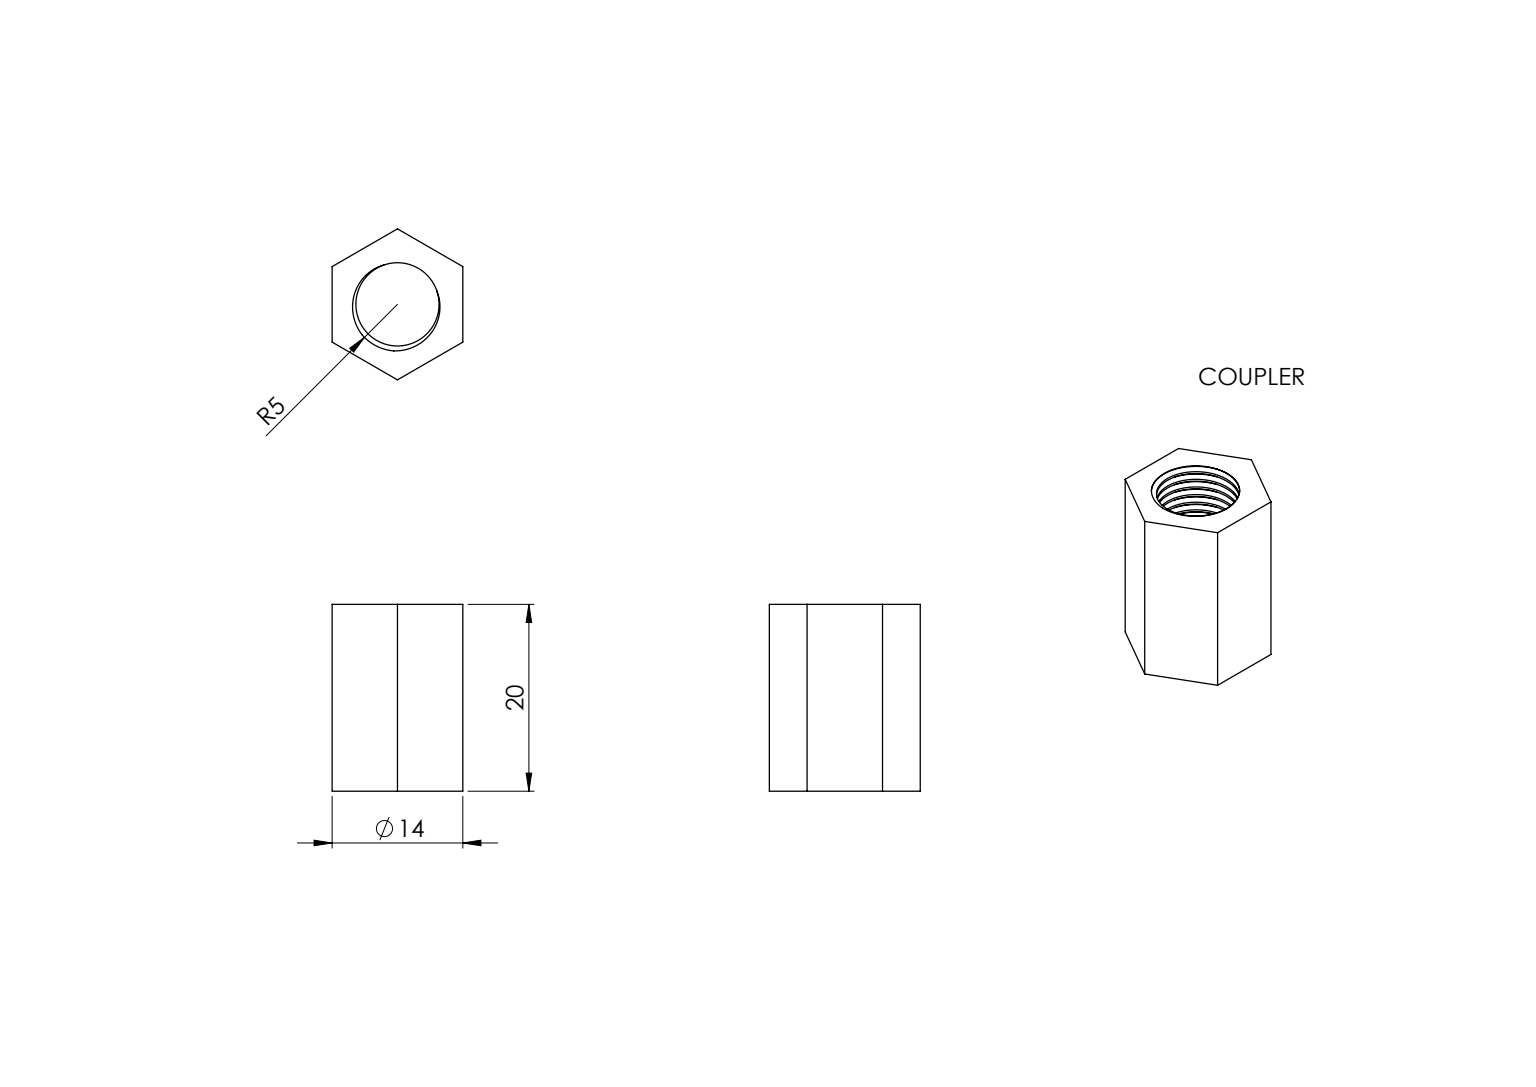
ISO-10303-21;
HEADER;
FILE_DESCRIPTION (('STEP AP214'),
    '1' );
FILE_NAME ('coupler.step',
    '2026-10-25T05:52:03',
    ( '' ),
    ( '' ),
    'SwSTEP 2.0',
    'SolidWorks 2026',
    '' );
FILE_SCHEMA (( 'AUTOMOTIVE_DESIGN' ));
ENDSEC;

DATA;
#3=CARTESIAN_POINT ( 'NONE',  ( -59.29741812935640155, -128.8750000013656063, -2.196230717870135685 ) ) ;
#16=CARTESIAN_POINT ( 'NONE',  ( -60.14911071818854538, -150.1875000027311842, 1.666127454062681368 ) ) ;
#81=CARTESIAN_POINT ( 'NONE',  ( -50.70258187064364108, -139.3750000013656063, 2.196230717870141014 ) ) ;
#85=ORIENTED_EDGE ( 'NONE', *, *, #22562, .F. ) ;
#86=ADVANCED_FACE ( 'NONE', ( #1332 ), #40849, .F. ) ;
#94=CARTESIAN_POINT ( 'NONE',  ( -54.60164318462004474, -140.3750000000000284, -4.984105922594373794 ) ) ;
#101=ADVANCED_FACE ( 'NONE', ( #35084 ), #10624, .T. ) ;
#104=ADVANCED_FACE ( 'NONE', ( #49860 ), #20614, .F. ) ;
#106=CARTESIAN_POINT ( 'NONE',  ( -58.39396692619412477, -139.4375000013656063, 2.891590998281057701 ) ) ;
#132=CARTESIAN_POINT ( 'NONE',  ( -51.60603307380591787, -145.1875000013656063, -2.891590998281053704 ) ) ;
#163=ORIENTED_EDGE ( 'NONE', *, *, #35025, .F. ) ;
#169=CARTESIAN_POINT ( 'NONE',  ( -50.18089887299979068, -133.6875000000000568, 2.462841084822635640 ) ) ;
#178=CARTESIAN_POINT ( 'NONE',  ( -60.14911071818854538, -125.1875000027312126, 1.666127454062681368 ) ) ;
#202=CARTESIAN_POINT ( 'NONE',  ( -53.51423613279429503, -126.2500000013656063, 4.591703134518082763 ) ) ;
#203=CARTESIAN_POINT ( 'NONE',  ( -52.10840900171896806, -147.1875000013656063, 3.393966926194110556 ) ) ;
#214=CARTESIAN_POINT ( 'NONE',  ( -55.35523342533222291, -125.5625000013655921, 4.444560631937231499 ) ) ;
#235=CARTESIAN_POINT ( 'NONE',  ( -59.44456063193725015, -149.8125000013656063, -0.3552334253322034230 ) ) ;
#246=CARTESIAN_POINT ( 'NONE',  ( -53.33387254593733928, -145.8125000000000284, 5.149110718188519620 ) ) ;
#253=ORIENTED_EDGE ( 'NONE', *, *, #51599, .T. ) ;
#254=CARTESIAN_POINT ( 'NONE',  ( -59.29741812935640155, -144.8750000013656063, -2.196230717870135685 ) ) ;
#255=CARTESIAN_POINT ( 'NONE',  ( -49.85088928181150436, -137.6875000027312126, -1.666127454062680702 ) ) ;
#267=CARTESIAN_POINT ( 'NONE',  ( -49.85088928181150436, -153.5625000000000284, -1.666127454062680480 ) ) ;
#268=CARTESIAN_POINT ( 'NONE',  ( -50.40829686548195099, -135.0000000013656347, -1.485763867205728284 ) ) ;
#283=CARTESIAN_POINT ( 'NONE',  ( -59.59170313451811296, -138.5000000013656347, 1.485763867205729394 ) ) ;
#314=CARTESIAN_POINT ( 'NONE',  ( -56.48576386720575471, -152.7500000013655779, -4.591703134518078322 ) ) ;
#321=CARTESIAN_POINT ( 'NONE',  ( -57.19623071787017210, -127.6250000013656205, 4.297418129356382899 ) ) ;
#331=CARTESIAN_POINT ( 'NONE',  ( -51.19402409849444524, -149.6250000027312126, -3.242614290531456334 ) ) ;
#360=CARTESIAN_POINT ( 'NONE',  ( -55.00000000000002132, -155.0000000000000284, 1.734723475976807094E-15 ) ) ;
#374=CARTESIAN_POINT ( 'NONE',  ( -59.77950423082105402, -135.0000000000000284, -0.4113032182319603658 ) ) ;
#389=EDGE_CURVE ( 'NONE', #14198, #16286, #4716, .T. ) ;
#399=CARTESIAN_POINT ( 'NONE',  ( -51.60603307380591787, -141.1875000013656063, -2.891590998281053704 ) ) ;
#402=EDGE_LOOP ( 'NONE', ( #47162, #48030, #33761, #57243 ) ) ;
#404=ORIENTED_EDGE ( 'NONE', *, *, #32775, .T. ) ;
#408=CYLINDRICAL_SURFACE ( 'NONE', #17648, 5.000000000000000000 ) ;
#418=CARTESIAN_POINT ( 'NONE',  ( -52.10840900171896806, -139.1875000013656347, 3.393966926194110556 ) ) ;
#441=CARTESIAN_POINT ( 'NONE',  ( -52.10840900171896806, -143.4375000013656063, 3.393966926194110556 ) ) ;
#470=CARTESIAN_POINT ( 'NONE',  ( -60.14911071818854538, -151.0625000000000284, 1.666127454062681146 ) ) ;
#485=CARTESIAN_POINT ( 'NONE',  ( -49.85088928181150436, -130.5625000000000568, -1.666127454062680702 ) ) ;
#491=ORIENTED_EDGE ( 'NONE', *, *, #46738, .F. ) ;
#493=CARTESIAN_POINT ( 'NONE',  ( -51.60603307380591787, -152.9375000013656063, -2.891590998281053704 ) ) ;
#515=CIRCLE ( 'NONE', #57003, 5.000000000000000000 ) ;
#516=CARTESIAN_POINT ( 'NONE',  ( -50.70258187064364108, -154.3750000013656063, 2.196230717870141014 ) ) ;
#517=CARTESIAN_POINT ( 'NONE',  ( -54.64476657466781973, -145.8125000013656063, -4.444560631937228834 ) ) ;
#518=EDGE_CURVE ( 'NONE', #43968, #24595, #43685, .T. ) ;
#542=EDGE_CURVE ( 'NONE', #41301, #34010, #1942, .T. ) ;
#546=DIRECTION ( 'NONE',  ( 0.000000000000000000, -1.000000000000000000, 0.000000000000000000 ) ) ;
#552=CARTESIAN_POINT ( 'NONE',  ( -52.10840900171896806, -146.4375000013656063, 3.393966926194110556 ) ) ;
#562=CARTESIAN_POINT ( 'NONE',  ( -52.53715891517739323, -147.4375000000000284, -4.819101127000233298 ) ) ;
#571=CARTESIAN_POINT ( 'NONE',  ( -59.59170313451810586, -144.7500000013655779, 1.485763867205729394 ) ) ;
#573=CARTESIAN_POINT ( 'NONE',  ( -51.75738570946856498, -134.8750000027312126, 3.805975901505576964 ) ) ;
#585=CARTESIAN_POINT ( 'NONE',  ( -52.80376928212989185, -132.8750000013656063, -4.297418129356379346 ) ) ;
#600=CARTESIAN_POINT ( 'NONE',  ( -59.44456063193725015, -138.5625000013656063, -0.3552334253322034230 ) ) ;
#610=CARTESIAN_POINT ( 'NONE',  ( -55.35523342533222291, -133.5625000013656063, 4.444560631937231499 ) ) ;
#633=CARTESIAN_POINT ( 'NONE',  ( -59.44456063193725015, -151.5625000013656063, -0.3552334253322034230 ) ) ;
#641=CARTESIAN_POINT ( 'NONE',  ( -52.80376928212989185, -129.1250000013655779, -4.297418129356379346 ) ) ;
#644=CARTESIAN_POINT ( 'NONE',  ( -50.01589407740564042, -136.7500000027312126, 0.3983568153799778022 ) ) ;
#651=CARTESIAN_POINT ( 'NONE',  ( -50.01589407740564042, -150.7500000027312410, 0.3983568153799778022 ) ) ;
#655=ORIENTED_EDGE ( 'NONE', *, *, #11941, .T. ) ;
#656=AXIS2_PLACEMENT_3D ( 'NONE', #10891, #51098, #35667 ) ;
#672=CARTESIAN_POINT ( 'NONE',  ( -54.64476657466781973, -150.8125000013656063, -4.444560631937228834 ) ) ;
#674=CARTESIAN_POINT ( 'NONE',  ( -50.01589407740564042, -148.6250000000000284, 0.3983568153799778022 ) ) ;
#697=VECTOR ( 'NONE', #14487, 1000.000000000000114 ) ;
#717=CARTESIAN_POINT ( 'NONE',  ( -55.35523342533222291, -139.5625000013656063, 4.444560631937231499 ) ) ;
#728=CARTESIAN_POINT ( 'NONE',  ( -52.53715891517739323, -140.4375000000000000, -4.819101127000233298 ) ) ;
#738=CARTESIAN_POINT ( 'NONE',  ( -50.40829686548195099, -141.0000000013656063, -1.485763867205728284 ) ) ;
#764=CARTESIAN_POINT ( 'NONE',  ( -49.85088928181150436, -154.5625000000000000, -1.666127454062680480 ) ) ;
#768=CARTESIAN_POINT ( 'NONE',  ( -55.35523342533222291, -143.5625000013656063, 4.444560631937231499 ) ) ;
#769=CARTESIAN_POINT ( 'NONE',  ( -55.00000000000002132, -155.0000000000000284, 1.734723475976807094E-15 ) ) ;
#774=CARTESIAN_POINT ( 'NONE',  ( -58.24261429053147765, -136.2500000000000284, -3.805975901505573855 ) ) ;
#782=CARTESIAN_POINT ( 'NONE',  ( -54.60164318462004474, -138.5000000027312126, -4.984105922594373794 ) ) ;
#804=CARTESIAN_POINT ( 'NONE',  ( -56.66612745406293783, -141.3125000000000000, -5.149110718188535607 ) ) ;
#809=CARTESIAN_POINT ( 'NONE',  ( -58.80597590150559739, -130.0000000000000284, 3.242614290531460330 ) ) ;
#819=CARTESIAN_POINT ( 'NONE',  ( -57.19623071787017210, -154.3750000013656063, 4.297418129356382899 ) ) ;
#822=DIRECTION ( 'NONE',  ( 0.000000000000000000, -1.000000000000000000, 0.000000000000000000 ) ) ;
#848=CARTESIAN_POINT ( 'NONE',  ( -56.48576386720575471, -124.7500000013655921, -4.591703134518078322 ) ) ;
#849=CARTESIAN_POINT ( 'NONE',  ( -55.35523342533222291, -142.3125000013656063, 4.444560631937231499 ) ) ;
#877=ORIENTED_EDGE ( 'NONE', *, *, #37498, .T. ) ;
#888=CARTESIAN_POINT ( 'NONE',  ( -51.75738570946856498, -139.7500000000000000, 3.805975901505576964 ) ) ;
#898=CARTESIAN_POINT ( 'NONE',  ( -59.59170313451810586, -146.7500000013656063, 1.485763867205729394 ) ) ;
#900=CARTESIAN_POINT ( 'NONE',  ( -60.14911071818854538, -134.1875000027312410, 1.666127454062681368 ) ) ;
#916=CARTESIAN_POINT ( 'NONE',  ( -52.80376928212989185, -128.8750000013656063, -4.297418129356379346 ) ) ;
#933=( BOUNDED_CURVE ( )  B_SPLINE_CURVE ( 2, ( #61186, #36731, #45181, #61505, #52157, #37669, #30381, #11955, #12285 ),
 .UNSPECIFIED., .F., .F. ) 
 B_SPLINE_CURVE_WITH_KNOTS ( ( 3, 2, 2, 2, 3 ),
 ( 0.2250000000000001998, 0.2291666666666668517, 0.2333333333333335313, 0.2375000000000001832, 0.2416666666666668628 ),
 .UNSPECIFIED. ) 
 CURVE ( )  GEOMETRIC_REPRESENTATION_ITEM ( )  RATIONAL_B_SPLINE_CURVE ( ( 0.9999999999999964473, 0.9238795325112902912, 1.000000000000000000, 0.9238795325112867385, 1.000000000000000000, 0.9238795325112867385, 1.000000000000000000, 0.9238795325112831858, 1.000000000000003553 ) ) 
 REPRESENTATION_ITEM ( '' )  );
#934=CARTESIAN_POINT ( 'NONE',  ( -52.80376928212989185, -138.8750000013655779, -4.297418129356379346 ) ) ;
#945=CARTESIAN_POINT ( 'NONE',  ( -52.80376928212989185, -130.1250000013656347, -4.297418129356379346 ) ) ;
#970=CARTESIAN_POINT ( 'NONE',  ( -59.59170313451810586, -151.5000000013655779, 1.485763867205729394 ) ) ;
#977=CARTESIAN_POINT ( 'NONE',  ( -50.01589407740564042, -154.6250000000000284, 0.3983568153799778022 ) ) ;
#988=CARTESIAN_POINT ( 'NONE',  ( -50.18089887299979068, -145.8125000027311842, 2.462841084822635640 ) ) ;
#1004=CARTESIAN_POINT ( 'NONE',  ( -56.66612745406288099, -143.3125000000000000, -5.149110718188529390 ) ) ;
#1006=CARTESIAN_POINT ( 'NONE',  ( -57.89159099828107458, -149.6875000013656063, -3.393966926194107447 ) ) ;
#1025=CARTESIAN_POINT ( 'NONE',  ( -51.75738570946856498, -140.7500000000000000, 3.805975901505576964 ) ) ;
#1037=CARTESIAN_POINT ( 'NONE',  ( -51.19402409849444524, -147.6250000027312126, -3.242614290531456334 ) ) ;
#1052=CARTESIAN_POINT ( 'NONE',  ( -51.60603307380591787, -134.1875000013656063, -2.891590998281053704 ) ) ;
#1058=CARTESIAN_POINT ( 'NONE',  ( -55.00000000000002132, -155.0000000000000284, 1.734723475976807094E-15 ) ) ;
#1068=CARTESIAN_POINT ( 'NONE',  ( -53.51423613279429503, -140.2500000013656063, 4.591703134518082763 ) ) ;
#1073=ORIENTED_EDGE ( 'NONE', *, *, #41605, .F. ) ;
#1090=CARTESIAN_POINT ( 'NONE',  ( -56.66612745406272467, -154.3125000000000284, -5.149110718188517843 ) ) ;
#1093=CARTESIAN_POINT ( 'NONE',  ( -50.55543936806279248, -145.3125000013656063, 0.3552334253322060320 ) ) ;
#1138=CARTESIAN_POINT ( 'NONE',  ( -50.01589407740564042, -128.6250000000000284, 0.3983568153799778022 ) ) ;
#1145=CARTESIAN_POINT ( 'NONE',  ( -52.53715891517739323, -124.5625000027312268, -4.819101127000233298 ) ) ;
#1167=VECTOR ( 'NONE', #55223, 1000.000000000000000 ) ;
#1170=CARTESIAN_POINT ( 'NONE',  ( -55.35523342533222291, -126.3125000013655921, 4.444560631937231499 ) ) ;
#1171=CARTESIAN_POINT ( 'NONE',  ( -55.35523342533222291, -141.3125000013656063, 4.444560631937231499 ) ) ;
#1213=CARTESIAN_POINT ( 'NONE',  ( -58.24261429053147765, -140.2500000000000000, -3.805975901505573855 ) ) ;
#1216=ORIENTED_EDGE ( 'NONE', *, *, #46137, .T. ) ;
#1223=CARTESIAN_POINT ( 'NONE',  ( -57.89159099828107458, -144.9375000013656063, -3.393966926194107447 ) ) ;
#1225=CARTESIAN_POINT ( 'NONE',  ( -53.33387254593733928, -132.9375000027312126, 5.149110718188519620 ) ) ;
#1237=CARTESIAN_POINT ( 'NONE',  ( -50.40829686548195099, -129.0000000013656063, -1.485763867205728284 ) ) ;
#1251=CARTESIAN_POINT ( 'NONE',  ( -53.51423613279429503, -138.2500000013656063, 4.591703134518082763 ) ) ;
#1260=CARTESIAN_POINT ( 'NONE',  ( -58.39396692619412477, -133.6875000013656063, 2.891590998281057701 ) ) ;
#1289=CARTESIAN_POINT ( 'NONE',  ( -54.64476657466781973, -149.8125000013656063, -4.444560631937228834 ) ) ;
#1296=EDGE_CURVE ( 'NONE', #19989, #11458, #56971, .T. ) ;
#1299=CARTESIAN_POINT ( 'NONE',  ( -58.24261429053147765, -154.2500000000000284, -3.805975901505573855 ) ) ;
#1309=CARTESIAN_POINT ( 'NONE',  ( -56.66612745406270335, -145.4375000027312694, -5.149110718188516067 ) ) ;
#1325=CARTESIAN_POINT ( 'NONE',  ( -51.60603307380591787, -148.9375000013656063, -2.891590998281053704 ) ) ;
#1332=FACE_OUTER_BOUND ( 'NONE', #402, .T. ) ;
#1364=CARTESIAN_POINT ( 'NONE',  ( -57.46284108482265651, -141.0625000027312410, 4.819101127000238627 ) ) ;
#1372=CARTESIAN_POINT ( 'NONE',  ( -59.59170313451811296, -135.7500000013656063, 1.485763867205729394 ) ) ;
#1388=CARTESIAN_POINT ( 'NONE',  ( -57.89159099828107458, -140.6875000013656063, -3.393966926194107447 ) ) ;
#1389=CARTESIAN_POINT ( 'NONE',  ( -51.75738570946856498, -154.7500000000000284, 3.805975901505576964 ) ) ;
#1413=CARTESIAN_POINT ( 'NONE',  ( -51.60603307380591787, -141.1875000013656063, -2.891590998281053704 ) ) ;
#1423=VERTEX_POINT ( 'NONE', #56144 ) ;
#1432=CARTESIAN_POINT ( 'NONE',  ( -58.24261429053147765, -151.3750000027312126, -3.805975901505573855 ) ) ;
#1444=AXIS2_PLACEMENT_3D ( 'NONE', #10621, #50516, #34419 ) ;
#1446=CARTESIAN_POINT ( 'NONE',  ( -54.60164318462004474, -137.3750000000000284, -4.984105922594373794 ) ) ;
#1453=CARTESIAN_POINT ( 'NONE',  ( -51.19402409849444524, -129.5000000000000284, -3.242614290531456334 ) ) ;
#1457=VECTOR ( 'NONE', #822, 1000.000000000000000 ) ;
#1461=CARTESIAN_POINT ( 'NONE',  ( -50.55543936806279248, -151.0625000013656063, 0.3552334253322060320 ) ) ;
#1467=EDGE_CURVE ( 'NONE', #46511, #2425, #9232, .T. ) ;
#1484=CARTESIAN_POINT ( 'NONE',  ( -59.29741812935640155, -127.6250000013656205, -2.196230717870135685 ) ) ;
#1485=CARTESIAN_POINT ( 'NONE',  ( -50.55543936806279248, -141.0625000013656063, 0.3552334253322060320 ) ) ;
#1488=CARTESIAN_POINT ( 'NONE',  ( -50.18089887299979068, -153.8125000027311842, 2.462841084822631199 ) ) ;
#1521=CARTESIAN_POINT ( 'NONE',  ( -55.39835681537999790, -141.8750000000000284, 4.984105922594378235 ) ) ;
#1530=CARTESIAN_POINT ( 'NONE',  ( -57.89159099828107458, -140.9375000013656063, -3.393966926194107447 ) ) ;
#1532=CARTESIAN_POINT ( 'NONE',  ( -50.01589407740564042, -133.7500000027312126, 0.3983568153799778022 ) ) ;
#1547=CARTESIAN_POINT ( 'NONE',  ( -55.35523342533222291, -128.3125000013656063, 4.444560631937231499 ) ) ;
#1562=CARTESIAN_POINT ( 'NONE',  ( -50.40829686548195099, -138.0000000013656063, -1.485763867205728284 ) ) ;
#1571=ORIENTED_EDGE ( 'NONE', *, *, #11677, .F. ) ;
#1573=CARTESIAN_POINT ( 'NONE',  ( -52.10840900171896806, -132.4375000013656063, 3.393966926194110556 ) ) ;
#1607=CARTESIAN_POINT ( 'NONE',  ( -56.48576386720575471, -125.0000000013656205, -4.591703134518078322 ) ) ;
#1617=CARTESIAN_POINT ( 'NONE',  ( -58.24261429053147765, -145.3750000027312126, -3.805975901505573855 ) ) ;
#1630=ORIENTED_EDGE ( 'NONE', *, *, #7870, .T. ) ;
#1637=CARTESIAN_POINT ( 'NONE',  ( -58.39396692619412477, -149.4375000013656063, 2.891590998281057701 ) ) ;
#1666=CARTESIAN_POINT ( 'NONE',  ( -50.01589407740564042, -147.7500000027312126, 0.3983568153799778022 ) ) ;
#1680=CARTESIAN_POINT ( 'NONE',  ( -57.19623071787017210, -133.6250000013655779, 4.297418129356382899 ) ) ;
#1688=CARTESIAN_POINT ( 'NONE',  ( -50.84841373685102184, -135.0000000000001137, -1.652645393539816210 ) ) ;
#1689=ORIENTED_EDGE ( 'NONE', *, *, #14237, .T. ) ;
#1717=AXIS2_PLACEMENT_3D ( 'NONE', #19426, #24252, #13966 ) ;
#1726=CARTESIAN_POINT ( 'NONE',  ( -50.40829686548195099, -141.2500000013656347, -1.485763867205728284 ) ) ;
#1728=EDGE_CURVE ( 'NONE', #35208, #29222, #34787, .T. ) ;
#1743=CARTESIAN_POINT ( 'NONE',  ( -50.18089887299976937, -138.8125000027312126, 2.462841084822397164 ) ) ;
#1748=CARTESIAN_POINT ( 'NONE',  ( -59.44456063193725015, -136.8125000013656063, -0.3552334253322034230 ) ) ;
#1760=CARTESIAN_POINT ( 'NONE',  ( -53.51423613279429503, -148.5000000013655779, 4.591703134518082763 ) ) ;
#1764=ORIENTED_EDGE ( 'NONE', *, *, #58262, .F. ) ;
#1772=CARTESIAN_POINT ( 'NONE',  ( -59.81910112700025905, -131.1875000000000568, -2.462841084822630311 ) ) ;
#1778=AXIS2_PLACEMENT_3D ( 'NONE', #35397, #61762, #7412 ) ;
#1781=CARTESIAN_POINT ( 'NONE',  ( -50.55543936806279248, -153.0625000013656063, 0.3552334253322060320 ) ) ;
#1782=CARTESIAN_POINT ( 'NONE',  ( -57.46284108482265651, -150.0625000027312126, 4.819101127000238627 ) ) ;
#1784=( BOUNDED_SURFACE ( )  B_SPLINE_SURFACE ( 1, 2, ( 
 ( #18999, #28654, #39246, #49226, #52797, #4527, #19635, #4227, #38932, #38612, #58248, #34108, #8733, #23841, #14174, #33800, #62771, #58873, #14803, #39563, #34417, #47958, #29595, #33489, #63399, #54046, #9983, #5167, #53418, #24785, #59204, #18691, #15132, #28341, #3913, #58567, #9351, #43131, #28963, #38317, #57945, #13865, #43444, #24152, #55013, #35392, #15775, #49544, #40843, #39883, #5484, #45996, #41159, #45039, #25745, #25420, #25099, #20923, #672, #10937, #60804, #16415, #55345, #35715, #50513, #45678, #26063, #36033, #11259, #54380, #6765, #30883, #55665, #6454, #11578, #1961, #1006, #34754, #20281, #30555, #1637, #21237, #50180, #6132, #60487, #31198, #44709, #50827, #1325, #40528, #26378, #45360, #35078, #54698, #21562, #10305, #29918, #59528, #60170, #20610, #30231, #15461, #16091, #10619, #49855, #5803, #40215, #59850, #11891, #21879, #61442, #22198, #12851, #31838, #32147, #7724, #27017, #46635, #2906, #55978, #17368, #51469, #16731, #36991, #32470, #37611, #42745, #36347, #42114, #41798, #22521, #27645, #52099, #12534, #51782, #2581, #27329, #46959, #61758, #17686, #52422, #8039, #31509, #37301, #17050, #56930, #56618, #47272, #3218, #22838, #42429, #51154, #62071, #26701, #2275, #36666, #7087, #41475, #27954, #17985, #57252, #13168, #8354, #46318, #32792, #47576, #3528, #23137, #61125, #56293, #12223, #7408, #14734, #53347, #43065, #43998, #24715, #53035, #43375, #62703, #33108, #18628, #18928, #19565, #8973, #62388, #9597, #19244, #52722, #29518, #38860, #58496, #9910, #9282, #14420, #38251, #57566, #63646, #34042, #53663, #63021, #8656, #48830, #18309, #28269, #28897, #24395, #29204, #24086, #13492, #4458, #4770, #13794, #14104, #48518, #28583, #48204, #43681, #37934, #38542, #33416, #47884, #58174, #39177, #58802, #3842, #23462, #63325, #23774, #34351, #53980, #49150, #33729, #5096, #4157, #57872, #15703, #35321, #50108, #16342, #35644, #59131, #30485, #44641, #6063, #20538, #25676, #5734, #25350, #934, #19882, #10868, #54298, #29843, #600, #283, #5414, #55590, #10549, #1251, #44970, #35964, #39495, #1562, #40135, #11509, #31125, #55270, #54942, #45285, #20852, #60417, #40456, #25031, #25988, #6692, #35009, #59777, #20210, #15066, #39812, #60096, #21164, #54624, #44319, #11188, #16017, #34679, #50748, #30811, #50441, #10238, #6382, #45605, #59454, #49476, #40771, #15385, #30159, #49788, #16654, #12772, #45921, #60732, #56540, #52019, #2823, #51708, #41086, #32071, #61364, #32394, #61679, #36279, #22442, #12460, #7649, #27562, #2504, #26622, #46241, #42039, #17612, #37228, #56854, #22122, #16974, #21807, #1884, #27252, #46879, #26297, #31433, #7963, #36585, #21488, #51073, #7336, #31761, #47195, #3138, #55903, #7014, #22757, #56220, #11814, #2203, #26947, #51394, #42355, #41402, #41714, #17286, #12140, #46564, #61994, #61053, #36909, #17914, #37535, #57175, #13092, #32712, #52340, #8274, #33653, #33338, #58093, #19158, #23999, #4077, #23700, #57795, #62933, #43297, #18847, #14024, #43915, #63245, #23064, #53271, #8579, #9206, #48126, #28819, #52955, #8893, #28508, #47497, #38467, #18231, #57490, #28191, #27878, #33030, #19483, #38173, #48440, #4380, #63563, #3450, #29122, #43601, #39096, #58725, #38777, #58416, #14343, #33964, #24309, #53585, #52646, #9515, #34270, #62629, #48745, #47806, #42669, #3763, #4687, #14651, #18551, #62308, #37857, #13409, #23387, #42986, #13715, #50027, #1484, #44887, #5985, #10153, #49065, #55186, #25590, #45203, #54543, #44238, #40375, #9821, #24631, #20450, #15939, #30404, #15625, #5011, #59694, #25266, #60016, #1170, #202, #20770, #40050, #35242, #11106, #30078, #54215, #29758, #35562, #30731, #50353, #6300, #49709, #44559, #49392, #29431, #10466, #25905, #19800, #45523, #5654, #21087, #40691, #60336, #848, #54861, #10792, #16264, #53896, #34583 ),
 ( #39408, #59047, #14975, #5336, #24953, #516, #20127, #39727, #59366, #15299, #34922, #36509, #26223, #22363, #55512, #6610, #2430, #61604, #12387, #61286, #50669, #41633, #7258, #41963, #7568, #45843, #32001, #22041, #17208, #37158, #12060, #36199, #55820, #51635, #27181, #46797, #2743, #31685, #26546, #31354, #11426, #36835, #56465, #35882, #41012, #17539, #46166, #31044, #60655, #16892, #41325, #56782, #50995, #51320, #26871, #2128, #21729, #12701, #1805, #56140, #6934, #21409, #46483, #32314, #51945, #61922, #16579, #7885, #60972, #27488, #47118, #3066, #22683, #42283, #11736, #8822, #52887, #28437, #23625, #53509, #9133, #32634, #4003, #18153, #43221, #57722, #37465, #32954, #62556, #52263, #23928, #22997, #8201, #29049, #24238, #28120, #48050, #8510, #27804, #9439, #28739, #62861, #18774, #38401, #33889, #58024, #62236, #63174, #43842, #47737, #18476, #37782, #47429, #57413, #38097, #38704, #3694, #17842, #48366, #13953, #3380, #48673, #33579, #53199, #4613, #4309, #43529, #13333, #13015, #19085, #58341, #14270, #13648, #42599, #57095, #52578, #23307, #42907, #33268, #39976, #25189, #14574, #5575, #34850, #5903, #35173, #9750, #59621, #30008, #49638, #1093, #39653, #132, #19726, #15553, #54789, #10719, #30326, #59290, #54136, #58968, #39026, #44805, #20375, #63488, #4937, #45129, #10075, #58654, #24560, #44482, #5260, #49950, #14896, #15221, #54471, #29687, #49317, #768, #34197, #441, #34504, #19412, #20048, #25510, #20702, #25833, #53821, #40306, #24881, #59944, #15867, #35488, #10398, #55107, #11029, #30653, #50276, #6221, #29357, #48990, #44164, #39335, #31609, #45769, #40931, #16814, #26788, #60579, #26471, #2046, #21013, #11981, #55432, #30971, #1726, #1413, #6536, #56704, #11660, #2356, #46086, #17462, #40620, #2664, #21652, #12622, #36434, #36122, #60264, #51244, #11349, #41244, #51866, #27104, #21964, #46407, #61210, #56388, #36759, #46719, #41559, #16182, #37084, #17136, #22285, #12315, #41884, #32235, #55744, #7809, #50596, #60891, #31927, #51555, #56064, #61530, #7491, #21331, #50914, #45449, #35807, #26150, #16500, #31280, #7180, #6857, #62478, #61849, #47664, #28354, #13880, #27411, #3616, #23855, #42205, #4240, #47356, #47974, #18076, #63103, #43458, #57650, #33508, #2991, #19015, #38628, #22927, #52181, #53435, #3928, #43146, #58270, #37385, #33815, #22609, #14190, #47042, #23223, #42836, #17768, #57338, #27729, #53124, #57019, #12934, #18398, #62786, #3305, #13578, #13254, #32878, #8749, #32558, #42519, #37697, #52506, #8126, #23546, #57959, #62156, #38330, #8440, #28044, #38019, #33196, #9058, #28668, #48285, #52811, #18705, #25999, #20219, #45617, #30822, #50453, #1260, #10879, #610, #15712, #11519, #1894, #36289, #30496, #21500, #28979, #25360, #54950, #24167, #16353, #15394, #43770, #41096, #16666, #20547, #6073, #1573, #10556, #40466, #40144, #35330, #55281, #48601, #5741, #59789, #50117, #39820, #6393, #40781, #60743, #21173, #4541, #50759, #54632, #20863, #60427, #35974, #55601, #25686, #31134, #6703, #59462, #26309, #45931, #9366, #60106, #45295, #35019, #16027, #30167, #49797, #44979, #35654, #945, #11200, #7345, #36921, #7024, #62004, #61064, #26633, #3461, #62319, #2515, #46890, #46574, #46253, #42048, #21816, #32081, #18244, #37545, #12782, #56864, #7974, #3149, #47206, #57185, #32404, #11824, #27888, #52031, #13104, #27572, #32722, #23074, #22131, #55912, #41413, #56550, #22769, #42365, #51718, #8284, #17923, #56231, #61374, #52350, #47510, #42678, #31443, #51086, #12471, #2213, #27264, #16984, #7659, #36596, #12152, #31771, #2833, #51403, #26956, #41725, #17295, #22451, #61691, #17622, #37239, #4391, #43928, #13418, #9833, #34283, #33351, #62641, #214, #14354, #53597, #29445, #47816, #44250, #33041, #53907, #49077, #33663, #53281, #5024, #4089, #38184, #24322 ) ),
 .UNSPECIFIED., .F., .F., .F. ) 
 B_SPLINE_SURFACE_WITH_KNOTS ( ( 2, 2 ),
 ( 3, 2, 2, 2, 2, 2, 2, 2, 2, 2, 2, 2, 2, 2, 2, 2, 2, 2, 2, 2, 2, 2, 2, 2, 2, 2, 2, 2, 2, 2, 2, 2, 2, 2, 2, 2, 2, 2, 2, 2, 2, 2, 2, 2, 2, 2, 2, 2, 2, 2, 2, 2, 2, 2, 2, 2, 2, 2, 2, 2, 2, 2, 2, 2, 2, 2, 2, 2, 2, 2, 2, 2, 2, 2, 2, 2, 2, 2, 2, 2, 2, 2, 2, 2, 2, 2, 2, 2, 2, 2, 2, 2, 2, 2, 2, 2, 2, 2, 2, 2, 2, 2, 2, 2, 2, 2, 2, 2, 2, 2, 2, 2, 2, 2, 2, 2, 2, 2, 2, 2, 2, 2, 2, 2, 2, 2, 2, 2, 2, 2, 2, 2, 2, 2, 2, 2, 2, 2, 2, 2, 2, 2, 2, 2, 2, 2, 2, 2, 2, 2, 2, 2, 2, 2, 2, 2, 2, 2, 2, 2, 2, 2, 2, 2, 2, 2, 2, 2, 2, 2, 2, 2, 2, 2, 2, 2, 2, 2, 2, 2, 2, 2, 2, 2, 2, 2, 2, 2, 2, 2, 2, 2, 2, 2, 2, 2, 2, 2, 2, 2, 2, 2, 2, 2, 2, 2, 2, 2, 2, 2, 2, 2, 2, 2, 2, 2, 2, 2, 2, 2, 2, 2, 2, 2, 2, 2, 2, 2, 2, 2, 2, 2, 2, 2, 2, 2, 2, 2, 2, 2, 3 ),
 ( 0.000000000000000000, 1.000000000000000000 ),
 ( 0.000000000000000000, 0.004166666666666666609, 0.008333333333333333218, 0.01250000000000000069, 0.01666666666666666644, 0.02083333333333333218, 0.02500000000000000139, 0.02916666666666666713, 0.03333333333333333287, 0.03749999999999999861, 0.04166666666666666435, 0.04583333333333333010, 0.05000000000000000278, 0.05416666666666666852, 0.05833333333333333426, 0.06250000000000000000, 0.06666666666666666574, 0.07083333333333333148, 0.07499999999999999722, 0.07916666666666666297, 0.08333333333333332871, 0.08749999999999999445, 0.09166666666666666019, 0.09583333333333333981, 0.1000000000000000056, 0.1041666666666666713, 0.1083333333333333370, 0.1125000000000000028, 0.1166666666666666685, 0.1208333333333333343, 0.1250000000000000000, 0.1291666666666666796, 0.1333333333333333315, 0.1375000000000000111, 0.1416666666666666630, 0.1458333333333333426, 0.1499999999999999944, 0.1541666666666666741, 0.1583333333333333259, 0.1625000000000000056, 0.1666666666666666574, 0.1708333333333333370, 0.1749999999999999889, 0.1791666666666666685, 0.1833333333333333204, 0.1875000000000000000, 0.1916666666666666796, 0.1958333333333333315, 0.2000000000000000111, 0.2041666666666666630, 0.2083333333333333426, 0.2124999999999999944, 0.2166666666666666741, 0.2208333333333333259, 0.2250000000000000056, 0.2291666666666666574, 0.2333333333333333370, 0.2374999999999999889, 0.2416666666666666685, 0.2458333333333333204, 0.2500000000000000000, 0.2541666666666666519, 0.2583333333333333592, 0.2625000000000000111, 0.2666666666666666630, 0.2708333333333333148, 0.2750000000000000222, 0.2791666666666666741, 0.2833333333333333259, 0.2874999999999999778, 0.2916666666666666852, 0.2958333333333333370, 0.2999999999999999889, 0.3041666666666666408, 0.3083333333333333481, 0.3125000000000000000, 0.3166666666666666519, 0.3208333333333333592, 0.3250000000000000111, 0.3291666666666666630, 0.3333333333333333148, 0.3375000000000000222, 0.3416666666666666741, 0.3458333333333333259, 0.3499999999999999778, 0.3541666666666666852, 0.3583333333333333370, 0.3624999999999999889, 0.3666666666666666408, 0.3708333333333333481, 0.3750000000000000000, 0.3791666666666666519, 0.3833333333333333592, 0.3875000000000000111, 0.3916666666666666630, 0.3958333333333333148, 0.4000000000000000222, 0.4041666666666666741, 0.4083333333333333259, 0.4124999999999999778, 0.4166666666666666852, 0.4208333333333333370, 0.4249999999999999889, 0.4291666666666666408, 0.4333333333333333481, 0.4375000000000000000, 0.4416666666666666519, 0.4458333333333333592, 0.4500000000000000111, 0.4541666666666666630, 0.4583333333333333148, 0.4625000000000000222, 0.4666666666666666741, 0.4708333333333333259, 0.4749999999999999778, 0.4791666666666666852, 0.4833333333333333370, 0.4874999999999999889, 0.4916666666666666408, 0.4958333333333333481, 0.5000000000000000000, 0.5041666666666666519, 0.5083333333333333037, 0.5124999999999999556, 0.5166666666666667185, 0.5208333333333333703, 0.5250000000000000222, 0.5291666666666666741, 0.5333333333333333259, 0.5374999999999999778, 0.5416666666666666297, 0.5458333333333332815, 0.5500000000000000444, 0.5541666666666666963, 0.5583333333333333481, 0.5625000000000000000, 0.5666666666666666519, 0.5708333333333333037, 0.5749999999999999556, 0.5791666666666667185, 0.5833333333333333703, 0.5875000000000000222, 0.5916666666666666741, 0.5958333333333333259, 0.5999999999999999778, 0.6041666666666666297, 0.6083333333333332815, 0.6125000000000000444, 0.6166666666666666963, 0.6208333333333333481, 0.6250000000000000000, 0.6291666666666666519, 0.6333333333333333037, 0.6374999999999999556, 0.6416666666666667185, 0.6458333333333333703, 0.6500000000000000222, 0.6541666666666666741, 0.6583333333333333259, 0.6624999999999999778, 0.6666666666666666297, 0.6708333333333332815, 0.6750000000000000444, 0.6791666666666666963, 0.6833333333333333481, 0.6875000000000000000, 0.6916666666666666519, 0.6958333333333333037, 0.6999999999999999556, 0.7041666666666667185, 0.7083333333333333703, 0.7125000000000000222, 0.7166666666666666741, 0.7208333333333333259, 0.7249999999999999778, 0.7291666666666666297, 0.7333333333333332815, 0.7375000000000000444, 0.7416666666666666963, 0.7458333333333333481, 0.7500000000000000000, 0.7541666666666666519, 0.7583333333333333037, 0.7624999999999999556, 0.7666666666666667185, 0.7708333333333333703, 0.7750000000000000222, 0.7791666666666666741, 0.7833333333333333259, 0.7874999999999999778, 0.7916666666666666297, 0.7958333333333332815, 0.8000000000000000444, 0.8041666666666666963, 0.8083333333333333481, 0.8125000000000000000, 0.8166666666666666519, 0.8208333333333333037, 0.8249999999999999556, 0.8291666666666667185, 0.8333333333333333703, 0.8375000000000000222, 0.8416666666666666741, 0.8458333333333333259, 0.8499999999999999778, 0.8541666666666666297, 0.8583333333333332815, 0.8625000000000000444, 0.8666666666666666963, 0.8708333333333333481, 0.8750000000000000000, 0.8791666666666666519, 0.8833333333333333037, 0.8874999999999999556, 0.8916666666666667185, 0.8958333333333333703, 0.9000000000000000222, 0.9041666666666666741, 0.9083333333333333259, 0.9124999999999999778, 0.9166666666666666297, 0.9208333333333332815, 0.9250000000000000444, 0.9291666666666666963, 0.9333333333333333481, 0.9375000000000000000, 0.9416666666666666519, 0.9458333333333333037, 0.9499999999999999556, 0.9541666666666667185, 0.9583333333333333703, 0.9625000000000000222, 0.9666666666666666741, 0.9708333333333333259, 0.9749999999999999778, 0.9791666666666666297, 0.9833333333333332815, 0.9875000000000000444, 0.9916666666666666963, 0.9958333333333333481, 1.000000000000000000 ),
 .UNSPECIFIED. ) 
 GEOMETRIC_REPRESENTATION_ITEM ( )  RATIONAL_B_SPLINE_SURFACE ( (
 ( 1.000000000000000000, 0.9238795325112867385, 1.000000000000000000, 0.9238795325112867385, 1.000000000000000000, 0.9238795325112867385, 1.000000000000000000, 0.9238795325112867385, 1.000000000000000000, 0.9238795325112867385, 1.000000000000000000, 0.9238795325112867385, 1.000000000000000000, 0.9238795325112867385, 1.000000000000000000, 0.9238795325112867385, 1.000000000000000000, 0.9238795325112867385, 1.000000000000000000, 0.9238795325112867385, 1.000000000000000000, 0.9238795325112867385, 1.000000000000000000, 0.9238795325112867385, 1.000000000000000000, 0.9238795325112867385, 1.000000000000000000, 0.9238795325112867385, 1.000000000000000000, 0.9238795325112867385, 1.000000000000000000, 0.9238795325112867385, 1.000000000000000000, 0.9238795325112867385, 1.000000000000000000, 0.9238795325112867385, 1.000000000000000000, 0.9238795325112867385, 1.000000000000000000, 0.9238795325112867385, 1.000000000000000000, 0.9238795325112867385, 1.000000000000000000, 0.9238795325112867385, 1.000000000000000000, 0.9238795325112867385, 1.000000000000000000, 0.9238795325112867385, 1.000000000000000000, 0.9238795325112867385, 1.000000000000000000, 0.9238795325112867385, 1.000000000000000000, 0.9238795325112867385, 1.000000000000000000, 0.9238795325112867385, 1.000000000000000000, 0.9238795325112867385, 1.000000000000000000, 0.9238795325112867385, 1.000000000000000000, 0.9238795325112867385, 1.000000000000000000, 0.9238795325112867385, 1.000000000000000000, 0.9238795325112867385, 1.000000000000000000, 0.9238795325112867385, 1.000000000000000000, 0.9238795325112867385, 1.000000000000000000, 0.9238795325112867385, 1.000000000000000000, 0.9238795325112867385, 1.000000000000000000, 0.9238795325112867385, 1.000000000000000000, 0.9238795325112867385, 1.000000000000000000, 0.9238795325112867385, 1.000000000000000000, 0.9238795325112867385, 1.000000000000000000, 0.9238795325112867385, 1.000000000000000000, 0.9238795325112867385, 1.000000000000000000, 0.9238795325112867385, 1.000000000000000000, 0.9238795325112867385, 1.000000000000000000, 0.9238795325112867385, 1.000000000000000000, 0.9238795325112867385, 1.000000000000000000, 0.9238795325112867385, 1.000000000000000000, 0.9238795325112867385, 1.000000000000000000, 0.9238795325112867385, 1.000000000000000000, 0.9238795325112867385, 1.000000000000000000, 0.9238795325112867385, 1.000000000000000000, 0.9238795325112867385, 1.000000000000000000, 0.9238795325112867385, 1.000000000000000000, 0.9238795325112867385, 1.000000000000000000, 0.9238795325112867385, 1.000000000000000000, 0.9238795325112867385, 1.000000000000000000, 0.9238795325112867385, 1.000000000000000000, 0.9238795325112867385, 1.000000000000000000, 0.9238795325112867385, 1.000000000000000000, 0.9238795325112867385, 1.000000000000000000, 0.9238795325112867385, 1.000000000000000000, 0.9238795325112867385, 1.000000000000000000, 0.9238795325112867385, 1.000000000000000000, 0.9238795325112867385, 1.000000000000000000, 0.9238795325112867385, 1.000000000000000000, 0.9238795325112867385, 1.000000000000000000, 0.9238795325112867385, 1.000000000000000000, 0.9238795325112867385, 1.000000000000000000, 0.9238795325112867385, 1.000000000000000000, 0.9238795325112867385, 1.000000000000000000, 0.9238795325112867385, 1.000000000000000000, 0.9238795325112867385, 1.000000000000000000, 0.9238795325112867385, 1.000000000000000000, 0.9238795325112867385, 1.000000000000000000, 0.9238795325112867385, 1.000000000000000000, 0.9238795325112867385, 1.000000000000000000, 0.9238795325112867385, 1.000000000000000000, 0.9238795325112867385, 1.000000000000000000, 0.9238795325112867385, 1.000000000000000000, 0.9238795325112867385, 1.000000000000000000, 0.9238795325112867385, 1.000000000000000000, 0.9238795325112867385, 1.000000000000000000, 0.9238795325112867385, 1.000000000000000000, 0.9238795325112867385, 1.000000000000000000, 0.9238795325112867385, 1.000000000000000000, 0.9238795325112867385, 1.000000000000000000, 0.9238795325112867385, 1.000000000000000000, 0.9238795325112867385, 1.000000000000000000, 0.9238795325112867385, 1.000000000000000000, 0.9238795325112867385, 1.000000000000000000, 0.9238795325112867385, 1.000000000000000000, 0.9238795325112867385, 1.000000000000000000, 0.9238795325112867385, 1.000000000000000000, 0.9238795325112867385, 1.000000000000000000, 0.9238795325112867385, 1.000000000000000000, 0.9238795325112867385, 1.000000000000000000, 0.9238795325112867385, 1.000000000000000000, 0.9238795325112867385, 1.000000000000000000, 0.9238795325112867385, 1.000000000000000000, 0.9238795325112867385, 1.000000000000000000, 0.9238795325112867385, 1.000000000000000000, 0.9238795325112867385, 1.000000000000000000, 0.9238795325112867385, 1.000000000000000000, 0.9238795325112867385, 1.000000000000000000, 0.9238795325112867385, 1.000000000000000000, 0.9238795325112867385, 1.000000000000000000, 0.9238795325112867385, 1.000000000000000000, 0.9238795325112867385, 1.000000000000000000, 0.9238795325112867385, 1.000000000000000000, 0.9238795325112867385, 1.000000000000000000, 0.9238795325112867385, 1.000000000000000000, 0.9238795325112867385, 1.000000000000000000, 0.9238795325112867385, 1.000000000000000000, 0.9238795325112867385, 1.000000000000000000, 0.9238795325112867385, 1.000000000000000000, 0.9238795325112867385, 1.000000000000000000, 0.9238795325112867385, 1.000000000000000000, 0.9238795325112867385, 1.000000000000000000, 0.9238795325112867385, 1.000000000000000000, 0.9238795325112867385, 1.000000000000000000, 0.9238795325112867385, 1.000000000000000000, 0.9238795325112867385, 1.000000000000000000, 0.9238795325112867385, 1.000000000000000000, 0.9238795325112867385, 1.000000000000000000, 0.9238795325112867385, 1.000000000000000000, 0.9238795325112867385, 1.000000000000000000, 0.9238795325112867385, 1.000000000000000000, 0.9238795325112867385, 1.000000000000000000, 0.9238795325112867385, 1.000000000000000000, 0.9238795325112867385, 1.000000000000000000, 0.9238795325112867385, 1.000000000000000000, 0.9238795325112867385, 1.000000000000000000, 0.9238795325112867385, 1.000000000000000000, 0.9238795325112867385, 1.000000000000000000, 0.9238795325112867385, 1.000000000000000000, 0.9238795325112867385, 1.000000000000000000, 0.9238795325112867385, 1.000000000000000000, 0.9238795325112867385, 1.000000000000000000, 0.9238795325112867385, 1.000000000000000000, 0.9238795325112867385, 1.000000000000000000, 0.9238795325112867385, 1.000000000000000000, 0.9238795325112867385, 1.000000000000000000, 0.9238795325112867385, 1.000000000000000000, 0.9238795325112867385, 1.000000000000000000, 0.9238795325112867385, 1.000000000000000000, 0.9238795325112867385, 1.000000000000000000, 0.9238795325112867385, 1.000000000000000000, 0.9238795325112867385, 1.000000000000000000, 0.9238795325112867385, 1.000000000000000000, 0.9238795325112867385, 1.000000000000000000, 0.9238795325112867385, 1.000000000000000000, 0.9238795325112867385, 1.000000000000000000, 0.9238795325112867385, 1.000000000000000000, 0.9238795325112867385, 1.000000000000000000, 0.9238795325112867385, 1.000000000000000000, 0.9238795325112867385, 1.000000000000000000, 0.9238795325112867385, 1.000000000000000000, 0.9238795325112867385, 1.000000000000000000, 0.9238795325112867385, 1.000000000000000000, 0.9238795325112867385, 1.000000000000000000, 0.9238795325112867385, 1.000000000000000000, 0.9238795325112867385, 1.000000000000000000, 0.9238795325112867385, 1.000000000000000000, 0.9238795325112867385, 1.000000000000000000, 0.9238795325112867385, 1.000000000000000000, 0.9238795325112867385, 1.000000000000000000, 0.9238795325112867385, 1.000000000000000000, 0.9238795325112867385, 1.000000000000000000, 0.9238795325112867385, 1.000000000000000000, 0.9238795325112867385, 1.000000000000000000, 0.9238795325112867385, 1.000000000000000000, 0.9238795325112867385, 1.000000000000000000, 0.9238795325112867385, 1.000000000000000000, 0.9238795325112867385, 1.000000000000000000, 0.9238795325112867385, 1.000000000000000000, 0.9238795325112867385, 1.000000000000000000, 0.9238795325112867385, 1.000000000000000000, 0.9238795325112867385, 1.000000000000000000, 0.9238795325112867385, 1.000000000000000000, 0.9238795325112867385, 1.000000000000000000, 0.9238795325112867385, 1.000000000000000000, 0.9238795325112867385, 1.000000000000000000, 0.9238795325112867385, 1.000000000000000000, 0.9238795325112867385, 1.000000000000000000, 0.9238795325112867385, 1.000000000000000000, 0.9238795325112867385, 1.000000000000000000, 0.9238795325112867385, 1.000000000000000000, 0.9238795325112867385, 1.000000000000000000, 0.9238795325112867385, 1.000000000000000000, 0.9238795325112867385, 1.000000000000000000, 0.9238795325112867385, 1.000000000000000000, 0.9238795325112867385, 1.000000000000000000, 0.9238795325112867385, 1.000000000000000000, 0.9238795325112867385, 1.000000000000000000, 0.9238795325112867385, 1.000000000000000000, 0.9238795325112867385, 1.000000000000000000, 0.9238795325112867385, 1.000000000000000000, 0.9238795325112867385, 1.000000000000000000, 0.9238795325112867385, 1.000000000000000000, 0.9238795325112867385, 1.000000000000000000, 0.9238795325112867385, 1.000000000000000000, 0.9238795325112867385, 1.000000000000000000, 0.9238795325112867385, 1.000000000000000000, 0.9238795325112867385, 1.000000000000000000, 0.9238795325112867385, 1.000000000000000000, 0.9238795325112867385, 1.000000000000000000, 0.9238795325112867385, 1.000000000000000000, 0.9238795325112867385, 1.000000000000000000, 0.9238795325112867385, 1.000000000000000000, 0.9238795325112867385, 1.000000000000000000, 0.9238795325112867385, 1.000000000000000000, 0.9238795325112867385, 1.000000000000000000, 0.9238795325112867385, 1.000000000000000000, 0.9238795325112867385, 1.000000000000000000, 0.9238795325112867385, 1.000000000000000000, 0.9238795325112867385, 1.000000000000000000, 0.9238795325112867385, 1.000000000000000000, 0.9238795325112867385, 1.000000000000000000, 0.9238795325112867385, 1.000000000000000000, 0.9238795325112867385, 1.000000000000000000, 0.9238795325112867385, 1.000000000000000000, 0.9238795325112867385, 1.000000000000000000, 0.9238795325112867385, 1.000000000000000000, 0.9238795325112867385, 1.000000000000000000, 0.9238795325112867385, 1.000000000000000000, 0.9238795325112867385, 1.000000000000000000, 0.9238795325112867385, 1.000000000000000000, 0.9238795325112867385, 1.000000000000000000, 0.9238795325112867385, 1.000000000000000000, 0.9238795325112867385, 1.000000000000000000, 0.9238795325112867385, 1.000000000000000000, 0.9238795325112867385, 1.000000000000000000, 0.9238795325112867385, 1.000000000000000000, 0.9238795325112867385, 1.000000000000000000, 0.9238795325112867385, 1.000000000000000000, 0.9238795325112867385, 1.000000000000000000, 0.9238795325112867385, 1.000000000000000000, 0.9238795325112867385, 1.000000000000000000, 0.9238795325112867385, 1.000000000000000000),
 ( 1.000000000000000000, 0.9238795325112867385, 1.000000000000000000, 0.9238795325112867385, 1.000000000000000000, 0.9238795325112867385, 1.000000000000000000, 0.9238795325112867385, 1.000000000000000000, 0.9238795325112867385, 1.000000000000000000, 0.9238795325112867385, 1.000000000000000000, 0.9238795325112867385, 1.000000000000000000, 0.9238795325112867385, 1.000000000000000000, 0.9238795325112867385, 1.000000000000000000, 0.9238795325112867385, 1.000000000000000000, 0.9238795325112867385, 1.000000000000000000, 0.9238795325112867385, 1.000000000000000000, 0.9238795325112867385, 1.000000000000000000, 0.9238795325112867385, 1.000000000000000000, 0.9238795325112867385, 1.000000000000000000, 0.9238795325112867385, 1.000000000000000000, 0.9238795325112867385, 1.000000000000000000, 0.9238795325112867385, 1.000000000000000000, 0.9238795325112867385, 1.000000000000000000, 0.9238795325112867385, 1.000000000000000000, 0.9238795325112867385, 1.000000000000000000, 0.9238795325112867385, 1.000000000000000000, 0.9238795325112867385, 1.000000000000000000, 0.9238795325112867385, 1.000000000000000000, 0.9238795325112867385, 1.000000000000000000, 0.9238795325112867385, 1.000000000000000000, 0.9238795325112867385, 1.000000000000000000, 0.9238795325112867385, 1.000000000000000000, 0.9238795325112867385, 1.000000000000000000, 0.9238795325112867385, 1.000000000000000000, 0.9238795325112867385, 1.000000000000000000, 0.9238795325112867385, 1.000000000000000000, 0.9238795325112867385, 1.000000000000000000, 0.9238795325112867385, 1.000000000000000000, 0.9238795325112867385, 1.000000000000000000, 0.9238795325112867385, 1.000000000000000000, 0.9238795325112867385, 1.000000000000000000, 0.9238795325112867385, 1.000000000000000000, 0.9238795325112867385, 1.000000000000000000, 0.9238795325112867385, 1.000000000000000000, 0.9238795325112867385, 1.000000000000000000, 0.9238795325112867385, 1.000000000000000000, 0.9238795325112867385, 1.000000000000000000, 0.9238795325112867385, 1.000000000000000000, 0.9238795325112867385, 1.000000000000000000, 0.9238795325112867385, 1.000000000000000000, 0.9238795325112867385, 1.000000000000000000, 0.9238795325112867385, 1.000000000000000000, 0.9238795325112867385, 1.000000000000000000, 0.9238795325112867385, 1.000000000000000000, 0.9238795325112867385, 1.000000000000000000, 0.9238795325112867385, 1.000000000000000000, 0.9238795325112867385, 1.000000000000000000, 0.9238795325112867385, 1.000000000000000000, 0.9238795325112867385, 1.000000000000000000, 0.9238795325112867385, 1.000000000000000000, 0.9238795325112867385, 1.000000000000000000, 0.9238795325112867385, 1.000000000000000000, 0.9238795325112867385, 1.000000000000000000, 0.9238795325112867385, 1.000000000000000000, 0.9238795325112867385, 1.000000000000000000, 0.9238795325112867385, 1.000000000000000000, 0.9238795325112867385, 1.000000000000000000, 0.9238795325112867385, 1.000000000000000000, 0.9238795325112867385, 1.000000000000000000, 0.9238795325112867385, 1.000000000000000000, 0.9238795325112867385, 1.000000000000000000, 0.9238795325112867385, 1.000000000000000000, 0.9238795325112867385, 1.000000000000000000, 0.9238795325112867385, 1.000000000000000000, 0.9238795325112867385, 1.000000000000000000, 0.9238795325112867385, 1.000000000000000000, 0.9238795325112867385, 1.000000000000000000, 0.9238795325112867385, 1.000000000000000000, 0.9238795325112867385, 1.000000000000000000, 0.9238795325112867385, 1.000000000000000000, 0.9238795325112867385, 1.000000000000000000, 0.9238795325112867385, 1.000000000000000000, 0.9238795325112867385, 1.000000000000000000, 0.9238795325112867385, 1.000000000000000000, 0.9238795325112867385, 1.000000000000000000, 0.9238795325112867385, 1.000000000000000000, 0.9238795325112867385, 1.000000000000000000, 0.9238795325112867385, 1.000000000000000000, 0.9238795325112867385, 1.000000000000000000, 0.9238795325112867385, 1.000000000000000000, 0.9238795325112867385, 1.000000000000000000, 0.9238795325112867385, 1.000000000000000000, 0.9238795325112867385, 1.000000000000000000, 0.9238795325112867385, 1.000000000000000000, 0.9238795325112867385, 1.000000000000000000, 0.9238795325112867385, 1.000000000000000000, 0.9238795325112867385, 1.000000000000000000, 0.9238795325112867385, 1.000000000000000000, 0.9238795325112867385, 1.000000000000000000, 0.9238795325112867385, 1.000000000000000000, 0.9238795325112867385, 1.000000000000000000, 0.9238795325112867385, 1.000000000000000000, 0.9238795325112867385, 1.000000000000000000, 0.9238795325112867385, 1.000000000000000000, 0.9238795325112867385, 1.000000000000000000, 0.9238795325112867385, 1.000000000000000000, 0.9238795325112867385, 1.000000000000000000, 0.9238795325112867385, 1.000000000000000000, 0.9238795325112867385, 1.000000000000000000, 0.9238795325112867385, 1.000000000000000000, 0.9238795325112867385, 1.000000000000000000, 0.9238795325112867385, 1.000000000000000000, 0.9238795325112867385, 1.000000000000000000, 0.9238795325112867385, 1.000000000000000000, 0.9238795325112867385, 1.000000000000000000, 0.9238795325112867385, 1.000000000000000000, 0.9238795325112867385, 1.000000000000000000, 0.9238795325112867385, 1.000000000000000000, 0.9238795325112867385, 1.000000000000000000, 0.9238795325112867385, 1.000000000000000000, 0.9238795325112867385, 1.000000000000000000, 0.9238795325112867385, 1.000000000000000000, 0.9238795325112867385, 1.000000000000000000, 0.9238795325112867385, 1.000000000000000000, 0.9238795325112867385, 1.000000000000000000, 0.9238795325112867385, 1.000000000000000000, 0.9238795325112867385, 1.000000000000000000, 0.9238795325112867385, 1.000000000000000000, 0.9238795325112867385, 1.000000000000000000, 0.9238795325112867385, 1.000000000000000000, 0.9238795325112867385, 1.000000000000000000, 0.9238795325112867385, 1.000000000000000000, 0.9238795325112867385, 1.000000000000000000, 0.9238795325112867385, 1.000000000000000000, 0.9238795325112867385, 1.000000000000000000, 0.9238795325112867385, 1.000000000000000000, 0.9238795325112867385, 1.000000000000000000, 0.9238795325112867385, 1.000000000000000000, 0.9238795325112867385, 1.000000000000000000, 0.9238795325112867385, 1.000000000000000000, 0.9238795325112867385, 1.000000000000000000, 0.9238795325112867385, 1.000000000000000000, 0.9238795325112867385, 1.000000000000000000, 0.9238795325112867385, 1.000000000000000000, 0.9238795325112867385, 1.000000000000000000, 0.9238795325112867385, 1.000000000000000000, 0.9238795325112867385, 1.000000000000000000, 0.9238795325112867385, 1.000000000000000000, 0.9238795325112867385, 1.000000000000000000, 0.9238795325112867385, 1.000000000000000000, 0.9238795325112867385, 1.000000000000000000, 0.9238795325112867385, 1.000000000000000000, 0.9238795325112867385, 1.000000000000000000, 0.9238795325112867385, 1.000000000000000000, 0.9238795325112867385, 1.000000000000000000, 0.9238795325112867385, 1.000000000000000000, 0.9238795325112867385, 1.000000000000000000, 0.9238795325112867385, 1.000000000000000000, 0.9238795325112867385, 1.000000000000000000, 0.9238795325112867385, 1.000000000000000000, 0.9238795325112867385, 1.000000000000000000, 0.9238795325112867385, 1.000000000000000000, 0.9238795325112867385, 1.000000000000000000, 0.9238795325112867385, 1.000000000000000000, 0.9238795325112867385, 1.000000000000000000, 0.9238795325112867385, 1.000000000000000000, 0.9238795325112867385, 1.000000000000000000, 0.9238795325112867385, 1.000000000000000000, 0.9238795325112867385, 1.000000000000000000, 0.9238795325112867385, 1.000000000000000000, 0.9238795325112867385, 1.000000000000000000, 0.9238795325112867385, 1.000000000000000000, 0.9238795325112867385, 1.000000000000000000, 0.9238795325112867385, 1.000000000000000000, 0.9238795325112867385, 1.000000000000000000, 0.9238795325112867385, 1.000000000000000000, 0.9238795325112867385, 1.000000000000000000, 0.9238795325112867385, 1.000000000000000000, 0.9238795325112867385, 1.000000000000000000, 0.9238795325112867385, 1.000000000000000000, 0.9238795325112867385, 1.000000000000000000, 0.9238795325112867385, 1.000000000000000000, 0.9238795325112867385, 1.000000000000000000, 0.9238795325112867385, 1.000000000000000000, 0.9238795325112867385, 1.000000000000000000, 0.9238795325112867385, 1.000000000000000000, 0.9238795325112867385, 1.000000000000000000, 0.9238795325112867385, 1.000000000000000000, 0.9238795325112867385, 1.000000000000000000, 0.9238795325112867385, 1.000000000000000000, 0.9238795325112867385, 1.000000000000000000, 0.9238795325112867385, 1.000000000000000000, 0.9238795325112867385, 1.000000000000000000, 0.9238795325112867385, 1.000000000000000000, 0.9238795325112867385, 1.000000000000000000, 0.9238795325112867385, 1.000000000000000000, 0.9238795325112867385, 1.000000000000000000, 0.9238795325112867385, 1.000000000000000000, 0.9238795325112867385, 1.000000000000000000, 0.9238795325112867385, 1.000000000000000000, 0.9238795325112867385, 1.000000000000000000, 0.9238795325112867385, 1.000000000000000000, 0.9238795325112867385, 1.000000000000000000, 0.9238795325112867385, 1.000000000000000000, 0.9238795325112867385, 1.000000000000000000, 0.9238795325112867385, 1.000000000000000000, 0.9238795325112867385, 1.000000000000000000, 0.9238795325112867385, 1.000000000000000000, 0.9238795325112867385, 1.000000000000000000, 0.9238795325112867385, 1.000000000000000000, 0.9238795325112867385, 1.000000000000000000, 0.9238795325112867385, 1.000000000000000000, 0.9238795325112867385, 1.000000000000000000, 0.9238795325112867385, 1.000000000000000000, 0.9238795325112867385, 1.000000000000000000, 0.9238795325112867385, 1.000000000000000000, 0.9238795325112867385, 1.000000000000000000, 0.9238795325112867385, 1.000000000000000000, 0.9238795325112867385, 1.000000000000000000, 0.9238795325112867385, 1.000000000000000000, 0.9238795325112867385, 1.000000000000000000, 0.9238795325112867385, 1.000000000000000000, 0.9238795325112867385, 1.000000000000000000, 0.9238795325112867385, 1.000000000000000000, 0.9238795325112867385, 1.000000000000000000, 0.9238795325112867385, 1.000000000000000000, 0.9238795325112867385, 1.000000000000000000, 0.9238795325112867385, 1.000000000000000000, 0.9238795325112867385, 1.000000000000000000, 0.9238795325112867385, 1.000000000000000000, 0.9238795325112867385, 1.000000000000000000, 0.9238795325112867385, 1.000000000000000000, 0.9238795325112867385, 1.000000000000000000, 0.9238795325112867385, 1.000000000000000000, 0.9238795325112867385, 1.000000000000000000, 0.9238795325112867385, 1.000000000000000000, 0.9238795325112867385, 1.000000000000000000, 0.9238795325112867385, 1.000000000000000000, 0.9238795325112867385, 1.000000000000000000, 0.9238795325112867385, 1.000000000000000000, 0.9238795325112867385, 1.000000000000000000, 0.9238795325112867385, 1.000000000000000000, 0.9238795325112867385, 1.000000000000000000, 0.9238795325112867385, 1.000000000000000000) ) ) 
 REPRESENTATION_ITEM ( '' )  SURFACE ( )  );
#1795=LINE ( 'NONE', #34911, #26498 ) ;
#1805=CARTESIAN_POINT ( 'NONE',  ( -54.64476657466781973, -151.0625000013656063, -4.444560631937228834 ) ) ;
#1806=CARTESIAN_POINT ( 'NONE',  ( -50.70258187064364108, -142.1250000013656063, 2.196230717870141014 ) ) ;
#1815=ORIENTED_EDGE ( 'NONE', *, *, #30216, .T. ) ;
#1818=CARTESIAN_POINT ( 'NONE',  ( -58.24261429053147765, -136.2500000000000284, -3.805975901505573855 ) ) ;
#1844=CARTESIAN_POINT ( 'NONE',  ( -54.60164318462004474, -142.3750000000000284, -4.984105922594373794 ) ) ;
#1853=CARTESIAN_POINT ( 'NONE',  ( -55.35523342533222291, -141.5625000013656063, 4.444560631937231499 ) ) ;
#1855=CARTESIAN_POINT ( 'NONE',  ( -60.14911071818854538, -135.1875000027312410, 1.666127454062681368 ) ) ;
#1869=CARTESIAN_POINT ( 'NONE',  ( -50.55543936806279248, -127.0625000013655921, 0.3552334253322060320 ) ) ;
#1884=CARTESIAN_POINT ( 'NONE',  ( -51.60603307380591787, -133.9375000013656063, -2.891590998281053704 ) ) ;
#1894=CARTESIAN_POINT ( 'NONE',  ( -50.70258187064364108, -133.3750000013656063, 2.196230717870141014 ) ) ;
#1906=AXIS2_PLACEMENT_3D ( 'NONE', #49615, #58077, #23369 ) ;
#1907=CARTESIAN_POINT ( 'NONE',  ( -53.33387254593710480, -138.9375000027312126, 5.149110718188539160 ) ) ;
#1921=CARTESIAN_POINT ( 'NONE',  ( -58.39396692619412477, -138.4375000013656063, 2.891590998281057701 ) ) ;
#1927=CARTESIAN_POINT ( 'NONE',  ( -50.01589407740564042, -153.6250000000000284, 0.3983568153799778022 ) ) ;
#1933=PRESENTATION_STYLE_ASSIGNMENT (( #51754 ) ) ;
#1939=CARTESIAN_POINT ( 'NONE',  ( -55.35523342533222291, -154.5625000013656347, 4.444560631937231499 ) ) ;
#1941=CARTESIAN_POINT ( 'NONE',  ( -59.98410592259440222, -145.2500000027312126, -0.3983568153799752487 ) ) ;
#1942=( BOUNDED_CURVE ( )  B_SPLINE_CURVE ( 2, ( #9601, #63025, #14108, #63650, #63332, #34046, #28273, #4774, #47888 ),
 .UNSPECIFIED., .F., .F. ) 
 B_SPLINE_CURVE_WITH_KNOTS ( ( 3, 2, 2, 2, 3 ),
 ( 0.3416666666666669516, 0.3458333333333336035, 0.3500000000000002554, 0.3541666666666669627, 0.3583333333333336146 ),
 .UNSPECIFIED. ) 
 CURVE ( )  GEOMETRIC_REPRESENTATION_ITEM ( )  RATIONAL_B_SPLINE_CURVE ( ( 0.9999999999999948930, 0.9238795325112918455, 1.000000000000000000, 0.9238795325112867385, 1.000000000000000000, 0.9238795325112867385, 1.000000000000000000, 0.9238795325112816315, 1.000000000000005107 ) ) 
 REPRESENTATION_ITEM ( '' )  );
#1961=CARTESIAN_POINT ( 'NONE',  ( -56.48576386720575471, -149.7500000013656063, -4.591703134518078322 ) ) ;
#1977=CARTESIAN_POINT ( 'NONE',  ( -58.80597590150559739, -152.1250000027312126, 3.242614290531460330 ) ) ;
#2005=CARTESIAN_POINT ( 'NONE',  ( -58.39396692619412477, -136.6875000013656063, 2.891590998281057701 ) ) ;
#2046=CARTESIAN_POINT ( 'NONE',  ( -55.35523342533222291, -141.5625000013656063, 4.444560631937231499 ) ) ;
#2081=CARTESIAN_POINT ( 'NONE',  ( -54.64476657466781973, -148.0625000013656063, -4.444560631937228834 ) ) ;
#2097=CARTESIAN_POINT ( 'NONE',  ( -53.33387254593733928, -125.8125000000000142, 5.149110718188519620 ) ) ;
#2105=CARTESIAN_POINT ( 'NONE',  ( -59.29741812935640155, -147.6250000013655779, -2.196230717870135685 ) ) ;
#2106=CARTESIAN_POINT ( 'NONE',  ( -59.98410592259440222, -150.2500000027312126, -0.3983568153799752487 ) ) ;
#2112=CARTESIAN_POINT ( 'NONE',  ( -52.53715891517739323, -152.5625000027311842, -4.819101127000233298 ) ) ;
#2128=CARTESIAN_POINT ( 'NONE',  ( -50.40829686548195099, -151.2500000013656063, -1.485763867205728284 ) ) ;
#2129=CARTESIAN_POINT ( 'NONE',  ( -52.10840900171896806, -142.1875000013656063, 3.393966926194110556 ) ) ;
#2165=CARTESIAN_POINT ( 'NONE',  ( -56.66612745406270335, -139.3125000000000284, -5.149110718188516067 ) ) ;
#2175=CARTESIAN_POINT ( 'NONE',  ( -52.80376928212989185, -144.1250000013656063, -4.297418129356378458 ) ) ;
#2178=CARTESIAN_POINT ( 'NONE',  ( -51.75738570946856498, -130.8750000027312126, 3.805975901505576964 ) ) ;
#2190=CARTESIAN_POINT ( 'NONE',  ( -57.19623071787017210, -128.3750000013656631, 4.297418129356382899 ) ) ;
#2203=CARTESIAN_POINT ( 'NONE',  ( -54.64476657466781973, -132.8125000013656063, -4.444560631937228834 ) ) ;
#2213=CARTESIAN_POINT ( 'NONE',  ( -56.48576386720575471, -127.0000000013656063, -4.591703134518078322 ) ) ;
#2239=CARTESIAN_POINT ( 'NONE',  ( -52.80376928212989185, -138.8750000013656063, -4.297418129356378458 ) ) ;
#2243=CARTESIAN_POINT ( 'NONE',  ( -51.75738570946856498, -148.7500000000000284, 3.805975901505576964 ) ) ;
#2244=CARTESIAN_POINT ( 'NONE',  ( -59.81910112700025905, -154.1875000000000000, -2.462841084822630311 ) ) ;
#2255=CARTESIAN_POINT ( 'NONE',  ( -50.18089887299979068, -147.8125000027312126, 2.462841084822635640 ) ) ;
#2275=CARTESIAN_POINT ( 'NONE',  ( -54.64476657466781973, -144.8125000013656063, -4.444560631937228834 ) ) ;
#2280=CARTESIAN_POINT ( 'NONE',  ( -58.24261429053147765, -141.3750000027312126, -3.805975901505573855 ) ) ;
#2317=CARTESIAN_POINT ( 'NONE',  ( -57.19623071787017210, -134.6250000013656347, 4.297418129356382899 ) ) ;
#2356=CARTESIAN_POINT ( 'NONE',  ( -57.89159099828107458, -140.9375000013656063, -3.393966926194107447 ) ) ;
#2387=CARTESIAN_POINT ( 'NONE',  ( -58.39396692619412477, -148.6875000013656063, 2.891590998281057701 ) ) ;
#2394=DIRECTION ( 'NONE',  ( 0.000000000000000000, 1.000000000000000000, 0.000000000000000000 ) ) ;
#2398=CARTESIAN_POINT ( 'NONE',  ( -59.98410592259440222, -126.1250000000000142, -0.3983568153799752487 ) ) ;
#2404=CARTESIAN_POINT ( 'NONE',  ( -59.29741812935640155, -148.6250000013656063, -2.196230717870135685 ) ) ;
#2425=VERTEX_POINT ( 'NONE', #30148 ) ;
#2430=CARTESIAN_POINT ( 'NONE',  ( -58.39396692619412477, -153.6875000013656063, 2.891590998281057701 ) ) ;
#2431=( BOUNDED_SURFACE ( )  B_SPLINE_SURFACE ( 1, 2, ( 
 ( #33164, #56669, #12587, #31891, #32200, #8091, #7769, #8706, #32842, #52778, #12897, #52470, #7460, #32519, #52149, #37662, #57303, #8406, #28007, #47625, #3581, #23188, #18359, #37984, #28634, #33782, #10289, #29894, #39543, #4826, #5146, #58226, #49524, #24446, #9331, #53399, #48569, #44049, #24766, #5465, #53088, #4509, #59181, #15115, #24135, #34399, #13844, #34732, #54359, #63381, #9024, #19617, #25081, #44690, #651, #33464, #28944, #48251, #4207, #43738, #20263, #57926, #23820, #16, #44370, #14155, #43424, #39229, #19296, #38914, #58548, #58853, #331, #63068, #18980, #14470, #38593, #34090, #53714, #9646, #29576, #14784, #29255, #48880, #54027, #9963, #49207, #19931, #26354, #36014, #25402, #10598, #20905, #15443, #16071, #41139, #6114, #11560, #30865, #49838, #30538, #2255, #35062, #11870, #25729, #35699, #54994, #21216, #60787, #26045, #6746, #10920, #40508, #31486, #60150, #5781, #45660, #54674, #50159, #46298, #55326, #30213, #50494, #45976, #39862, #51131, #45340, #55646, #35371, #6434, #16395, #45021, #16712, #988, #20591, #11241, #36328, #40197, #7066, #1309, #1617, #40824, #1941, #59833, #60470, #31179, #50809, #21543, #15755, #55956, #26679, #59506, #42404, #47250, #2559, #36642, #26994, #47552, #32446, #3502, #41771, #27620, #42720, #46613, #22173, #37910, #61420, #17663, #31813, #18286, #22812, #17344, #57541, #3196, #22496, #12513, #36963, #28245, #32124, #56593, #51760, #56907, #7387, #47859, #7704, #23116, #13467, #33085, #56274, #62363, #52699, #8016, #27307, #8633, #12197, #46932, #62047, #21859, #17963, #37279, #41454, #2882, #61103, #17028, #42092, #51448, #61734, #12826, #37586, #52075, #57227, #13146, #32766, #52397, #8332, #27931, #18905, #28873, #48180, #53638, #48804, #58147, #23440, #4743, #34016, #63616, #34325, #53325, #9881, #19853, #9571, #10211, #57851, #59104, #53950, #48495, #18603, #14394, #29178, #38229, #39467, #19215, #14076, #8945, #19537, #24368, #15031, #29487, #4432, #24059, #49123, #43970, #38832, #13769, #43656, #39151, #33705, #34647, #63297, #33391, #58776, #14706, #58469, #255, #5065, #9258, #54271, #53006, #23754, #24685, #44293, #29814, #28559, #3817, #43041, #62681, #4132, #43349, #62995, #38519, #49761, #55564, #5388, #50720, #54913, #26271, #6664, #49446, #45893, #40106, #60065, #25003, #6355, #30132, #41061, #16315, #25643, #20182, #20824, #55240, #21137, #44613, #25959, #1855, #21461, #45576, #11162, #5707, #573, #54596, #11479, #15989, #31099, #25322, #30784, #60708, #10518, #44942, #16628, #900, #45259, #59427, #36249, #50407, #55876, #15674, #1532, #39780, #11788, #15356, #10840, #34981, #40742, #20507, #59749, #35293, #30456, #50081, #6038, #1225, #40425, #35614, #60389, #35936, #42014, #42330, #31738, #47473, #61654, #46538, #7309, #22092, #17588, #61970, #42646, #26599, #41691, #13066, #61338, #26922, #17261, #3114, #37205, #41375, #2479, #36884, #46215, #32686, #12435, #17891, #27539, #16947, #2178, #32047, #6987, #7624, #52317, #56514, #22732, #22415, #61021, #51683, #57464, #21783, #3427, #27228, #46849, #2796, #12749, #8252, #56831, #37511, #32369, #51993, #23043, #7937, #36560, #47171, #56191, #57151, #37830, #27852, #12111, #62287, #18209, #31406, #51044, #51368, #29096, #8869, #4355, #53560, #62603, #53871, #8555, #28168, #48411, #9798, #3740, #24607, #43270, #14001, #48100, #19459, #47783, #23975, #19135, #34242, #28484, #38442, #57771, #63220, #58391, #4054, #33004, #14317, #43577, #9485, #43888, #62910, #39073, #29406, #38752, #19778, #23361, #4984, #63536, #58069, #42960, #33939, #48723, #18526, #49039, #28795, #23672, #38146, #4663, #24285, #44213, #58701, #33628, #53247, #14629, #178, #39386, #13693, #9183, #13383, #18823, #52621, #33312, #52932, #25562, #1145, #40024, #55484, #20745, #49685, #31018, #24928, #15273 ),
 ( #60311, #819, #35858, #16239, #59017, #11400, #5630, #5952, #34558, #15914, #39702, #50646, #25881, #35217, #29734, #30378, #59342, #6584, #40349, #59668, #25241, #54519, #1781, #44856, #493, #20424, #50001, #44536, #21381, #15599, #40667, #26199, #45819, #49366, #21062, #14948, #45179, #10442, #54189, #5310, #30056, #59991, #10127, #35535, #10767, #20096, #34897, #54837, #55163, #11082, #30704, #50329, #6275, #45497, #1461, #36486, #36810, #56754, #3041, #55797, #17514, #41298, #47093, #60632, #42257, #46460, #17816, #61898, #40988, #37441, #31661, #51611, #16552, #61579, #21706, #32609, #7858, #17184, #11714, #12362, #60947, #57072, #46772, #41610, #51297, #56112, #47403, #7233, #46139, #26847, #31976, #26521, #3354, #2404, #22659, #52235, #12984, #31332, #8177, #27779, #27156, #12036, #36176, #50967, #22016, #22340, #6910, #2718, #56440, #2105, #16868, #61260, #7544, #41938, #37134, #12677, #32291, #51917, #27464, #18447, #18751, #38678, #48648, #37754, #43819, #38070, #48027, #3667, #9108, #4285, #13624, #42571, #23904, #53174, #19060, #53485, #8795, #29024, #39000, #28715, #29331, #13307, #14552, #9413, #3977, #57386, #33553, #48338, #32930, #58632, #38375, #33242, #28094, #58317, #43504, #34171, #4590, #23597, #43194, #24213, #63149, #58002, #52553, #62836, #14242, #52862, #53794, #13928, #8485, #33865, #63465, #19384, #9728, #48961, #28407, #22971, #47712, #42883, #62211, #18127, #23280, #62528, #57698, #55081, #4913, #5550, #40592, #39946, #12207, #58940, #61111, #35460, #49611, #19702, #15527, #54763, #39312, #20989, #20347, #15197, #10050, #20675, #10691, #17036, #30625, #29982, #25162, #11003, #49921, #59594, #14869, #44776, #30301, #59265, #36651, #738, #34478, #35147, #5874, #25482, #1388, #45103, #34822, #56281, #54110, #24854, #54445, #1068, #40281, #29663, #59920, #50247, #24533, #15841, #31825, #6195, #25810, #5234, #45423, #44136, #106, #10373, #49294, #44458, #418, #20021, #39627, #62056, #27001, #8339, #32131, #43049, #18295, #27629, #22180, #22823, #51767, #3826, #57237, #52085, #42098, #46943, #57858, #61744, #56603, #17672, #42413, #36975, #13779, #37286, #33092, #62689, #23446, #41783, #13476, #18610, #37593, #2891, #8641, #61428, #22503, #32773, #38238, #13153, #3203, #51457, #12520, #7394, #46620, #7711, #17351, #2566, #27315, #52408, #52707, #56915, #47258, #3512, #28254, #12833, #47867, #32453, #8023, #17969, #27938, #47562, #23123, #42727, #62372, #37918, #57548, #268, #19229, #39480, #49460, #63629, #58479, #14089, #19549, #14718, #24070, #53016, #34338, #39163, #29503, #19866, #38845, #59116, #5400, #58788, #39795, #23761, #25016, #15045, #14405, #48188, #43982, #53962, #4141, #44626, #48815, #43666, #38528, #49135, #9894, #585, #34664, #34027, #53648, #54283, #5078, #4753, #43358, #9582, #24700, #63307, #20193, #29188, #63005, #44304, #10221, #24381, #29827, #59441, #33401, #8957, #18914, #53333, #28567, #58156, #33714, #9267, #28882, #48503, #4440, #16003, #51057, #50425, #55577, #15687, #21473, #34993, #16641, #20837, #55889, #36263, #15370, #11803, #6050, #25973, #54608, #35949, #59761, #7001, #45907, #55255, #49773, #6368, #35307, #31418, #21151, #35627, #25658, #10853, #21794, #45271, #20521, #1237, #45589, #916, #41389, #40439, #60718, #26610, #46227, #5719, #41072, #2190, #1547, #30468, #10532, #25334, #50096, #60404, #30144, #40755, #30797, #44956, #40120, #54927, #60081, #11174, #16329, #11495, #31111, #50733, #6677, #26284, #1869, #13079, #23054, #12126, #18220, #12447, #41702, #52634, #27866, #37217, #31749, #32383, #61350, #13395, #3125, #61668, #51695, #56527, #3752, #7636, #2493, #27241, #52008, #46550, #23374, #46865, #42659, #8568, #33018, #51381, #62298, #28179, #47183, #32059, #37846, #7323, #2809, #42343, #47795, #22746, #12760, #61037, #22109 ) ),
 .UNSPECIFIED., .F., .F., .F. ) 
 B_SPLINE_SURFACE_WITH_KNOTS ( ( 2, 2 ),
 ( 3, 2, 2, 2, 2, 2, 2, 2, 2, 2, 2, 2, 2, 2, 2, 2, 2, 2, 2, 2, 2, 2, 2, 2, 2, 2, 2, 2, 2, 2, 2, 2, 2, 2, 2, 2, 2, 2, 2, 2, 2, 2, 2, 2, 2, 2, 2, 2, 2, 2, 2, 2, 2, 2, 2, 2, 2, 2, 2, 2, 2, 2, 2, 2, 2, 2, 2, 2, 2, 2, 2, 2, 2, 2, 2, 2, 2, 2, 2, 2, 2, 2, 2, 2, 2, 2, 2, 2, 2, 2, 2, 2, 2, 2, 2, 2, 2, 2, 2, 2, 2, 2, 2, 2, 2, 2, 2, 2, 2, 2, 2, 2, 2, 2, 2, 2, 2, 2, 2, 2, 2, 2, 2, 2, 2, 2, 2, 2, 2, 2, 2, 2, 2, 2, 2, 2, 2, 2, 2, 2, 2, 2, 2, 2, 2, 2, 2, 2, 2, 2, 2, 2, 2, 2, 2, 2, 2, 2, 2, 2, 2, 2, 2, 2, 2, 2, 2, 2, 2, 2, 2, 2, 2, 2, 2, 2, 2, 2, 2, 2, 2, 2, 2, 2, 2, 2, 2, 2, 2, 2, 2, 2, 2, 2, 2, 2, 2, 2, 2, 2, 2, 2, 2, 2, 2, 2, 2, 2, 2, 2, 2, 2, 2, 2, 2, 2, 2, 2, 2, 2, 2, 2, 2, 2, 2, 2, 2, 2, 2, 2, 2, 2, 2, 2, 2, 2, 2, 2, 2, 2, 3 ),
 ( 0.000000000000000000, 1.000000000000000000 ),
 ( 0.000000000000000000, 0.004166666666666666609, 0.008333333333333333218, 0.01250000000000000069, 0.01666666666666666644, 0.02083333333333333218, 0.02500000000000000139, 0.02916666666666666713, 0.03333333333333333287, 0.03749999999999999861, 0.04166666666666666435, 0.04583333333333333010, 0.05000000000000000278, 0.05416666666666666852, 0.05833333333333333426, 0.06250000000000000000, 0.06666666666666666574, 0.07083333333333333148, 0.07499999999999999722, 0.07916666666666666297, 0.08333333333333332871, 0.08749999999999999445, 0.09166666666666666019, 0.09583333333333333981, 0.1000000000000000056, 0.1041666666666666713, 0.1083333333333333370, 0.1125000000000000028, 0.1166666666666666685, 0.1208333333333333343, 0.1250000000000000000, 0.1291666666666666796, 0.1333333333333333315, 0.1375000000000000111, 0.1416666666666666630, 0.1458333333333333426, 0.1499999999999999944, 0.1541666666666666741, 0.1583333333333333259, 0.1625000000000000056, 0.1666666666666666574, 0.1708333333333333370, 0.1749999999999999889, 0.1791666666666666685, 0.1833333333333333204, 0.1875000000000000000, 0.1916666666666666796, 0.1958333333333333315, 0.2000000000000000111, 0.2041666666666666630, 0.2083333333333333426, 0.2124999999999999944, 0.2166666666666666741, 0.2208333333333333259, 0.2250000000000000056, 0.2291666666666666574, 0.2333333333333333370, 0.2374999999999999889, 0.2416666666666666685, 0.2458333333333333204, 0.2500000000000000000, 0.2541666666666666519, 0.2583333333333333592, 0.2625000000000000111, 0.2666666666666666630, 0.2708333333333333148, 0.2750000000000000222, 0.2791666666666666741, 0.2833333333333333259, 0.2874999999999999778, 0.2916666666666666852, 0.2958333333333333370, 0.2999999999999999889, 0.3041666666666666408, 0.3083333333333333481, 0.3125000000000000000, 0.3166666666666666519, 0.3208333333333333592, 0.3250000000000000111, 0.3291666666666666630, 0.3333333333333333148, 0.3375000000000000222, 0.3416666666666666741, 0.3458333333333333259, 0.3499999999999999778, 0.3541666666666666852, 0.3583333333333333370, 0.3624999999999999889, 0.3666666666666666408, 0.3708333333333333481, 0.3750000000000000000, 0.3791666666666666519, 0.3833333333333333592, 0.3875000000000000111, 0.3916666666666666630, 0.3958333333333333148, 0.4000000000000000222, 0.4041666666666666741, 0.4083333333333333259, 0.4124999999999999778, 0.4166666666666666852, 0.4208333333333333370, 0.4249999999999999889, 0.4291666666666666408, 0.4333333333333333481, 0.4375000000000000000, 0.4416666666666666519, 0.4458333333333333592, 0.4500000000000000111, 0.4541666666666666630, 0.4583333333333333148, 0.4625000000000000222, 0.4666666666666666741, 0.4708333333333333259, 0.4749999999999999778, 0.4791666666666666852, 0.4833333333333333370, 0.4874999999999999889, 0.4916666666666666408, 0.4958333333333333481, 0.5000000000000000000, 0.5041666666666666519, 0.5083333333333333037, 0.5124999999999999556, 0.5166666666666667185, 0.5208333333333333703, 0.5250000000000000222, 0.5291666666666666741, 0.5333333333333333259, 0.5374999999999999778, 0.5416666666666666297, 0.5458333333333332815, 0.5500000000000000444, 0.5541666666666666963, 0.5583333333333333481, 0.5625000000000000000, 0.5666666666666666519, 0.5708333333333333037, 0.5749999999999999556, 0.5791666666666667185, 0.5833333333333333703, 0.5875000000000000222, 0.5916666666666666741, 0.5958333333333333259, 0.5999999999999999778, 0.6041666666666666297, 0.6083333333333332815, 0.6125000000000000444, 0.6166666666666666963, 0.6208333333333333481, 0.6250000000000000000, 0.6291666666666666519, 0.6333333333333333037, 0.6374999999999999556, 0.6416666666666667185, 0.6458333333333333703, 0.6500000000000000222, 0.6541666666666666741, 0.6583333333333333259, 0.6624999999999999778, 0.6666666666666666297, 0.6708333333333332815, 0.6750000000000000444, 0.6791666666666666963, 0.6833333333333333481, 0.6875000000000000000, 0.6916666666666666519, 0.6958333333333333037, 0.6999999999999999556, 0.7041666666666667185, 0.7083333333333333703, 0.7125000000000000222, 0.7166666666666666741, 0.7208333333333333259, 0.7249999999999999778, 0.7291666666666666297, 0.7333333333333332815, 0.7375000000000000444, 0.7416666666666666963, 0.7458333333333333481, 0.7500000000000000000, 0.7541666666666666519, 0.7583333333333333037, 0.7624999999999999556, 0.7666666666666667185, 0.7708333333333333703, 0.7750000000000000222, 0.7791666666666666741, 0.7833333333333333259, 0.7874999999999999778, 0.7916666666666666297, 0.7958333333333332815, 0.8000000000000000444, 0.8041666666666666963, 0.8083333333333333481, 0.8125000000000000000, 0.8166666666666666519, 0.8208333333333333037, 0.8249999999999999556, 0.8291666666666667185, 0.8333333333333333703, 0.8375000000000000222, 0.8416666666666666741, 0.8458333333333333259, 0.8499999999999999778, 0.8541666666666666297, 0.8583333333333332815, 0.8625000000000000444, 0.8666666666666666963, 0.8708333333333333481, 0.8750000000000000000, 0.8791666666666666519, 0.8833333333333333037, 0.8874999999999999556, 0.8916666666666667185, 0.8958333333333333703, 0.9000000000000000222, 0.9041666666666666741, 0.9083333333333333259, 0.9124999999999999778, 0.9166666666666666297, 0.9208333333333332815, 0.9250000000000000444, 0.9291666666666666963, 0.9333333333333333481, 0.9375000000000000000, 0.9416666666666666519, 0.9458333333333333037, 0.9499999999999999556, 0.9541666666666667185, 0.9583333333333333703, 0.9625000000000000222, 0.9666666666666666741, 0.9708333333333333259, 0.9749999999999999778, 0.9791666666666666297, 0.9833333333333332815, 0.9875000000000000444, 0.9916666666666666963, 0.9958333333333333481, 1.000000000000000000 ),
 .UNSPECIFIED. ) 
 GEOMETRIC_REPRESENTATION_ITEM ( )  RATIONAL_B_SPLINE_SURFACE ( (
 ( 1.000000000000000000, 0.9238795325112867385, 1.000000000000000000, 0.9238795325112867385, 1.000000000000000000, 0.9238795325112867385, 1.000000000000000000, 0.9238795325112867385, 1.000000000000000000, 0.9238795325112867385, 1.000000000000000000, 0.9238795325112867385, 1.000000000000000000, 0.9238795325112867385, 1.000000000000000000, 0.9238795325112867385, 1.000000000000000000, 0.9238795325112867385, 1.000000000000000000, 0.9238795325112867385, 1.000000000000000000, 0.9238795325112867385, 1.000000000000000000, 0.9238795325112867385, 1.000000000000000000, 0.9238795325112867385, 1.000000000000000000, 0.9238795325112867385, 1.000000000000000000, 0.9238795325112867385, 1.000000000000000000, 0.9238795325112867385, 1.000000000000000000, 0.9238795325112867385, 1.000000000000000000, 0.9238795325112867385, 1.000000000000000000, 0.9238795325112867385, 1.000000000000000000, 0.9238795325112867385, 1.000000000000000000, 0.9238795325112867385, 1.000000000000000000, 0.9238795325112867385, 1.000000000000000000, 0.9238795325112867385, 1.000000000000000000, 0.9238795325112867385, 1.000000000000000000, 0.9238795325112867385, 1.000000000000000000, 0.9238795325112867385, 1.000000000000000000, 0.9238795325112867385, 1.000000000000000000, 0.9238795325112867385, 1.000000000000000000, 0.9238795325112867385, 1.000000000000000000, 0.9238795325112867385, 1.000000000000000000, 0.9238795325112867385, 1.000000000000000000, 0.9238795325112867385, 1.000000000000000000, 0.9238795325112867385, 1.000000000000000000, 0.9238795325112867385, 1.000000000000000000, 0.9238795325112867385, 1.000000000000000000, 0.9238795325112867385, 1.000000000000000000, 0.9238795325112867385, 1.000000000000000000, 0.9238795325112867385, 1.000000000000000000, 0.9238795325112867385, 1.000000000000000000, 0.9238795325112867385, 1.000000000000000000, 0.9238795325112867385, 1.000000000000000000, 0.9238795325112867385, 1.000000000000000000, 0.9238795325112867385, 1.000000000000000000, 0.9238795325112867385, 1.000000000000000000, 0.9238795325112867385, 1.000000000000000000, 0.9238795325112867385, 1.000000000000000000, 0.9238795325112867385, 1.000000000000000000, 0.9238795325112867385, 1.000000000000000000, 0.9238795325112867385, 1.000000000000000000, 0.9238795325112867385, 1.000000000000000000, 0.9238795325112867385, 1.000000000000000000, 0.9238795325112867385, 1.000000000000000000, 0.9238795325112867385, 1.000000000000000000, 0.9238795325112867385, 1.000000000000000000, 0.9238795325112867385, 1.000000000000000000, 0.9238795325112867385, 1.000000000000000000, 0.9238795325112867385, 1.000000000000000000, 0.9238795325112867385, 1.000000000000000000, 0.9238795325112867385, 1.000000000000000000, 0.9238795325112867385, 1.000000000000000000, 0.9238795325112867385, 1.000000000000000000, 0.9238795325112867385, 1.000000000000000000, 0.9238795325112867385, 1.000000000000000000, 0.9238795325112867385, 1.000000000000000000, 0.9238795325112867385, 1.000000000000000000, 0.9238795325112867385, 1.000000000000000000, 0.9238795325112867385, 1.000000000000000000, 0.9238795325112867385, 1.000000000000000000, 0.9238795325112867385, 1.000000000000000000, 0.9238795325112867385, 1.000000000000000000, 0.9238795325112867385, 1.000000000000000000, 0.9238795325112867385, 1.000000000000000000, 0.9238795325112867385, 1.000000000000000000, 0.9238795325112867385, 1.000000000000000000, 0.9238795325112867385, 1.000000000000000000, 0.9238795325112867385, 1.000000000000000000, 0.9238795325112867385, 1.000000000000000000, 0.9238795325112867385, 1.000000000000000000, 0.9238795325112867385, 1.000000000000000000, 0.9238795325112867385, 1.000000000000000000, 0.9238795325112867385, 1.000000000000000000, 0.9238795325112867385, 1.000000000000000000, 0.9238795325112867385, 1.000000000000000000, 0.9238795325112867385, 1.000000000000000000, 0.9238795325112867385, 1.000000000000000000, 0.9238795325112867385, 1.000000000000000000, 0.9238795325112867385, 1.000000000000000000, 0.9238795325112867385, 1.000000000000000000, 0.9238795325112867385, 1.000000000000000000, 0.9238795325112867385, 1.000000000000000000, 0.9238795325112867385, 1.000000000000000000, 0.9238795325112867385, 1.000000000000000000, 0.9238795325112867385, 1.000000000000000000, 0.9238795325112867385, 1.000000000000000000, 0.9238795325112867385, 1.000000000000000000, 0.9238795325112867385, 1.000000000000000000, 0.9238795325112867385, 1.000000000000000000, 0.9238795325112867385, 1.000000000000000000, 0.9238795325112867385, 1.000000000000000000, 0.9238795325112867385, 1.000000000000000000, 0.9238795325112867385, 1.000000000000000000, 0.9238795325112867385, 1.000000000000000000, 0.9238795325112867385, 1.000000000000000000, 0.9238795325112867385, 1.000000000000000000, 0.9238795325112867385, 1.000000000000000000, 0.9238795325112867385, 1.000000000000000000, 0.9238795325112867385, 1.000000000000000000, 0.9238795325112867385, 1.000000000000000000, 0.9238795325112867385, 1.000000000000000000, 0.9238795325112867385, 1.000000000000000000, 0.9238795325112867385, 1.000000000000000000, 0.9238795325112867385, 1.000000000000000000, 0.9238795325112867385, 1.000000000000000000, 0.9238795325112867385, 1.000000000000000000, 0.9238795325112867385, 1.000000000000000000, 0.9238795325112867385, 1.000000000000000000, 0.9238795325112867385, 1.000000000000000000, 0.9238795325112867385, 1.000000000000000000, 0.9238795325112867385, 1.000000000000000000, 0.9238795325112867385, 1.000000000000000000, 0.9238795325112867385, 1.000000000000000000, 0.9238795325112867385, 1.000000000000000000, 0.9238795325112867385, 1.000000000000000000, 0.9238795325112867385, 1.000000000000000000, 0.9238795325112867385, 1.000000000000000000, 0.9238795325112867385, 1.000000000000000000, 0.9238795325112867385, 1.000000000000000000, 0.9238795325112867385, 1.000000000000000000, 0.9238795325112867385, 1.000000000000000000, 0.9238795325112867385, 1.000000000000000000, 0.9238795325112867385, 1.000000000000000000, 0.9238795325112867385, 1.000000000000000000, 0.9238795325112867385, 1.000000000000000000, 0.9238795325112867385, 1.000000000000000000, 0.9238795325112867385, 1.000000000000000000, 0.9238795325112867385, 1.000000000000000000, 0.9238795325112867385, 1.000000000000000000, 0.9238795325112867385, 1.000000000000000000, 0.9238795325112867385, 1.000000000000000000, 0.9238795325112867385, 1.000000000000000000, 0.9238795325112867385, 1.000000000000000000, 0.9238795325112867385, 1.000000000000000000, 0.9238795325112867385, 1.000000000000000000, 0.9238795325112867385, 1.000000000000000000, 0.9238795325112867385, 1.000000000000000000, 0.9238795325112867385, 1.000000000000000000, 0.9238795325112867385, 1.000000000000000000, 0.9238795325112867385, 1.000000000000000000, 0.9238795325112867385, 1.000000000000000000, 0.9238795325112867385, 1.000000000000000000, 0.9238795325112867385, 1.000000000000000000, 0.9238795325112867385, 1.000000000000000000, 0.9238795325112867385, 1.000000000000000000, 0.9238795325112867385, 1.000000000000000000, 0.9238795325112867385, 1.000000000000000000, 0.9238795325112867385, 1.000000000000000000, 0.9238795325112867385, 1.000000000000000000, 0.9238795325112867385, 1.000000000000000000, 0.9238795325112867385, 1.000000000000000000, 0.9238795325112867385, 1.000000000000000000, 0.9238795325112867385, 1.000000000000000000, 0.9238795325112867385, 1.000000000000000000, 0.9238795325112867385, 1.000000000000000000, 0.9238795325112867385, 1.000000000000000000, 0.9238795325112867385, 1.000000000000000000, 0.9238795325112867385, 1.000000000000000000, 0.9238795325112867385, 1.000000000000000000, 0.9238795325112867385, 1.000000000000000000, 0.9238795325112867385, 1.000000000000000000, 0.9238795325112867385, 1.000000000000000000, 0.9238795325112867385, 1.000000000000000000, 0.9238795325112867385, 1.000000000000000000, 0.9238795325112867385, 1.000000000000000000, 0.9238795325112867385, 1.000000000000000000, 0.9238795325112867385, 1.000000000000000000, 0.9238795325112867385, 1.000000000000000000, 0.9238795325112867385, 1.000000000000000000, 0.9238795325112867385, 1.000000000000000000, 0.9238795325112867385, 1.000000000000000000, 0.9238795325112867385, 1.000000000000000000, 0.9238795325112867385, 1.000000000000000000, 0.9238795325112867385, 1.000000000000000000, 0.9238795325112867385, 1.000000000000000000, 0.9238795325112867385, 1.000000000000000000, 0.9238795325112867385, 1.000000000000000000, 0.9238795325112867385, 1.000000000000000000, 0.9238795325112867385, 1.000000000000000000, 0.9238795325112867385, 1.000000000000000000, 0.9238795325112867385, 1.000000000000000000, 0.9238795325112867385, 1.000000000000000000, 0.9238795325112867385, 1.000000000000000000, 0.9238795325112867385, 1.000000000000000000, 0.9238795325112867385, 1.000000000000000000, 0.9238795325112867385, 1.000000000000000000, 0.9238795325112867385, 1.000000000000000000, 0.9238795325112867385, 1.000000000000000000, 0.9238795325112867385, 1.000000000000000000, 0.9238795325112867385, 1.000000000000000000, 0.9238795325112867385, 1.000000000000000000, 0.9238795325112867385, 1.000000000000000000, 0.9238795325112867385, 1.000000000000000000, 0.9238795325112867385, 1.000000000000000000, 0.9238795325112867385, 1.000000000000000000, 0.9238795325112867385, 1.000000000000000000, 0.9238795325112867385, 1.000000000000000000, 0.9238795325112867385, 1.000000000000000000, 0.9238795325112867385, 1.000000000000000000, 0.9238795325112867385, 1.000000000000000000, 0.9238795325112867385, 1.000000000000000000, 0.9238795325112867385, 1.000000000000000000, 0.9238795325112867385, 1.000000000000000000, 0.9238795325112867385, 1.000000000000000000, 0.9238795325112867385, 1.000000000000000000, 0.9238795325112867385, 1.000000000000000000, 0.9238795325112867385, 1.000000000000000000, 0.9238795325112867385, 1.000000000000000000, 0.9238795325112867385, 1.000000000000000000, 0.9238795325112867385, 1.000000000000000000, 0.9238795325112867385, 1.000000000000000000, 0.9238795325112867385, 1.000000000000000000, 0.9238795325112867385, 1.000000000000000000, 0.9238795325112867385, 1.000000000000000000, 0.9238795325112867385, 1.000000000000000000, 0.9238795325112867385, 1.000000000000000000, 0.9238795325112867385, 1.000000000000000000, 0.9238795325112867385, 1.000000000000000000, 0.9238795325112867385, 1.000000000000000000, 0.9238795325112867385, 1.000000000000000000, 0.9238795325112867385, 1.000000000000000000, 0.9238795325112867385, 1.000000000000000000, 0.9238795325112867385, 1.000000000000000000, 0.9238795325112867385, 1.000000000000000000, 0.9238795325112867385, 1.000000000000000000, 0.9238795325112867385, 1.000000000000000000, 0.9238795325112867385, 1.000000000000000000, 0.9238795325112867385, 1.000000000000000000, 0.9238795325112867385, 1.000000000000000000, 0.9238795325112867385, 1.000000000000000000, 0.9238795325112867385, 1.000000000000000000, 0.9238795325112867385, 1.000000000000000000),
 ( 1.000000000000000000, 0.9238795325112867385, 1.000000000000000000, 0.9238795325112867385, 1.000000000000000000, 0.9238795325112867385, 1.000000000000000000, 0.9238795325112867385, 1.000000000000000000, 0.9238795325112867385, 1.000000000000000000, 0.9238795325112867385, 1.000000000000000000, 0.9238795325112867385, 1.000000000000000000, 0.9238795325112867385, 1.000000000000000000, 0.9238795325112867385, 1.000000000000000000, 0.9238795325112867385, 1.000000000000000000, 0.9238795325112867385, 1.000000000000000000, 0.9238795325112867385, 1.000000000000000000, 0.9238795325112867385, 1.000000000000000000, 0.9238795325112867385, 1.000000000000000000, 0.9238795325112867385, 1.000000000000000000, 0.9238795325112867385, 1.000000000000000000, 0.9238795325112867385, 1.000000000000000000, 0.9238795325112867385, 1.000000000000000000, 0.9238795325112867385, 1.000000000000000000, 0.9238795325112867385, 1.000000000000000000, 0.9238795325112867385, 1.000000000000000000, 0.9238795325112867385, 1.000000000000000000, 0.9238795325112867385, 1.000000000000000000, 0.9238795325112867385, 1.000000000000000000, 0.9238795325112867385, 1.000000000000000000, 0.9238795325112867385, 1.000000000000000000, 0.9238795325112867385, 1.000000000000000000, 0.9238795325112867385, 1.000000000000000000, 0.9238795325112867385, 1.000000000000000000, 0.9238795325112867385, 1.000000000000000000, 0.9238795325112867385, 1.000000000000000000, 0.9238795325112867385, 1.000000000000000000, 0.9238795325112867385, 1.000000000000000000, 0.9238795325112867385, 1.000000000000000000, 0.9238795325112867385, 1.000000000000000000, 0.9238795325112867385, 1.000000000000000000, 0.9238795325112867385, 1.000000000000000000, 0.9238795325112867385, 1.000000000000000000, 0.9238795325112867385, 1.000000000000000000, 0.9238795325112867385, 1.000000000000000000, 0.9238795325112867385, 1.000000000000000000, 0.9238795325112867385, 1.000000000000000000, 0.9238795325112867385, 1.000000000000000000, 0.9238795325112867385, 1.000000000000000000, 0.9238795325112867385, 1.000000000000000000, 0.9238795325112867385, 1.000000000000000000, 0.9238795325112867385, 1.000000000000000000, 0.9238795325112867385, 1.000000000000000000, 0.9238795325112867385, 1.000000000000000000, 0.9238795325112867385, 1.000000000000000000, 0.9238795325112867385, 1.000000000000000000, 0.9238795325112867385, 1.000000000000000000, 0.9238795325112867385, 1.000000000000000000, 0.9238795325112867385, 1.000000000000000000, 0.9238795325112867385, 1.000000000000000000, 0.9238795325112867385, 1.000000000000000000, 0.9238795325112867385, 1.000000000000000000, 0.9238795325112867385, 1.000000000000000000, 0.9238795325112867385, 1.000000000000000000, 0.9238795325112867385, 1.000000000000000000, 0.9238795325112867385, 1.000000000000000000, 0.9238795325112867385, 1.000000000000000000, 0.9238795325112867385, 1.000000000000000000, 0.9238795325112867385, 1.000000000000000000, 0.9238795325112867385, 1.000000000000000000, 0.9238795325112867385, 1.000000000000000000, 0.9238795325112867385, 1.000000000000000000, 0.9238795325112867385, 1.000000000000000000, 0.9238795325112867385, 1.000000000000000000, 0.9238795325112867385, 1.000000000000000000, 0.9238795325112867385, 1.000000000000000000, 0.9238795325112867385, 1.000000000000000000, 0.9238795325112867385, 1.000000000000000000, 0.9238795325112867385, 1.000000000000000000, 0.9238795325112867385, 1.000000000000000000, 0.9238795325112867385, 1.000000000000000000, 0.9238795325112867385, 1.000000000000000000, 0.9238795325112867385, 1.000000000000000000, 0.9238795325112867385, 1.000000000000000000, 0.9238795325112867385, 1.000000000000000000, 0.9238795325112867385, 1.000000000000000000, 0.9238795325112867385, 1.000000000000000000, 0.9238795325112867385, 1.000000000000000000, 0.9238795325112867385, 1.000000000000000000, 0.9238795325112867385, 1.000000000000000000, 0.9238795325112867385, 1.000000000000000000, 0.9238795325112867385, 1.000000000000000000, 0.9238795325112867385, 1.000000000000000000, 0.9238795325112867385, 1.000000000000000000, 0.9238795325112867385, 1.000000000000000000, 0.9238795325112867385, 1.000000000000000000, 0.9238795325112867385, 1.000000000000000000, 0.9238795325112867385, 1.000000000000000000, 0.9238795325112867385, 1.000000000000000000, 0.9238795325112867385, 1.000000000000000000, 0.9238795325112867385, 1.000000000000000000, 0.9238795325112867385, 1.000000000000000000, 0.9238795325112867385, 1.000000000000000000, 0.9238795325112867385, 1.000000000000000000, 0.9238795325112867385, 1.000000000000000000, 0.9238795325112867385, 1.000000000000000000, 0.9238795325112867385, 1.000000000000000000, 0.9238795325112867385, 1.000000000000000000, 0.9238795325112867385, 1.000000000000000000, 0.9238795325112867385, 1.000000000000000000, 0.9238795325112867385, 1.000000000000000000, 0.9238795325112867385, 1.000000000000000000, 0.9238795325112867385, 1.000000000000000000, 0.9238795325112867385, 1.000000000000000000, 0.9238795325112867385, 1.000000000000000000, 0.9238795325112867385, 1.000000000000000000, 0.9238795325112867385, 1.000000000000000000, 0.9238795325112867385, 1.000000000000000000, 0.9238795325112867385, 1.000000000000000000, 0.9238795325112867385, 1.000000000000000000, 0.9238795325112867385, 1.000000000000000000, 0.9238795325112867385, 1.000000000000000000, 0.9238795325112867385, 1.000000000000000000, 0.9238795325112867385, 1.000000000000000000, 0.9238795325112867385, 1.000000000000000000, 0.9238795325112867385, 1.000000000000000000, 0.9238795325112867385, 1.000000000000000000, 0.9238795325112867385, 1.000000000000000000, 0.9238795325112867385, 1.000000000000000000, 0.9238795325112867385, 1.000000000000000000, 0.9238795325112867385, 1.000000000000000000, 0.9238795325112867385, 1.000000000000000000, 0.9238795325112867385, 1.000000000000000000, 0.9238795325112867385, 1.000000000000000000, 0.9238795325112867385, 1.000000000000000000, 0.9238795325112867385, 1.000000000000000000, 0.9238795325112867385, 1.000000000000000000, 0.9238795325112867385, 1.000000000000000000, 0.9238795325112867385, 1.000000000000000000, 0.9238795325112867385, 1.000000000000000000, 0.9238795325112867385, 1.000000000000000000, 0.9238795325112867385, 1.000000000000000000, 0.9238795325112867385, 1.000000000000000000, 0.9238795325112867385, 1.000000000000000000, 0.9238795325112867385, 1.000000000000000000, 0.9238795325112867385, 1.000000000000000000, 0.9238795325112867385, 1.000000000000000000, 0.9238795325112867385, 1.000000000000000000, 0.9238795325112867385, 1.000000000000000000, 0.9238795325112867385, 1.000000000000000000, 0.9238795325112867385, 1.000000000000000000, 0.9238795325112867385, 1.000000000000000000, 0.9238795325112867385, 1.000000000000000000, 0.9238795325112867385, 1.000000000000000000, 0.9238795325112867385, 1.000000000000000000, 0.9238795325112867385, 1.000000000000000000, 0.9238795325112867385, 1.000000000000000000, 0.9238795325112867385, 1.000000000000000000, 0.9238795325112867385, 1.000000000000000000, 0.9238795325112867385, 1.000000000000000000, 0.9238795325112867385, 1.000000000000000000, 0.9238795325112867385, 1.000000000000000000, 0.9238795325112867385, 1.000000000000000000, 0.9238795325112867385, 1.000000000000000000, 0.9238795325112867385, 1.000000000000000000, 0.9238795325112867385, 1.000000000000000000, 0.9238795325112867385, 1.000000000000000000, 0.9238795325112867385, 1.000000000000000000, 0.9238795325112867385, 1.000000000000000000, 0.9238795325112867385, 1.000000000000000000, 0.9238795325112867385, 1.000000000000000000, 0.9238795325112867385, 1.000000000000000000, 0.9238795325112867385, 1.000000000000000000, 0.9238795325112867385, 1.000000000000000000, 0.9238795325112867385, 1.000000000000000000, 0.9238795325112867385, 1.000000000000000000, 0.9238795325112867385, 1.000000000000000000, 0.9238795325112867385, 1.000000000000000000, 0.9238795325112867385, 1.000000000000000000, 0.9238795325112867385, 1.000000000000000000, 0.9238795325112867385, 1.000000000000000000, 0.9238795325112867385, 1.000000000000000000, 0.9238795325112867385, 1.000000000000000000, 0.9238795325112867385, 1.000000000000000000, 0.9238795325112867385, 1.000000000000000000, 0.9238795325112867385, 1.000000000000000000, 0.9238795325112867385, 1.000000000000000000, 0.9238795325112867385, 1.000000000000000000, 0.9238795325112867385, 1.000000000000000000, 0.9238795325112867385, 1.000000000000000000, 0.9238795325112867385, 1.000000000000000000, 0.9238795325112867385, 1.000000000000000000, 0.9238795325112867385, 1.000000000000000000, 0.9238795325112867385, 1.000000000000000000, 0.9238795325112867385, 1.000000000000000000, 0.9238795325112867385, 1.000000000000000000, 0.9238795325112867385, 1.000000000000000000, 0.9238795325112867385, 1.000000000000000000, 0.9238795325112867385, 1.000000000000000000, 0.9238795325112867385, 1.000000000000000000, 0.9238795325112867385, 1.000000000000000000, 0.9238795325112867385, 1.000000000000000000, 0.9238795325112867385, 1.000000000000000000, 0.9238795325112867385, 1.000000000000000000, 0.9238795325112867385, 1.000000000000000000, 0.9238795325112867385, 1.000000000000000000, 0.9238795325112867385, 1.000000000000000000, 0.9238795325112867385, 1.000000000000000000, 0.9238795325112867385, 1.000000000000000000, 0.9238795325112867385, 1.000000000000000000, 0.9238795325112867385, 1.000000000000000000, 0.9238795325112867385, 1.000000000000000000, 0.9238795325112867385, 1.000000000000000000, 0.9238795325112867385, 1.000000000000000000, 0.9238795325112867385, 1.000000000000000000, 0.9238795325112867385, 1.000000000000000000, 0.9238795325112867385, 1.000000000000000000, 0.9238795325112867385, 1.000000000000000000, 0.9238795325112867385, 1.000000000000000000, 0.9238795325112867385, 1.000000000000000000, 0.9238795325112867385, 1.000000000000000000, 0.9238795325112867385, 1.000000000000000000, 0.9238795325112867385, 1.000000000000000000, 0.9238795325112867385, 1.000000000000000000, 0.9238795325112867385, 1.000000000000000000, 0.9238795325112867385, 1.000000000000000000, 0.9238795325112867385, 1.000000000000000000, 0.9238795325112867385, 1.000000000000000000, 0.9238795325112867385, 1.000000000000000000, 0.9238795325112867385, 1.000000000000000000, 0.9238795325112867385, 1.000000000000000000, 0.9238795325112867385, 1.000000000000000000, 0.9238795325112867385, 1.000000000000000000, 0.9238795325112867385, 1.000000000000000000, 0.9238795325112867385, 1.000000000000000000, 0.9238795325112867385, 1.000000000000000000, 0.9238795325112867385, 1.000000000000000000, 0.9238795325112867385, 1.000000000000000000, 0.9238795325112867385, 1.000000000000000000, 0.9238795325112867385, 1.000000000000000000, 0.9238795325112867385, 1.000000000000000000, 0.9238795325112867385, 1.000000000000000000, 0.9238795325112867385, 1.000000000000000000, 0.9238795325112867385, 1.000000000000000000, 0.9238795325112867385, 1.000000000000000000) ) ) 
 REPRESENTATION_ITEM ( '' )  SURFACE ( )  );
#2458=CARTESIAN_POINT ( 'NONE',  ( -58.39396692619412477, -154.6875000013656063, 2.891590998281057701 ) ) ;
#2469=CARTESIAN_POINT ( 'NONE',  ( -55.39835681537999790, -135.8750000000000284, 4.984105922594378235 ) ) ;
#2477=CARTESIAN_POINT ( 'NONE',  ( -52.80376928212989185, -141.1250000013656063, -4.297418129356378458 ) ) ;
#2479=CARTESIAN_POINT ( 'NONE',  ( -58.24261429053147765, -131.3750000027312126, -3.805975901505573855 ) ) ;
#2493=CARTESIAN_POINT ( 'NONE',  ( -54.64476657466781973, -125.8125000013655921, -4.444560631937228834 ) ) ;
#2495=CARTESIAN_POINT ( 'NONE',  ( -51.75738570946856498, -141.8750000027312126, 3.805975901505576964 ) ) ;
#2504=CARTESIAN_POINT ( 'NONE',  ( -59.44456063193725015, -134.5625000013656063, -0.3552334253322034230 ) ) ;
#2515=CARTESIAN_POINT ( 'NONE',  ( -53.51423613279429503, -129.5000000013656347, 4.591703134518082763 ) ) ;
#2539=CARTESIAN_POINT ( 'NONE',  ( -51.75738570946856498, -137.8750000027312126, 3.805975901505576964 ) ) ;
#2543=CARTESIAN_POINT ( 'NONE',  ( -59.59170313451810586, -137.5000000013656063, 1.485763867205729394 ) ) ;
#2549=CARTESIAN_POINT ( 'NONE',  ( -51.19402409849444524, -149.5000000000000284, -3.242614290531456334 ) ) ;
#2558=CARTESIAN_POINT ( 'NONE',  ( -57.19623071787016499, -154.6250000013656063, 4.297418129356382899 ) ) ;
#2559=CARTESIAN_POINT ( 'NONE',  ( -54.60164318462004474, -144.5000000027312126, -4.984105922594373794 ) ) ;
#2566=CARTESIAN_POINT ( 'NONE',  ( -53.51423613279429503, -136.2500000013656063, 4.591703134518082763 ) ) ;
#2581=CARTESIAN_POINT ( 'NONE',  ( -50.40829686548195099, -146.0000000013656347, -1.485763867205728284 ) ) ;
#2624=CARTESIAN_POINT ( 'NONE',  ( -57.89159099828107458, -130.9375000013656063, -3.393966926194107447 ) ) ;
#2635=ORIENTED_EDGE ( 'NONE', *, *, #62620, .F. ) ;
#2640=CARTESIAN_POINT ( 'NONE',  ( -58.24261429053147765, -148.3750000027312126, -3.805975901505573855 ) ) ;
#2645=VERTEX_POINT ( 'NONE', #57400 ) ;
#2664=CARTESIAN_POINT ( 'NONE',  ( -58.39396692619412477, -140.6875000013656063, 2.891590998281057701 ) ) ;
#2671=ORIENTED_EDGE ( 'NONE', *, *, #9855, .T. ) ;
#2696=EDGE_CURVE ( 'NONE', #42590, #21128, #32721, .T. ) ;
#2697=CARTESIAN_POINT ( 'NONE',  ( -51.60603307380591787, -149.1875000013656063, -2.891590998281053704 ) ) ;
#2702=ORIENTED_EDGE ( 'NONE', *, *, #18187, .T. ) ;
#2708=( BOUNDED_CURVE ( )  B_SPLINE_CURVE ( 2, ( #53966, #14408, #34030, #29830, #49462, #25019, #53651, #49138, #58791 ),
 .UNSPECIFIED., .F., .F. ) 
 B_SPLINE_CURVE_WITH_KNOTS ( ( 3, 2, 2, 2, 3 ),
 ( 0.2416666666666668628, 0.2458333333333335147, 0.2500000000000002220, 0.2541666666666668739, 0.2583333333333335813 ),
 .UNSPECIFIED. ) 
 CURVE ( )  GEOMETRIC_REPRESENTATION_ITEM ( )  RATIONAL_B_SPLINE_CURVE ( ( 0.9999999999999964473, 0.9238795325112902912, 1.000000000000000000, 0.9238795325112867385, 1.000000000000000000, 0.9238795325112867385, 1.000000000000000000, 0.9238795325112826307, 1.000000000000003997 ) ) 
 REPRESENTATION_ITEM ( '' )  );
#2709=CARTESIAN_POINT ( 'NONE',  ( -54.60164318462004474, -127.3750000000000142, -4.984105922594373794 ) ) ;
#2718=CARTESIAN_POINT ( 'NONE',  ( -56.48576386720575471, -147.7500000013655779, -4.591703134518078322 ) ) ;
#2725=AXIS2_PLACEMENT_3D ( 'NONE', #11968, #7798, #51231 ) ;
#2743=CARTESIAN_POINT ( 'NONE',  ( -52.10840900171896806, -152.4375000013656063, 3.393966926194110556 ) ) ;
#2783=CARTESIAN_POINT ( 'NONE',  ( -56.66612745406270335, -136.3125000000000000, -5.149110718188516067 ) ) ;
#2789=ADVANCED_FACE ( 'NONE', ( #54460 ), #39016, .F. ) ;
#2794=CARTESIAN_POINT ( 'NONE',  ( -53.51423613279429503, -140.5000000013655779, 4.591703134518083651 ) ) ;
#2796=CARTESIAN_POINT ( 'NONE',  ( -53.33387254593733928, -129.9375000027312126, 5.149110718188519620 ) ) ;
#2809=CARTESIAN_POINT ( 'NONE',  ( -54.64476657466781973, -124.8125000013655921, -4.444560631937228834 ) ) ;
#2822=VECTOR ( 'NONE', #33796, 1000.000000000000000 ) ;
#2823=CARTESIAN_POINT ( 'NONE',  ( -55.35523342533222291, -135.3125000013656063, 4.444560631937231499 ) ) ;
#2833=CARTESIAN_POINT ( 'NONE',  ( -55.35523342533222291, -126.5625000013655921, 4.444560631937231499 ) ) ;
#2840=CARTESIAN_POINT ( 'NONE',  ( -54.60164318462004474, -137.5000000027312126, -4.984105922594373794 ) ) ;
#2856=CARTESIAN_POINT ( 'NONE',  ( -59.44456063193725015, -153.8125000013656347, -0.3552334253322034230 ) ) ;
#2860=CARTESIAN_POINT ( 'NONE',  ( -50.55543936806279248, -138.0625000013656063, 0.3552334253322060320 ) ) ;
#2868=CARTESIAN_POINT ( 'NONE',  ( -51.19402409849444524, -148.5000000000000284, -3.242614290531456334 ) ) ;
#2875=SURFACE_SIDE_STYLE ('',( #16706 ) ) ;
#2881=CARTESIAN_POINT ( 'NONE',  ( -58.39396692619412477, -153.6875000013656063, 2.891590998281057701 ) ) ;
#2882=CARTESIAN_POINT ( 'NONE',  ( -52.53715891517739323, -141.5625000027312126, -4.819101127000233298 ) ) ;
#2891=CARTESIAN_POINT ( 'NONE',  ( -50.70258187064364108, -137.1250000013655779, 2.196230717870141014 ) ) ;
#2906=CARTESIAN_POINT ( 'NONE',  ( -50.55543936806279248, -147.0625000013656063, 0.3552334253322060320 ) ) ;
#2914=( BOUNDED_CURVE ( )  B_SPLINE_CURVE ( 2, ( #20101, #5316, #49689, #59673, #5635, #48416, #53876, #63225, #24933 ),
 .UNSPECIFIED., .F., .F. ) 
 B_SPLINE_CURVE_WITH_KNOTS ( ( 3, 2, 2, 2, 3 ),
 ( 0.2916666666666669072, 0.2958333333333335591, 0.3000000000000002665, 0.3041666666666669183, 0.3083333333333336257 ),
 .UNSPECIFIED. ) 
 CURVE ( )  GEOMETRIC_REPRESENTATION_ITEM ( )  RATIONAL_B_SPLINE_CURVE ( ( 0.9999999999999958922, 0.9238795325112908463, 1.000000000000000000, 0.9238795325112867385, 1.000000000000000000, 0.9238795325112867385, 1.000000000000000000, 0.9238795325112816315, 1.000000000000005107 ) ) 
 REPRESENTATION_ITEM ( '' )  );
#2948=CARTESIAN_POINT ( 'NONE',  ( -56.48576386720575471, -131.0000000013656063, -4.591703134518078322 ) ) ;
#2955=FACE_OUTER_BOUND ( 'NONE', #59978, .T. ) ;
#2966=CARTESIAN_POINT ( 'NONE',  ( -52.53715891517739323, -148.5625000027311842, -4.819101127000233298 ) ) ;
#2976=CARTESIAN_POINT ( 'NONE',  ( -55.00000000000002132, -155.0000000000000284, 1.734723475976807094E-15 ) ) ;
#2979=CARTESIAN_POINT ( 'NONE',  ( -51.75738570946856498, -138.8750000027312126, 3.805975901505576964 ) ) ;
#2981=CYLINDRICAL_SURFACE ( 'NONE', #2725, 5.000000000000000000 ) ;
#2991=CARTESIAN_POINT ( 'NONE',  ( -57.89159099828107458, -136.9375000013655779, -3.393966926194107447 ) ) ;
#3023=CARTESIAN_POINT ( 'NONE',  ( -50.40829686548195099, -142.2500000013656063, -1.485763867205728284 ) ) ;
#3033=CARTESIAN_POINT ( 'NONE',  ( -51.75738570946856498, -126.7500000000000284, 3.805975901505576964 ) ) ;
#3041=CARTESIAN_POINT ( 'NONE',  ( -54.64476657466781973, -150.8125000013656063, -4.444560631937228834 ) ) ;
#3061=ORIENTED_EDGE ( 'NONE', *, *, #32988, .F. ) ;
#3066=CARTESIAN_POINT ( 'NONE',  ( -50.40829686548195099, -150.2500000013656063, -1.485763867205728284 ) ) ;
#3089=ORIENTED_EDGE ( 'NONE', *, *, #49591, .T. ) ;
#3104=CARTESIAN_POINT ( 'NONE',  ( -56.66612745406270335, -137.3125000000000284, -5.149110718188516067 ) ) ;
#3111=EDGE_LOOP ( 'NONE', ( #55303, #24448, #48634, #52654 ) ) ;
#3112=CARTESIAN_POINT ( 'NONE',  ( -58.39396692619412477, -137.6875000013656063, 2.891590998281057701 ) ) ;
#3114=CARTESIAN_POINT ( 'NONE',  ( -52.53715891517739323, -131.5625000027312410, -4.819101127000233298 ) ) ;
#3125=CARTESIAN_POINT ( 'NONE',  ( -52.10840900171896806, -126.1875000013656063, 3.393966926194110556 ) ) ;
#3128=AXIS2_PLACEMENT_3D ( 'NONE', #42970, #38155, #52942 ) ;
#3138=CARTESIAN_POINT ( 'NONE',  ( -52.10840900171896806, -133.1875000013656063, 3.393966926194110556 ) ) ;
#3149=CARTESIAN_POINT ( 'NONE',  ( -59.59170313451811296, -128.7500000013656063, 1.485763867205729394 ) ) ;
#3157=CARTESIAN_POINT ( 'NONE',  ( -49.85088928181150436, -137.6875000027311842, -1.666127454062680480 ) ) ;
#3162=ORIENTED_EDGE ( 'NONE', *, *, #43472, .F. ) ;
#3163=ADVANCED_FACE ( 'NONE', ( #21952 ), #2981, .F. ) ;
#3173=CARTESIAN_POINT ( 'NONE',  ( -50.55543936806279248, -154.3125000013656347, 0.3552334253322060320 ) ) ;
#3177=CARTESIAN_POINT ( 'NONE',  ( -55.35523342533222291, -139.3125000013656063, 4.444560631937231499 ) ) ;
#3184=CARTESIAN_POINT ( 'NONE',  ( -53.33387254593733928, -150.8125000000000000, 5.149110718188519620 ) ) ;
#3193=CARTESIAN_POINT ( 'NONE',  ( -58.24261429053147765, -149.3750000027312126, -3.805975901505573855 ) ) ;
#3195=CARTESIAN_POINT ( 'NONE',  ( -50.70258187064364108, -151.3750000013656063, 2.196230717870141014 ) ) ;
#3196=CARTESIAN_POINT ( 'NONE',  ( -59.81910112700025905, -143.3125000027312126, -2.462841084822630311 ) ) ;
#3203=CARTESIAN_POINT ( 'NONE',  ( -57.89159099828107458, -136.6875000013656063, -3.393966926194107447 ) ) ;
#3218=CARTESIAN_POINT ( 'NONE',  ( -52.10840900171896806, -145.1875000013656063, 3.393966926194110556 ) ) ;
#3234=CARTESIAN_POINT ( 'NONE',  ( -59.98410592259440222, -149.1250000000000284, -0.3983568153799752487 ) ) ;
#3257=ORIENTED_EDGE ( 'NONE', *, *, #9421, .F. ) ;
#3266=CARTESIAN_POINT ( 'NONE',  ( -53.51423613279429503, -130.5000000013656063, 4.591703134518082763 ) ) ;
#3281=CARTESIAN_POINT ( 'NONE',  ( -51.19402409849444524, -148.6250000027312126, -3.242614290531456334 ) ) ;
#3291=DIRECTION ( 'NONE',  ( 0.000000000000000000, 1.000000000000000000, 0.000000000000000000 ) ) ;
#3305=CARTESIAN_POINT ( 'NONE',  ( -52.10840900171896806, -135.4375000013656063, 3.393966926194110556 ) ) ;
#3307=CARTESIAN_POINT ( 'NONE',  ( -56.66612745406286678, -145.3125000000000284, -5.149110718188528502 ) ) ;
#3329=DIRECTION ( 'NONE',  ( -0.6485228581062915110, 0.000000000000000000, -0.7611951803011149931 ) ) ;
#3338=CARTESIAN_POINT ( 'NONE',  ( -52.10840900171896806, -144.4375000013656063, 3.393966926194110556 ) ) ;
#3347=CARTESIAN_POINT ( 'NONE',  ( -54.60164318462004474, -125.3750000000000142, -4.984105922594373794 ) ) ;
#3354=CARTESIAN_POINT ( 'NONE',  ( -57.89159099828107458, -148.6875000013656063, -3.393966926194107447 ) ) ;
#3369=CARTESIAN_POINT ( 'NONE',  ( -52.53715891517739323, -146.4375000000000000, -4.819101127000233298 ) ) ;
#3380=CARTESIAN_POINT ( 'NONE',  ( -51.60603307380591787, -147.1875000013656063, -2.891590998281053704 ) ) ;
#3385=CARTESIAN_POINT ( 'NONE',  ( -51.75738570946856498, -136.7500000000000284, 3.805975901505576964 ) ) ;
#3397=CARTESIAN_POINT ( 'NONE',  ( -50.01589407740564042, -152.6250000000000284, 0.3983568153799778022 ) ) ;
#3415=CARTESIAN_POINT ( 'NONE',  ( -50.01589407740564042, -136.6250000000000284, 0.3983568153799778022 ) ) ;
#3418=CARTESIAN_POINT ( 'NONE',  ( -50.01589407740564042, -140.6250000000000284, 0.3983568153799778022 ) ) ;
#3423=ORIENTED_EDGE ( 'NONE', *, *, #31816, .F. ) ;
#3425=CARTESIAN_POINT ( 'NONE',  ( -56.48576386720575471, -138.0000000013656063, -4.591703134518078322 ) ) ;
#3427=CARTESIAN_POINT ( 'NONE',  ( -58.80597590150559739, -130.1250000027312126, 3.242614290531460330 ) ) ;
#3443=ORIENTED_EDGE ( 'NONE', *, *, #61012, .T. ) ;
#3450=CARTESIAN_POINT ( 'NONE',  ( -58.39396692619412477, -129.4375000013656063, 2.891590998281057701 ) ) ;
#3461=CARTESIAN_POINT ( 'NONE',  ( -57.19623071787017210, -129.6250000013655779, 4.297418129356382899 ) ) ;
#3492=CARTESIAN_POINT ( 'NONE',  ( -58.24261429053147765, -150.2500000000000284, -3.805975901505573855 ) ) ;
#3501=CARTESIAN_POINT ( 'NONE',  ( -59.59170313451810586, -150.7500000013655779, 1.485763867205729394 ) ) ;
#3502=CARTESIAN_POINT ( 'NONE',  ( -60.14911071818854538, -144.1875000027312410, 1.666127454062681368 ) ) ;
#3512=CARTESIAN_POINT ( 'NONE',  ( -52.80376928212989185, -135.8750000013655779, -4.297418129356379346 ) ) ;
#3523=FACE_OUTER_BOUND ( 'NONE', #29654, .T. ) ;
#3528=CARTESIAN_POINT ( 'NONE',  ( -50.55543936806279248, -144.0625000013656063, 0.3552334253322060320 ) ) ;
#3541=( BOUNDED_CURVE ( )  B_SPLINE_CURVE ( 2, ( #44303, #29187, #48814, #267, #63628, #38527, #9893, #19548, #58155 ),
 .UNSPECIFIED., .F., .F. ) 
 B_SPLINE_CURVE_WITH_KNOTS ( ( 3, 2, 2, 2, 3 ),
 ( 0.04166666666666670599, 0.04583333333333337173, 0.05000000000000004441, 0.05416666666666671709, 0.05833333333333338283 ),
 .UNSPECIFIED. ) 
 CURVE ( )  GEOMETRIC_REPRESENTATION_ITEM ( )  RATIONAL_B_SPLINE_CURVE ( ( 0.9999999999999992228, 0.9238795325112875156, 1.000000000000000000, 0.9238795325112867385, 1.000000000000000000, 0.9238795325112867385, 1.000000000000000000, 0.9238795325112858503, 1.000000000000000888 ) ) 
 REPRESENTATION_ITEM ( '' )  );
#3571=CARTESIAN_POINT ( 'NONE',  ( -59.44456063193725015, -130.8125000013656063, -0.3552334253322034230 ) ) ;
#3581=CARTESIAN_POINT ( 'NONE',  ( -51.75738570946856498, -152.8750000027312126, 3.805975901505576964 ) ) ;
#3616=CARTESIAN_POINT ( 'NONE',  ( -57.19623071787017210, -137.6250000013655779, 4.297418129356382899 ) ) ;
#3617=CARTESIAN_POINT ( 'NONE',  ( -51.75738570946856498, -155.0000000000000284, 3.805975901505577408 ) ) ;
#3646=CARTESIAN_POINT ( 'NONE',  ( -55.35523342533222291, -143.5625000013656063, 4.444560631937231499 ) ) ;
#3667=CARTESIAN_POINT ( 'NONE',  ( -59.59170313451811296, -146.5000000013656347, 1.485763867205729394 ) ) ;
#3679=CARTESIAN_POINT ( 'NONE',  ( -49.85088928181150436, -142.6875000027312126, -1.666127454062680480 ) ) ;
#3686=CARTESIAN_POINT ( 'NONE',  ( -58.80597590150559739, -140.1250000027312126, 3.242614290531460330 ) ) ;
#3694=CARTESIAN_POINT ( 'NONE',  ( -52.10840900171896806, -147.4375000013656063, 3.393966926194110556 ) ) ;
#3700=CARTESIAN_POINT ( 'NONE',  ( -57.46284108482265651, -147.9375000000000284, 4.819101127000238627 ) ) ;
#3729=CARTESIAN_POINT ( 'NONE',  ( -49.85088928181150436, -134.5625000000000568, -1.666127454062680702 ) ) ;
#3731=ORIENTED_EDGE ( 'NONE', *, *, #30650, .F. ) ;
#3738=CARTESIAN_POINT ( 'NONE',  ( -52.80376928212989185, -138.1250000013656063, -4.297418129356378458 ) ) ;
#3740=CARTESIAN_POINT ( 'NONE',  ( -55.39835681537999790, -128.0000000027312126, 4.984105922594378235 ) ) ;
#3748=DIRECTION ( 'NONE',  ( 0.000000000000000000, 1.000000000000000000, 0.000000000000000000 ) ) ;
#3752=CARTESIAN_POINT ( 'NONE',  ( -51.60603307380591787, -125.9375000013656063, -2.891590998281053704 ) ) ;
#3763=CARTESIAN_POINT ( 'NONE',  ( -55.35523342533222291, -128.3125000013656063, 4.444560631937231499 ) ) ;
#3798=CARTESIAN_POINT ( 'NONE',  ( -57.19623071787017210, -150.6250000013656063, 4.297418129356382899 ) ) ;
#3805=VERTEX_POINT ( 'NONE', #8356 ) ;
#3806=CARTESIAN_POINT ( 'NONE',  ( -52.53715891517739323, -150.4375000000000000, -4.819101127000233298 ) ) ;
#3816=CARTESIAN_POINT ( 'NONE',  ( -56.48576386720575471, -149.0000000013656063, -4.591703134518078322 ) ) ;
#3817=CARTESIAN_POINT ( 'NONE',  ( -57.46284108482265651, -137.0625000027312126, 4.819101127000239515 ) ) ;
#3826=CARTESIAN_POINT ( 'NONE',  ( -57.19623071787017210, -138.3750000013656063, 4.297418129356382899 ) ) ;
#3842=CARTESIAN_POINT ( 'NONE',  ( -57.19623071787017210, -140.3750000013656063, 4.297418129356382899 ) ) ;
#3874=EDGE_LOOP ( 'NONE', ( #21814, #9313, #31557, #7235 ) ) ;
#3875=CARTESIAN_POINT ( 'NONE',  ( -55.35523342533222291, -153.3125000013656063, 4.444560631937231499 ) ) ;
#3882=CARTESIAN_POINT ( 'NONE',  ( -52.80376928212989185, -132.1250000013656347, -4.297418129356379346 ) ) ;
#3895=ORIENTED_EDGE ( 'NONE', *, *, #27956, .F. ) ;
#3896=LINE ( 'NONE', #58858, #7240 ) ;
#3899=CARTESIAN_POINT ( 'NONE',  ( -58.24261429053147765, -150.3750000027312126, -3.805975901505573855 ) ) ;
#3913=CARTESIAN_POINT ( 'NONE',  ( -55.35523342533222291, -152.3125000013656063, 4.444560631937231499 ) ) ;
#3928=CARTESIAN_POINT ( 'NONE',  ( -55.35523342533222291, -136.5625000013656063, 4.444560631937231499 ) ) ;
#3960=CARTESIAN_POINT ( 'NONE',  ( -51.60603307380591787, -145.1875000013656063, -2.891590998281053704 ) ) ;
#3970=CARTESIAN_POINT ( 'NONE',  ( -58.24261429053147765, -143.3750000027312126, -3.805975901505573855 ) ) ;
#3977=CARTESIAN_POINT ( 'NONE',  ( -58.39396692619412477, -145.4375000013656063, 2.891590998281057701 ) ) ;
#3995=CARTESIAN_POINT ( 'NONE',  ( -59.98410592259440222, -140.2500000027312126, -0.3983568153799752487 ) ) ;
#4003=CARTESIAN_POINT ( 'NONE',  ( -55.35523342533222291, -149.5625000013656063, 4.444560631937231499 ) ) ;
#4029=CARTESIAN_POINT ( 'NONE',  ( -50.01589407740564042, -135.6250000000000284, 0.3983568153799778022 ) ) ;
#4044=CARTESIAN_POINT ( 'NONE',  ( -54.60164318462004474, -132.3750000000000284, -4.984105922594373794 ) ) ;
#4045=VECTOR ( 'NONE', #49167, 1000.000000000000000 ) ;
#4052=CARTESIAN_POINT ( 'NONE',  ( -53.51423613279429503, -137.5000000013656063, 4.591703134518083651 ) ) ;
#4054=CARTESIAN_POINT ( 'NONE',  ( -57.46284108482265651, -127.0625000027312410, 4.819101127000239515 ) ) ;
#4077=CARTESIAN_POINT ( 'NONE',  ( -55.35523342533222291, -131.3125000013656063, 4.444560631937231499 ) ) ;
#4078=CARTESIAN_POINT ( 'NONE',  ( -59.29741812935640155, -147.6250000013655779, -2.196230717870135685 ) ) ;
#4086=VERTEX_POINT ( 'NONE', #53998 ) ;
#4089=CARTESIAN_POINT ( 'NONE',  ( -59.44456063193725015, -124.8125000013655921, -0.3552334253322034230 ) ) ;
#4090=DIRECTION ( 'NONE',  ( 0.000000000000000000, 1.000000000000000000, 0.000000000000000000 ) ) ;
#4097=CARTESIAN_POINT ( 'NONE',  ( -51.19402409849444524, -137.6250000027312410, -3.242614290531456334 ) ) ;
#4105=FACE_BOUND ( 'NONE', #26594, .T. ) ;
#4113=CARTESIAN_POINT ( 'NONE',  ( -52.80376928212989185, -151.1250000013655779, -4.297418129356379346 ) ) ;
#4117=CARTESIAN_POINT ( 'NONE',  ( -50.55543936806279248, -135.0625000013656063, 0.3552334253322060320 ) ) ;
#4122=CARTESIAN_POINT ( 'NONE',  ( -58.80597590150559739, -146.0000000000000284, 3.242614290531460330 ) ) ;
#4125=ORIENTED_EDGE ( 'NONE', *, *, #22819, .T. ) ;
#4131=CARTESIAN_POINT ( 'NONE',  ( -52.80376928212989185, -152.1250000013656063, -4.297418129356378458 ) ) ;
#4132=CARTESIAN_POINT ( 'NONE',  ( -51.75738570946856498, -136.8750000027312126, 3.805975901505576964 ) ) ;
#4134=CARTESIAN_POINT ( 'NONE',  ( -55.00000000000002132, -155.0000000000000284, 1.734723475976807094E-15 ) ) ;
#4141=CARTESIAN_POINT ( 'NONE',  ( -55.35523342533222291, -133.3125000013656063, 4.444560631937231499 ) ) ;
#4157=CARTESIAN_POINT ( 'NONE',  ( -54.64476657466781973, -139.8125000013656063, -4.444560631937228834 ) ) ;
#4191=CARTESIAN_POINT ( 'NONE',  ( -52.10840900171896806, -153.1875000013656063, 3.393966926194110556 ) ) ;
#4198=CARTESIAN_POINT ( 'NONE',  ( -59.44456063193725015, -125.8125000013655921, -0.3552334253322034230 ) ) ;
#4204=DIRECTION ( 'NONE',  ( -0.6485228581062915110, 0.000000000000000000, -0.7611951803011149931 ) ) ;
#4207=CARTESIAN_POINT ( 'NONE',  ( -54.60164318462004474, -150.5000000027312126, -4.984105922594373794 ) ) ;
#4225=VECTOR ( 'NONE', #31624, 1000.000000000000000 ) ;
#4226=LINE ( 'NONE', #49225, #63324 ) ;
#4227=CARTESIAN_POINT ( 'NONE',  ( -50.40829686548195099, -154.0000000013655779, -1.485763867205728284 ) ) ;
#4237=CARTESIAN_POINT ( 'NONE',  ( -56.66612745406288099, -142.3125000000000000, -5.149110718188529390 ) ) ;
#4240=CARTESIAN_POINT ( 'NONE',  ( -52.10840900171896806, -137.4375000013656063, 3.393966926194110556 ) ) ;
#4252=LINE ( 'NONE', #33520, #41171 ) ;
#4268=CARTESIAN_POINT ( 'NONE',  ( -52.80376928212989185, -144.1250000013656063, -4.297418129356379346 ) ) ;
#4277=DIRECTION ( 'NONE',  ( 0.000000000000000000, 1.000000000000000000, 0.000000000000000000 ) ) ;
#4285=CARTESIAN_POINT ( 'NONE',  ( -57.19623071787017210, -146.3750000013655779, 4.297418129356382899 ) ) ;
#4297=CARTESIAN_POINT ( 'NONE',  ( -50.01589407740564042, -142.7500000027312126, 0.3983568153799778022 ) ) ;
#4309=CARTESIAN_POINT ( 'NONE',  ( -59.29741812935640155, -146.8750000013656063, -2.196230717870135685 ) ) ;
#4325=DIRECTION ( 'NONE',  ( 0.8660254037844385966, 0.000000000000000000, 0.4999999999999999445 ) ) ;
#4344=CARTESIAN_POINT ( 'NONE',  ( -53.33387254593733928, -131.8125000000000284, 5.149110718188519620 ) ) ;
#4355=CARTESIAN_POINT ( 'NONE',  ( -54.60164318462004474, -128.5000000027312126, -4.984105922594373794 ) ) ;
#4364=DIRECTION ( 'NONE',  ( 0.000000000000000000, 1.000000000000000000, 0.000000000000000000 ) ) ;
#4368=ADVANCED_FACE ( 'NONE', ( #10568 ), #5753, .F. ) ;
#4380=CARTESIAN_POINT ( 'NONE',  ( -59.44456063193725015, -129.5625000013656063, -0.3552334253322034230 ) ) ;
#4381=CARTESIAN_POINT ( 'NONE',  ( -50.40829686548195099, -147.0000000013656063, -1.485763867205728284 ) ) ;
#4391=CARTESIAN_POINT ( 'NONE',  ( -56.48576386720575471, -126.0000000013656063, -4.591703134518078322 ) ) ;
#4402=ORIENTED_EDGE ( 'NONE', *, *, #62174, .F. ) ;
#4411=CARTESIAN_POINT ( 'NONE',  ( -57.89159099828107458, -149.9375000013656063, -3.393966926194107447 ) ) ;
#4421=CARTESIAN_POINT ( 'NONE',  ( -57.46284108482265651, -146.9375000000000284, 4.819101127000239515 ) ) ;
#4431=CARTESIAN_POINT ( 'NONE',  ( -50.70258187064364108, -150.3750000013656063, 2.196230717870141014 ) ) ;
#4432=CARTESIAN_POINT ( 'NONE',  ( -51.19402409849444524, -138.6250000027312410, -3.242614290531456334 ) ) ;
#4439=CARTESIAN_POINT ( 'NONE',  ( -55.00000000000001421, -155.0000000000000284, 8.082903768654762899 ) ) ;
#4440=CARTESIAN_POINT ( 'NONE',  ( -50.55543936806279248, -131.0625000013656063, 0.3552334253322060320 ) ) ;
#4458=CARTESIAN_POINT ( 'NONE',  ( -55.35523342533222291, -141.3125000013656063, 4.444560631937231499 ) ) ;
#4465=ORIENTED_EDGE ( 'NONE', *, *, #63072, .T. ) ;
#4490=CARTESIAN_POINT ( 'NONE',  ( -50.55543936806279248, -152.0625000013656063, 0.3552334253322060320 ) ) ;
#4497=CARTESIAN_POINT ( 'NONE',  ( -50.40829686548195099, -125.2500000013656347, -1.485763867205728284 ) ) ;
#4505=CARTESIAN_POINT ( 'NONE',  ( -57.46284108482265651, -142.9375000000000000, 4.819101127000238627 ) ) ;
#4509=CARTESIAN_POINT ( 'NONE',  ( -52.53715891517739323, -151.5625000027312126, -4.819101127000233298 ) ) ;
#4514=CYLINDRICAL_SURFACE ( 'NONE', #46662, 5.000000000000000000 ) ;
#4527=CARTESIAN_POINT ( 'NONE',  ( -50.70258187064364108, -154.1250000013656347, 2.196230717870141014 ) ) ;
#4541=CARTESIAN_POINT ( 'NONE',  ( -53.51423613279429503, -131.5000000013656347, 4.591703134518082763 ) ) ;
#4543=DIRECTION ( 'NONE',  ( -0.6485228581062915110, 0.000000000000000000, -0.7611951803011149931 ) ) ;
#4570=CARTESIAN_POINT ( 'NONE',  ( -54.64476657466781973, -141.0625000013656063, -4.444560631937228834 ) ) ;
#4590=CARTESIAN_POINT ( 'NONE',  ( -57.89159099828107458, -144.6875000013656063, -3.393966926194107447 ) ) ;
#4613=CARTESIAN_POINT ( 'NONE',  ( -57.89159099828107458, -146.9375000013656063, -3.393966926194107447 ) ) ;
#4622=ORIENTED_EDGE ( 'NONE', *, *, #18187, .F. ) ;
#4630=LINE ( 'NONE', #19429, #48024 ) ;
#4641=( BOUNDED_CURVE ( )  B_SPLINE_CURVE ( 2, ( #31113, #51383, #56204, #45591, #21476, #6679, #36266, #16963, #2495 ),
 .UNSPECIFIED., .F., .F. ) 
 B_SPLINE_CURVE_WITH_KNOTS ( ( 3, 2, 2, 2, 3 ),
 ( 0.3916666666666669960, 0.3958333333333336479, 0.4000000000000003553, 0.4041666666666670071, 0.4083333333333336590 ),
 .UNSPECIFIED. ) 
 CURVE ( )  GEOMETRIC_REPRESENTATION_ITEM ( )  RATIONAL_B_SPLINE_CURVE ( ( 0.9999999999999938938, 0.9238795325112928447, 1.000000000000000000, 0.9238795325112867385, 1.000000000000000000, 0.9238795325112867385, 1.000000000000000000, 0.9238795325112806323, 1.000000000000005995 ) ) 
 REPRESENTATION_ITEM ( '' )  );
#4653=CARTESIAN_POINT ( 'NONE',  ( -50.01589407740564042, -131.6250000000000284, 0.3983568153799778022 ) ) ;
#4656=VERTEX_POINT ( 'NONE', #47828 ) ;
#4660=CARTESIAN_POINT ( 'NONE',  ( -51.75738570946856498, -155.0000000000000284, 3.805975901505577408 ) ) ;
#4663=CARTESIAN_POINT ( 'NONE',  ( -51.19402409849444524, -125.6250000027312126, -3.242614290531456334 ) ) ;
#4679=ORIENTED_EDGE ( 'NONE', *, *, #8923, .F. ) ;
#4687=CARTESIAN_POINT ( 'NONE',  ( -53.51423613279429503, -128.2500000013656063, 4.591703134518082763 ) ) ;
#4688=CARTESIAN_POINT ( 'NONE',  ( -50.55543936806279248, -145.0625000013656063, 0.3552334253322060320 ) ) ;
#4716=( BOUNDED_CURVE ( )  B_SPLINE_CURVE ( 2, ( #51475, #50833, #56300, #27648, #22842, #46640, #31843, #27333, #2280 ),
 .UNSPECIFIED., .F., .F. ) 
 B_SPLINE_CURVE_WITH_KNOTS ( ( 3, 2, 2, 2, 3 ),
 ( 0.4083333333333336590, 0.4125000000000003109, 0.4166666666666670182, 0.4208333333333336701, 0.4250000000000003220 ),
 .UNSPECIFIED. ) 
 CURVE ( )  GEOMETRIC_REPRESENTATION_ITEM ( )  RATIONAL_B_SPLINE_CURVE ( ( 0.9999999999999938938, 0.9238795325112928447, 1.000000000000000000, 0.9238795325112867385, 1.000000000000000000, 0.9238795325112867385, 1.000000000000000000, 0.9238795325112806323, 1.000000000000005995 ) ) 
 REPRESENTATION_ITEM ( '' )  );
#4723=CARTESIAN_POINT ( 'NONE',  ( -50.70258187064364108, -151.3750000013656063, 2.196230717870141014 ) ) ;
#4734=CARTESIAN_POINT ( 'NONE',  ( -58.80597590150559739, -147.0000000000000284, 3.242614290531460330 ) ) ;
#4740=CARTESIAN_POINT ( 'NONE',  ( -58.80597590150559739, -135.1250000027312410, 3.242614290531460330 ) ) ;
#4742=CARTESIAN_POINT ( 'NONE',  ( -53.51423613279429503, -144.5000000013656063, 4.591703134518083651 ) ) ;
#4743=CARTESIAN_POINT ( 'NONE',  ( -60.14911071818854538, -140.1875000027312126, 1.666127454062681368 ) ) ;
#4753=CARTESIAN_POINT ( 'NONE',  ( -59.59170313451811296, -132.5000000013656063, 1.485763867205729394 ) ) ;
#4770=CARTESIAN_POINT ( 'NONE',  ( -53.51423613279429503, -141.2500000013656347, 4.591703134518082763 ) ) ;
#4774=CARTESIAN_POINT ( 'NONE',  ( -56.66612745406286678, -144.3125000000000000, -5.149110718188528502 ) ) ;
#4776=EDGE_LOOP ( 'NONE', ( #31730, #57028, #46594, #62025 ) ) ;
#4806=CARTESIAN_POINT ( 'NONE',  ( -50.40829686548195099, -153.0000000013656063, -1.485763867205728284 ) ) ;
#4811=CARTESIAN_POINT ( 'NONE',  ( -50.01589407740564042, -149.7500000027312126, 0.3983568153799778022 ) ) ;
#4815=CARTESIAN_POINT ( 'NONE',  ( -59.44456063193725015, -126.8125000013655921, -0.3552334253322034230 ) ) ;
#4820=CARTESIAN_POINT ( 'NONE',  ( -52.53715891517739323, -136.5625000027311842, -4.819101127000233298 ) ) ;
#4826=CARTESIAN_POINT ( 'NONE',  ( -59.81910112700025905, -152.3125000027312410, -2.462841084822630311 ) ) ;
#4840=LINE ( 'NONE', #59199, #11013 ) ;
#4863=AXIS2_PLACEMENT_3D ( 'NONE', #49467, #40127, #50432 ) ;
#4866=CARTESIAN_POINT ( 'NONE',  ( -56.66612745406274598, -151.4375000027312126, -5.149110718188520508 ) ) ;
#4892=CARTESIAN_POINT ( 'NONE',  ( -56.48576386720575471, -140.0000000013656063, -4.591703134518078322 ) ) ;
#4900=CARTESIAN_POINT ( 'NONE',  ( -49.85088928181150436, -150.5625000000000284, -1.666127454062680480 ) ) ;
#4913=CARTESIAN_POINT ( 'NONE',  ( -51.60603307380591787, -142.9375000013656063, -2.891590998281053704 ) ) ;
#4937=CARTESIAN_POINT ( 'NONE',  ( -50.70258187064364108, -144.3750000013656063, 2.196230717870141014 ) ) ;
#4975=CARTESIAN_POINT ( 'NONE',  ( -49.85088928181150436, -135.5625000000000284, -1.666127454062680702 ) ) ;
#4984=CARTESIAN_POINT ( 'NONE',  ( -59.81910112700025905, -126.3125000027312268, -2.462841084822630311 ) ) ;
#4994=B_SPLINE_CURVE_WITH_KNOTS ( 'NONE', 3,
 ( #55712, #30933, #50559, #60223, #11625, #44764, #20979, #36082, #31245, #25152, #30290, #59909, #26116, #50879, #6503, #20335, #1688, #39937 ),
 .UNSPECIFIED., .F., .F.,
 ( 4, 2, 2, 2, 2, 2, 2, 2, 4 ),
 ( 0.000000000000000000, 0.0008814191908704200945, 0.001762838381740840189, 0.002644257572611260609, 0.003525676763481680378, 0.004407095954352101448, 0.005288515145222522085, 0.006169934336092942721, 0.007051353526963364225 ),
 .UNSPECIFIED. ) ;
#5011=CARTESIAN_POINT ( 'NONE',  ( -59.44456063193725015, -126.5625000013655921, -0.3552334253322034230 ) ) ;
#5013=CARTESIAN_POINT ( 'NONE',  ( -52.80376928212989185, -145.8750000013655779, -4.297418129356378458 ) ) ;
#5024=CARTESIAN_POINT ( 'NONE',  ( -59.29741812935640155, -124.8750000013656205, -2.196230717870135685 ) ) ;
#5046=ORIENTED_EDGE ( 'NONE', *, *, #53080, .F. ) ;
#5047=CARTESIAN_POINT ( 'NONE',  ( -50.70258187064364108, -150.3750000013656063, 2.196230717870141014 ) ) ;
#5057=CARTESIAN_POINT ( 'NONE',  ( -51.75738570946856498, -146.7500000000000284, 3.805975901505576964 ) ) ;
#5064=CARTESIAN_POINT ( 'NONE',  ( -51.60603307380591787, -145.1875000013656063, -2.891590998281053704 ) ) ;
#5065=CARTESIAN_POINT ( 'NONE',  ( -51.19402409849444524, -137.6250000027312410, -3.242614290531456334 ) ) ;
#5078=CARTESIAN_POINT ( 'NONE',  ( -59.44456063193725015, -132.5625000013656063, -0.3552334253322034230 ) ) ;
#5096=CARTESIAN_POINT ( 'NONE',  ( -52.80376928212989185, -139.8750000013655779, -4.297418129356379346 ) ) ;
#5128=CARTESIAN_POINT ( 'NONE',  ( -53.51423613279429503, -152.2500000013656063, 4.591703134518083651 ) ) ;
#5137=CARTESIAN_POINT ( 'NONE',  ( -50.55543936806279248, -128.3125000013656063, 0.3552334253322060320 ) ) ;
#5146=CARTESIAN_POINT ( 'NONE',  ( -59.98410592259440222, -152.2500000027312410, -0.3983568153799752487 ) ) ;
#5167=CARTESIAN_POINT ( 'NONE',  ( -56.48576386720575471, -152.7500000013655779, -4.591703134518078322 ) ) ;
#5172=EDGE_CURVE ( 'NONE', #61334, #29222, #35640, .T. ) ;
#5192=CARTESIAN_POINT ( 'NONE',  ( -59.80389192646541119, -135.0000000000000853, 0.7536779647045089847 ) ) ;
#5213=CARTESIAN_POINT ( 'NONE',  ( -57.89159099828107458, -140.9375000013656063, -3.393966926194107447 ) ) ;
#5221=CARTESIAN_POINT ( 'NONE',  ( -58.24261429053147765, -150.2500000000000284, -3.805975901505573855 ) ) ;
#5224=CARTESIAN_POINT ( 'NONE',  ( -55.00000000000002132, -155.0000000000000284, 1.734723475976807094E-15 ) ) ;
#5234=CARTESIAN_POINT ( 'NONE',  ( -59.29741812935640155, -139.6250000013655779, -2.196230717870135685 ) ) ;
#5260=CARTESIAN_POINT ( 'NONE',  ( -56.48576386720575471, -144.0000000013656063, -4.591703134518078322 ) ) ;
#5285=CARTESIAN_POINT ( 'NONE',  ( -58.80597590150559739, -151.0000000000000284, 3.242614290531460330 ) ) ;
#5288=CARTESIAN_POINT ( 'NONE',  ( -58.24261429053147765, -135.2500000000000284, -3.805975901505573855 ) ) ;
#5301=CARTESIAN_POINT ( 'NONE',  ( -51.75738570946856498, -129.7500000000000284, 3.805975901505576964 ) ) ;
#5310=CARTESIAN_POINT ( 'NONE',  ( -50.40829686548195099, -152.0000000013655779, -1.485763867205728284 ) ) ;
#5316=CARTESIAN_POINT ( 'NONE',  ( -59.81910112700026616, -146.1875000000000000, -2.462841084822510851 ) ) ;
#5336=CARTESIAN_POINT ( 'NONE',  ( -53.51423613279429503, -154.5000000013655779, 4.591703134518082763 ) ) ;
#5337=CARTESIAN_POINT ( 'NONE',  ( -50.70258187064364108, -148.1250000013656063, 2.196230717870141014 ) ) ;
#5346=ORIENTED_EDGE ( 'NONE', *, *, #1728, .T. ) ;
#5367=CARTESIAN_POINT ( 'NONE',  ( -59.44456063193725015, -146.8125000013656063, -0.3552334253322034230 ) ) ;
#5377=CARTESIAN_POINT ( 'NONE',  ( -53.33387254593733928, -143.8125000000000000, 5.149110718188519620 ) ) ;
#5386=CARTESIAN_POINT ( 'NONE',  ( -50.40829686548195099, -146.2500000013656347, -1.485763867205728284 ) ) ;
#5388=CARTESIAN_POINT ( 'NONE',  ( -54.60164318462004474, -136.5000000027312126, -4.984105922594373794 ) ) ;
#5395=ORIENTED_EDGE ( 'NONE', *, *, #23605, .F. ) ;
#5400=CARTESIAN_POINT ( 'NONE',  ( -51.60603307380591787, -133.9375000013656063, -2.891590998281053704 ) ) ;
#5414=CARTESIAN_POINT ( 'NONE',  ( -58.39396692619412477, -138.4375000013656063, 2.891590998281057701 ) ) ;
#5445=CARTESIAN_POINT ( 'NONE',  ( -55.35523342533222291, -151.3125000013656063, 4.444560631937231499 ) ) ;
#5452=CARTESIAN_POINT ( 'NONE',  ( -57.89159099828107458, -126.9375000013656063, -3.393966926194107447 ) ) ;
#5465=CARTESIAN_POINT ( 'NONE',  ( -49.85088928181150436, -151.6875000027311842, -1.666127454062680702 ) ) ;
#5468=ADVANCED_FACE ( 'NONE', ( #33910 ), #9771, .F. ) ;
#5484=CARTESIAN_POINT ( 'NONE',  ( -55.35523342533222291, -151.3125000013656063, 4.444560631937231499 ) ) ;
#5522=ORIENTED_EDGE ( 'NONE', *, *, #1296, .F. ) ;
#5530=CARTESIAN_POINT ( 'NONE',  ( -52.80376928212989185, -140.1250000013655779, -4.297418129356379346 ) ) ;
#5550=CARTESIAN_POINT ( 'NONE',  ( -52.80376928212989185, -142.8750000013656063, -4.297418129356379346 ) ) ;
#5575=CARTESIAN_POINT ( 'NONE',  ( -59.44456063193725015, -145.8125000013656063, -0.3552334253322034230 ) ) ;
#5591=APPLICATION_CONTEXT ( 'automotive_design' ) ;
#5601=CARTESIAN_POINT ( 'NONE',  ( -53.33387254593727533, -150.8125000000000000, 5.149110718188522284 ) ) ;
#5622=CARTESIAN_POINT ( 'NONE',  ( -55.39835681537999790, -130.8750000000000284, 4.984105922594378235 ) ) ;
#5630=CARTESIAN_POINT ( 'NONE',  ( -50.55543936806279248, -154.0625000013656347, 0.3552334253322060320 ) ) ;
#5633=LINE ( 'NONE', #44859, #1457 ) ;
#5635=CARTESIAN_POINT ( 'NONE',  ( -58.80597590150559739, -146.0000000000000284, 3.242614290531460330 ) ) ;
#5654=CARTESIAN_POINT ( 'NONE',  ( -50.40829686548195099, -125.0000000013656205, -1.485763867205728284 ) ) ;
#5655=CARTESIAN_POINT ( 'NONE',  ( -56.48576386720575471, -143.7500000013656063, -4.591703134518078322 ) ) ;
#5696=CARTESIAN_POINT ( 'NONE',  ( -57.46284108482265651, -141.9375000000000000, 4.819101127000239515 ) ) ;
#5698=CARTESIAN_POINT ( 'NONE',  ( -51.75738570946856498, -143.8750000027312126, 3.805975901505576964 ) ) ;
#5705=CARTESIAN_POINT ( 'NONE',  ( -56.48576386720575471, -145.0000000013656063, -4.591703134518078322 ) ) ;
#5707=CARTESIAN_POINT ( 'NONE',  ( -53.33387254593733928, -134.9375000027312126, 5.149110718188519620 ) ) ;
#5719=CARTESIAN_POINT ( 'NONE',  ( -59.59170313451811296, -128.5000000013656063, 1.485763867205729394 ) ) ;
#5725=ORIENTED_EDGE ( 'NONE', *, *, #56583, .F. ) ;
#5734=CARTESIAN_POINT ( 'NONE',  ( -50.40829686548195099, -139.0000000013655779, -1.485763867205728284 ) ) ;
#5741=CARTESIAN_POINT ( 'NONE',  ( -56.48576386720575471, -132.0000000013656063, -4.591703134518078322 ) ) ;
#5746=FACE_OUTER_BOUND ( 'NONE', #38244, .T. ) ;
#5753=CYLINDRICAL_SURFACE ( 'NONE', #656, 5.000000000000000000 ) ;
#5765=CARTESIAN_POINT ( 'NONE',  ( -50.55543936806279248, -150.0625000013656063, 0.3552334253322060320 ) ) ;
#5772=CARTESIAN_POINT ( 'NONE',  ( -54.60164318462004474, -153.3750000000000284, -4.984105922594373794 ) ) ;
#5781=CARTESIAN_POINT ( 'NONE',  ( -53.33387254593733928, -146.9375000027311842, 5.149110718188519620 ) ) ;
#5803=CARTESIAN_POINT ( 'NONE',  ( -52.80376928212989185, -147.8750000013656063, -4.297418129356379346 ) ) ;
#5808=DIRECTION ( 'NONE',  ( 0.8660254037844387076, 0.000000000000000000, 0.4999999999999997780 ) ) ;
#5838=CARTESIAN_POINT ( 'NONE',  ( -56.66612745406280993, -147.4375000027312126, -5.149110718188524061 ) ) ;
#5842=CLOSED_SHELL ( 'NONE', ( #55137, #46871, #24407, #32603, #18518, #104, #37699, #36450, #47631, #44739, #46150, #20564, #58599, #28766, #21225, #20217, #86, #5468, #41517, #20481, #33343, #2789, #18178, #60671, #7509, #8261, #25863, #50241, #15404, #14683, #10685, #11137, #25934, #15056, #3163, #43204, #19589, #4368, #25135, #60551, #32523, #11935, #7795, #60536, #40952, #14676, #101, #27875, #40956, #53092, #30827, #38078, #7160 ) ) ;
#5856=CARTESIAN_POINT ( 'NONE',  ( -50.70258187064364108, -137.3750000013656063, 2.196230717870141014 ) ) ;
#5863=FACE_OUTER_BOUND ( 'NONE', #9027, .T. ) ;
#5866=DIRECTION ( 'NONE',  ( 0.000000000000000000, -1.000000000000000000, 0.000000000000000000 ) ) ;
#5874=CARTESIAN_POINT ( 'NONE',  ( -54.64476657466781973, -140.8125000013656063, -4.444560631937228834 ) ) ;
#5877=VECTOR ( 'NONE', #8745, 1000.000000000000000 ) ;
#5896=( BOUNDED_CURVE ( )  B_SPLINE_CURVE ( 2, ( #54711, #58264, #23852, #24164, #44084, #44722, #14499, #4237, #15145 ),
 .UNSPECIFIED., .F., .F. ) 
 B_SPLINE_CURVE_WITH_KNOTS ( ( 3, 2, 2, 2, 3 ),
 ( 0.4083333333333336590, 0.4125000000000003109, 0.4166666666666670182, 0.4208333333333336701, 0.4250000000000003220 ),
 .UNSPECIFIED. ) 
 CURVE ( )  GEOMETRIC_REPRESENTATION_ITEM ( )  RATIONAL_B_SPLINE_CURVE ( ( 0.9999999999999938938, 0.9238795325112928447, 1.000000000000000000, 0.9238795325112867385, 1.000000000000000000, 0.9238795325112867385, 1.000000000000000000, 0.9238795325112806323, 1.000000000000005995 ) ) 
 REPRESENTATION_ITEM ( '' )  );
#5900=CARTESIAN_POINT ( 'NONE',  ( -54.60164318462004474, -154.3750000000000284, -4.984105922594373794 ) ) ;
#5903=CARTESIAN_POINT ( 'NONE',  ( -58.39396692619412477, -145.6875000013656063, 2.891590998281057701 ) ) ;
#5919=CARTESIAN_POINT ( 'NONE',  ( -50.01589407740564042, -138.7500000027312126, 0.3983568153799778022 ) ) ;
#5945=CARTESIAN_POINT ( 'NONE',  ( -59.81910112700025905, -129.1875000000000284, -2.462841084822630311 ) ) ;
#5948=ORIENTED_EDGE ( 'NONE', *, *, #20136, .T. ) ;
#5952=CARTESIAN_POINT ( 'NONE',  ( -50.40829686548195099, -154.0000000013655779, -1.485763867205728284 ) ) ;
#5961=CARTESIAN_POINT ( 'NONE',  ( -56.66612745406273888, -152.4375000027312126, -5.149110718188518732 ) ) ;
#5985=CARTESIAN_POINT ( 'NONE',  ( -59.59170313451811296, -127.5000000013656347, 1.485763867205729394 ) ) ;
#5986=CARTESIAN_POINT ( 'NONE',  ( -59.59170313451810586, -141.5000000013656063, 1.485763867205729394 ) ) ;
#6005=( BOUNDED_CURVE ( )  B_SPLINE_CURVE ( 2, ( #33676, #23726, #54492, #43629, #43013, #18575, #48468, #38802, #33057 ),
 .UNSPECIFIED., .F., .F. ) 
 B_SPLINE_CURVE_WITH_KNOTS ( ( 3, 2, 2, 2, 3 ),
 ( 0.3083333333333336257, 0.3125000000000002776, 0.3166666666666669294, 0.3208333333333336368, 0.3250000000000002887 ),
 .UNSPECIFIED. ) 
 CURVE ( )  GEOMETRIC_REPRESENTATION_ITEM ( )  RATIONAL_B_SPLINE_CURVE ( ( 0.9999999999999948930, 0.9238795325112918455, 1.000000000000000000, 0.9238795325112867385, 1.000000000000000000, 0.9238795325112867385, 1.000000000000000000, 0.9238795325112816315, 1.000000000000005107 ) ) 
 REPRESENTATION_ITEM ( '' )  );
#6027=CARTESIAN_POINT ( 'NONE',  ( -50.18089887299979068, -142.6875000000000284, 2.462841084822635640 ) ) ;
#6032=PRODUCT_CONTEXT ( 'NONE', #56132, 'mechanical' ) ;
#6036=CARTESIAN_POINT ( 'NONE',  ( -50.70258187064364108, -148.3750000013656063, 2.196230717870141014 ) ) ;
#6038=CARTESIAN_POINT ( 'NONE',  ( -55.39835681537999790, -133.0000000027312126, 4.984105922594378235 ) ) ;
#6050=CARTESIAN_POINT ( 'NONE',  ( -52.10840900171896806, -130.1875000013656063, 3.393966926194110556 ) ) ;
#6052=CARTESIAN_POINT ( 'NONE',  ( -55.39835681537999790, -146.0000000027312126, 4.984105922594378235 ) ) ;
#6063=CARTESIAN_POINT ( 'NONE',  ( -52.10840900171896806, -139.1875000013656347, 3.393966926194110556 ) ) ;
#6073=CARTESIAN_POINT ( 'NONE',  ( -53.51423613279429503, -132.5000000013656063, 4.591703134518082763 ) ) ;
#6079=DIRECTION ( 'NONE',  ( 0.000000000000000000, 1.000000000000000000, 0.000000000000000000 ) ) ;
#6097=CARTESIAN_POINT ( 'NONE',  ( -53.51423613279429503, -149.2500000013656063, 4.591703134518083651 ) ) ;
#6103=DIRECTION ( 'NONE',  ( -0.6485228581062915110, 0.000000000000000000, -0.7611951803011149931 ) ) ;
#6104=CARTESIAN_POINT ( 'NONE',  ( -49.85088928181150436, -152.5625000000000284, -1.666127454062680702 ) ) ;
#6114=CARTESIAN_POINT ( 'NONE',  ( -58.80597590150559739, -148.1250000027312126, 3.242614290531460330 ) ) ;
#6132=CARTESIAN_POINT ( 'NONE',  ( -53.51423613279429503, -149.2500000013655779, 4.591703134518082763 ) ) ;
#6137=DIRECTION ( 'NONE',  ( 0.000000000000000000, 1.000000000000000000, 0.000000000000000000 ) ) ;
#6170=CARTESIAN_POINT ( 'NONE',  ( -60.14911071818854538, -141.1875000027312126, 1.666127454062681146 ) ) ;
#6178=CARTESIAN_POINT ( 'NONE',  ( -54.64476657466781973, -135.0625000013656063, -4.444560631937228834 ) ) ;
#6186=DIRECTION ( 'NONE',  ( 0.000000000000000000, 1.000000000000000000, 0.000000000000000000 ) ) ;
#6189=CARTESIAN_POINT ( 'NONE',  ( -62.00000000000001421, -135.0000000000000284, 4.041451884327384114 ) ) ;
#6195=CARTESIAN_POINT ( 'NONE',  ( -56.48576386720575471, -139.7500000013656347, -4.591703134518078322 ) ) ;
#6221=CARTESIAN_POINT ( 'NONE',  ( -50.55543936806279248, -142.3125000013656063, 0.3552334253322060320 ) ) ;
#6252=VECTOR ( 'NONE', #19345, 1000.000000000000000 ) ;
#6267=CARTESIAN_POINT ( 'NONE',  ( -56.66612745406270335, -128.3125000000000284, -5.149110718188516067 ) ) ;
#6275=CARTESIAN_POINT ( 'NONE',  ( -52.10840900171896806, -151.1875000013656063, 3.393966926194110556 ) ) ;
#6290=DIRECTION ( 'NONE',  ( 0.000000000000000000, 1.000000000000000000, 0.000000000000000000 ) ) ;
#6296=VERTEX_POINT ( 'NONE', #26657 ) ;
#6300=CARTESIAN_POINT ( 'NONE',  ( -59.44456063193725015, -125.5625000013655921, -0.3552334253322034230 ) ) ;
#6301=CARTESIAN_POINT ( 'NONE',  ( -59.29741812935640155, -141.6250000013655495, -2.196230717870135685 ) ) ;
#6323=ORIENTED_EDGE ( 'NONE', *, *, #11677, .T. ) ;
#6341=CARTESIAN_POINT ( 'NONE',  ( -52.53715891517739323, -141.4375000000000284, -4.819101127000233298 ) ) ;
#6351=ORIENTED_EDGE ( 'NONE', *, *, #40525, .F. ) ;
#6353=CARTESIAN_POINT ( 'NONE',  ( -58.39396692619412477, -141.6875000013656063, 2.891590998281057701 ) ) ;
#6355=CARTESIAN_POINT ( 'NONE',  ( -51.75738570946856498, -135.8750000027312410, 3.805975901505576964 ) ) ;
#6368=CARTESIAN_POINT ( 'NONE',  ( -59.29741812935640155, -129.6250000013655779, -2.196230717870135685 ) ) ;
#6382=CARTESIAN_POINT ( 'NONE',  ( -52.10840900171896806, -136.1875000013656063, 3.393966926194110556 ) ) ;
#6393=CARTESIAN_POINT ( 'NONE',  ( -59.59170313451811296, -131.7500000013656063, 1.485763867205729394 ) ) ;
#6405=CARTESIAN_POINT ( 'NONE',  ( -59.81910112700027327, -138.3125000027311842, -2.462841084822392279 ) ) ;
#6423=CARTESIAN_POINT ( 'NONE',  ( -50.01589407740564042, -151.6250000000000284, 0.3983568153799778022 ) ) ;
#6432=CARTESIAN_POINT ( 'NONE',  ( -58.39396692619412477, -154.6875000013656063, 2.891590998281057701 ) ) ;
#6434=CARTESIAN_POINT ( 'NONE',  ( -57.46284108482265651, -146.0625000027312126, 4.819101127000239515 ) ) ;
#6450=CARTESIAN_POINT ( 'NONE',  ( -51.75738570946856498, -144.8750000027312126, 3.805975901505576964 ) ) ;
#6454=CARTESIAN_POINT ( 'NONE',  ( -52.80376928212989185, -149.8750000013655779, -4.297418129356379346 ) ) ;
#6497=CARTESIAN_POINT ( 'NONE',  ( -59.44456063193725015, -135.8125000013656063, -0.3552334253322034230 ) ) ;
#6501=ORIENTED_EDGE ( 'NONE', *, *, #15413, .F. ) ;
#6503=CARTESIAN_POINT ( 'NONE',  ( -51.25142410359330114, -135.0000000000000568, -2.431704782982593294 ) ) ;
#6536=CARTESIAN_POINT ( 'NONE',  ( -52.80376928212989185, -141.1250000013655779, -4.297418129356379346 ) ) ;
#6554=CARTESIAN_POINT ( 'NONE',  ( -50.70258187064364108, -136.3750000013656063, 2.196230717870141014 ) ) ;
#6566=CARTESIAN_POINT ( 'NONE',  ( -56.48576386720575471, -149.0000000013656063, -4.591703134518078322 ) ) ;
#6572=CARTESIAN_POINT ( 'NONE',  ( -55.39835681537999790, -149.0000000027312126, 4.984105922594378235 ) ) ;
#6577=CARTESIAN_POINT ( 'NONE',  ( -60.14911071818854538, -128.0625000000000284, 1.666127454062681368 ) ) ;
#6584=CARTESIAN_POINT ( 'NONE',  ( -57.19623071787017210, -153.3750000013656347, 4.297418129356382899 ) ) ;
#6597=CARTESIAN_POINT ( 'NONE',  ( -51.75738570946856498, -138.7500000000000000, 3.805975901505576964 ) ) ;
#6610=CARTESIAN_POINT ( 'NONE',  ( -59.59170313451811296, -153.7500000013656063, 1.485763867205729394 ) ) ;
#6611=CARTESIAN_POINT ( 'NONE',  ( -54.64476657466781973, -140.8125000013656063, -4.444560631937228834 ) ) ;
#6614=CARTESIAN_POINT ( 'NONE',  ( -58.24261429053147765, -137.2500000000000000, -3.805975901505573855 ) ) ;
#6631=DIRECTION ( 'NONE',  ( 0.000000000000000000, 1.000000000000000000, 0.000000000000000000 ) ) ;
#6652=CARTESIAN_POINT ( 'NONE',  ( -57.46284108482265651, -142.9375000000000000, 4.819101127000239515 ) ) ;
#6662=CARTESIAN_POINT ( 'NONE',  ( -50.40829686548195099, -142.2500000013656063, -1.485763867205728284 ) ) ;
#6664=CARTESIAN_POINT ( 'NONE',  ( -59.98410592259440222, -136.2500000027312126, -0.3983568153799752487 ) ) ;
#6677=CARTESIAN_POINT ( 'NONE',  ( -52.10840900171896806, -127.1875000013656063, 3.393966926194110556 ) ) ;
#6679=CARTESIAN_POINT ( 'NONE',  ( -57.46284108482265651, -142.0625000027312126, 4.819101127000238627 ) ) ;
#6692=CARTESIAN_POINT ( 'NONE',  ( -53.51423613279429503, -137.2500000013656063, 4.591703134518082763 ) ) ;
#6700=DIRECTION ( 'NONE',  ( -0.6485228581062915110, 0.000000000000000000, -0.7611951803011149931 ) ) ;
#6701=EDGE_LOOP ( 'NONE', ( #51330, #53753, #24980, #13443 ) ) ;
#6703=CARTESIAN_POINT ( 'NONE',  ( -57.89159099828107458, -130.9375000013656063, -3.393966926194107447 ) ) ;
#6735=CARTESIAN_POINT ( 'NONE',  ( -60.14911071818854538, -154.0625000000000000, 1.666127454062681368 ) ) ;
#6746=CARTESIAN_POINT ( 'NONE',  ( -59.98410592259440222, -147.2500000027312126, -0.3983568153799752487 ) ) ;
#6762=CARTESIAN_POINT ( 'NONE',  ( -62.00000000000001421, -135.0000000000000284, 4.041451884327384114 ) ) ;
#6765=CARTESIAN_POINT ( 'NONE',  ( -50.55543936806279248, -150.0625000013656063, 0.3552334253322060320 ) ) ;
#6800=DIRECTION ( 'NONE',  ( 0.000000000000000000, 1.000000000000000000, 0.000000000000000000 ) ) ;
#6816=CARTESIAN_POINT ( 'NONE',  ( -56.48576386720575471, -136.0000000013656063, -4.591703134518078322 ) ) ;
#6857=CARTESIAN_POINT ( 'NONE',  ( -54.64476657466781973, -138.0625000013656063, -4.444560631937228834 ) ) ;
#6871=CARTESIAN_POINT ( 'NONE',  ( -51.19402409849444524, -138.6250000027312410, -3.242614290531456334 ) ) ;
#6877=CARTESIAN_POINT ( 'NONE',  ( -59.59170313451810586, -135.7500000013656063, 1.485763867205729394 ) ) ;
#6883=CARTESIAN_POINT ( 'NONE',  ( -60.14911071818854538, -139.0625000000000284, 1.666127454062681146 ) ) ;
#6889=CARTESIAN_POINT ( 'NONE',  ( -59.44456063193725015, -148.8125000013656063, -0.3552334253322034230 ) ) ;
#6901=CARTESIAN_POINT ( 'NONE',  ( -59.81910112700025905, -126.1875000000000426, -2.462841084822630311 ) ) ;
#6910=CARTESIAN_POINT ( 'NONE',  ( -54.64476657466781973, -147.8125000013656063, -4.444560631937228834 ) ) ;
#6919=CARTESIAN_POINT ( 'NONE',  ( -58.24261429053147765, -152.3750000027312126, -3.805975901505573855 ) ) ;
#6930=ORIENTED_EDGE ( 'NONE', *, *, #14786, .F. ) ;
#6934=CARTESIAN_POINT ( 'NONE',  ( -57.89159099828107458, -150.9375000013656063, -3.393966926194107447 ) ) ;
#6936=CARTESIAN_POINT ( 'NONE',  ( -57.19623071787016499, -143.3750000013656063, 4.297418129356382899 ) ) ;
#6939=CARTESIAN_POINT ( 'NONE',  ( -57.46284108482265651, -136.9375000000000000, 4.819101127000238627 ) ) ;
#6975=CARTESIAN_POINT ( 'NONE',  ( -59.98410592259440222, -141.1250000000000284, -0.3983568153799752487 ) ) ;
#6982=CARTESIAN_POINT ( 'NONE',  ( -60.14911071818854538, -137.1875000027312126, 1.666127454062681146 ) ) ;
#6985=CARTESIAN_POINT ( 'NONE',  ( -56.48576386720575471, -144.0000000013656063, -4.591703134518078322 ) ) ;
#6987=CARTESIAN_POINT ( 'NONE',  ( -50.01589407740564042, -130.7500000027312126, 0.3983568153799778022 ) ) ;
#7001=CARTESIAN_POINT ( 'NONE',  ( -52.80376928212989185, -129.8750000013656063, -4.297418129356379346 ) ) ;
#7006=ORIENTED_EDGE ( 'NONE', *, *, #38613, .F. ) ;
#7007=CARTESIAN_POINT ( 'NONE',  ( -54.60164318462004474, -146.3750000000000284, -4.984105922594373794 ) ) ;
#7014=CARTESIAN_POINT ( 'NONE',  ( -50.55543936806279248, -133.0625000013656063, 0.3552334253322060320 ) ) ;
#7024=CARTESIAN_POINT ( 'NONE',  ( -59.29741812935640155, -129.8750000013656063, -2.196230717870135685 ) ) ;
#7034=ORIENTED_EDGE ( 'NONE', *, *, #40264, .T. ) ;
#7049=CARTESIAN_POINT ( 'NONE',  ( -51.60603307380591787, -136.9375000013655779, -2.891590998281053704 ) ) ;
#7054=CARTESIAN_POINT ( 'NONE',  ( -57.46284108482265651, -152.9375000000000000, 4.819101127000239515 ) ) ;
#7064=CARTESIAN_POINT ( 'NONE',  ( -50.40829686548195099, -154.2500000013656063, -1.485763867205728284 ) ) ;
#7066=CARTESIAN_POINT ( 'NONE',  ( -54.60164318462004474, -145.5000000027312126, -4.984105922594373794 ) ) ;
#7087=CARTESIAN_POINT ( 'NONE',  ( -57.89159099828107458, -144.6875000013656063, -3.393966926194107447 ) ) ;
#7131=CARTESIAN_POINT ( 'NONE',  ( -57.19623071787017210, -136.6250000013655779, 4.297418129356382899 ) ) ;
#7147=VECTOR ( 'NONE', #44056, 1000.000000000000114 ) ;
#7160=ADVANCED_FACE ( 'NONE', ( #3523 ), #23133, .T. ) ;
#7180=CARTESIAN_POINT ( 'NONE',  ( -52.80376928212989185, -138.1250000013656063, -4.297418129356379346 ) ) ;
#7210=CARTESIAN_POINT ( 'NONE',  ( -52.10840900171896806, -145.4375000013656063, 3.393966926194110556 ) ) ;
#7218=CARTESIAN_POINT ( 'NONE',  ( -62.00000000000001421, -135.0000000000000284, 4.041451884327384114 ) ) ;
#7221=VERTEX_POINT ( 'NONE', #58491 ) ;
#7224=CARTESIAN_POINT ( 'NONE',  ( -50.18089887299979068, -126.6875000000000426, 2.462841084822635640 ) ) ;
#7228=ORIENTED_EDGE ( 'NONE', *, *, #10330, .F. ) ;
#7233=CARTESIAN_POINT ( 'NONE',  ( -50.40829686548195099, -149.0000000013656063, -1.485763867205728284 ) ) ;
#7235=ORIENTED_EDGE ( 'NONE', *, *, #10335, .T. ) ;
#7240=VECTOR ( 'NONE', #14790, 1000.000000000000000 ) ;
#7258=CARTESIAN_POINT ( 'NONE',  ( -50.55543936806279248, -153.3125000013656063, 0.3552334253322060320 ) ) ;
#7269=CARTESIAN_POINT ( 'NONE',  ( -59.81910112700025905, -153.1875000000000000, -2.462841084822604110 ) ) ;
#7297=CARTESIAN_POINT ( 'NONE',  ( -58.80597590150559739, -136.0000000000000284, 3.242614290531460330 ) ) ;
#7301=( BOUNDED_CURVE ( )  B_SPLINE_CURVE ( 2, ( #20279, #54695, #10935, #39881, #40524, #25418, #16089, #1004, #45036 ),
 .UNSPECIFIED., .F., .F. ) 
 B_SPLINE_CURVE_WITH_KNOTS ( ( 3, 2, 2, 2, 3 ),
 ( 0.3750000000000002776, 0.3791666666666669294, 0.3833333333333336368, 0.3875000000000003442, 0.3916666666666669960 ),
 .UNSPECIFIED. ) 
 CURVE ( )  GEOMETRIC_REPRESENTATION_ITEM ( )  RATIONAL_B_SPLINE_CURVE ( ( 0.9999999999999948930, 0.9238795325112918455, 1.000000000000000000, 0.9238795325112867385, 1.000000000000000000, 0.9238795325112867385, 1.000000000000000000, 0.9238795325112806323, 1.000000000000005995 ) ) 
 REPRESENTATION_ITEM ( '' )  );
#7307=CARTESIAN_POINT ( 'NONE',  ( -53.51423613279429503, -141.5000000013656063, 4.591703134518083651 ) ) ;
#7309=CARTESIAN_POINT ( 'NONE',  ( -59.98410592259440222, -132.2500000027312126, -0.3983568153799752487 ) ) ;
#7322=CARTESIAN_POINT ( 'NONE',  ( -59.98410592259440222, -154.1250000000000284, -0.3983568153799752487 ) ) ;
#7323=CARTESIAN_POINT ( 'NONE',  ( -52.80376928212989185, -124.8750000013656205, -4.297418129356379346 ) ) ;
#7336=CARTESIAN_POINT ( 'NONE',  ( -57.19623071787017210, -133.3750000013656063, 4.297418129356382899 ) ) ;
#7345=CARTESIAN_POINT ( 'NONE',  ( -56.48576386720575471, -130.0000000013656063, -4.591703134518078322 ) ) ;
#7348=EDGE_CURVE ( 'NONE', #32996, #25453, #13921, .T. ) ;
#7368=CARTESIAN_POINT ( 'NONE',  ( -50.55543936806279248, -153.3125000013656063, 0.3552334253322060320 ) ) ;
#7372=CARTESIAN_POINT ( 'NONE',  ( -59.29741812935640155, -137.6250000013655779, -2.196230717870135685 ) ) ;
#7377=CARTESIAN_POINT ( 'NONE',  ( -55.39835681537999790, -150.8750000000000284, 4.984105922594378235 ) ) ;
#7381=FILL_AREA_STYLE ('',( #46291 ) ) ;
#7387=CARTESIAN_POINT ( 'NONE',  ( -50.01589407740564042, -142.7500000027312126, 0.3983568153799778022 ) ) ;
#7394=CARTESIAN_POINT ( 'NONE',  ( -59.59170313451811296, -136.5000000013656347, 1.485763867205729394 ) ) ;
#7408=CARTESIAN_POINT ( 'NONE',  ( -56.48576386720575471, -143.7500000013656063, -4.591703134518078322 ) ) ;
#7412=DIRECTION ( 'NONE',  ( -0.6485228581062915110, 0.000000000000000000, -0.7611951803011149931 ) ) ;
#7425=CARTESIAN_POINT ( 'NONE',  ( -55.00000000000002132, -155.0000000000000284, 1.734723475976807094E-15 ) ) ;
#7452=CARTESIAN_POINT ( 'NONE',  ( -53.51423613279429503, -133.5000000013656347, 4.591703134518082763 ) ) ;
#7460=CARTESIAN_POINT ( 'NONE',  ( -58.24261429053147765, -153.3750000027312126, -3.805975901505573855 ) ) ;
#7491=CARTESIAN_POINT ( 'NONE',  ( -57.19623071787017210, -138.6250000013655779, 4.297418129356382899 ) ) ;
#7492=( BOUNDED_CURVE ( )  B_SPLINE_CURVE ( 2, ( #22897, #56039, #38305, #23828, #23195, #28951, #9337, #8414, #3899 ),
 .UNSPECIFIED., .F., .F. ) 
 B_SPLINE_CURVE_WITH_KNOTS ( ( 3, 2, 2, 2, 3 ),
 ( 0.1083333333333334203, 0.1125000000000000999, 0.1166666666666667657, 0.1208333333333334314, 0.1250000000000001110 ),
 .UNSPECIFIED. ) 
 CURVE ( )  GEOMETRIC_REPRESENTATION_ITEM ( )  RATIONAL_B_SPLINE_CURVE ( ( 0.9999999999999984457, 0.9238795325112882928, 1.000000000000000000, 0.9238795325112867385, 1.000000000000000000, 0.9238795325112867385, 1.000000000000000000, 0.9238795325112847401, 1.000000000000001998 ) ) 
 REPRESENTATION_ITEM ( '' )  );
#7501=ORIENTED_EDGE ( 'NONE', *, *, #29899, .F. ) ;
#7509=ADVANCED_FACE ( 'NONE', ( #55751 ), #49960, .F. ) ;
#7525=CARTESIAN_POINT ( 'NONE',  ( -52.10840900171896806, -148.4375000013656063, 3.393966926194110556 ) ) ;
#7528=VERTEX_POINT ( 'NONE', #21973 ) ;
#7535=LINE ( 'NONE', #43736, #59097 ) ;
#7536=CARTESIAN_POINT ( 'NONE',  ( -59.81910112700025905, -125.1875000000000284, -2.462841084822630311 ) ) ;
#7544=CARTESIAN_POINT ( 'NONE',  ( -58.39396692619412477, -147.4375000013656063, 2.891590998281057701 ) ) ;
#7568=CARTESIAN_POINT ( 'NONE',  ( -51.60603307380591787, -153.1875000013656063, -2.891590998281053704 ) ) ;
#7576=CARTESIAN_POINT ( 'NONE',  ( -58.80597590150559739, -138.1250000027312410, 3.242614290531460330 ) ) ;
#7593=DIRECTION ( 'NONE',  ( -0.6485228581062915110, 0.000000000000000000, -0.7611951803011149931 ) ) ;
#7613=CARTESIAN_POINT ( 'NONE',  ( -59.81910112700025905, -139.1874999999999716, -2.462841084822630311 ) ) ;
#7622=CARTESIAN_POINT ( 'NONE',  ( -50.55543936806279248, -141.3125000013656063, 0.3552334253322060320 ) ) ;
#7624=CARTESIAN_POINT ( 'NONE',  ( -49.85088928181150436, -130.6875000027312410, -1.666127454062680702 ) ) ;
#7636=CARTESIAN_POINT ( 'NONE',  ( -52.80376928212989185, -125.8750000013656063, -4.297418129356379346 ) ) ;
#7642=CARTESIAN_POINT ( 'NONE',  ( -51.75738570946856498, -139.8750000027312126, 3.805975901505576964 ) ) ;
#7647=DIRECTION ( 'NONE',  ( 0.000000000000000000, 1.000000000000000000, 0.000000000000000000 ) ) ;
#7649=CARTESIAN_POINT ( 'NONE',  ( -57.89159099828107458, -134.6875000013656063, -3.393966926194107447 ) ) ;
#7659=CARTESIAN_POINT ( 'NONE',  ( -59.44456063193725015, -126.8125000013655921, -0.3552334253322034230 ) ) ;
#7683=DIRECTION ( 'NONE',  ( -0.4999999999999998890, 0.000000000000000000, -0.8660254037844387076 ) ) ;
#7687=CARTESIAN_POINT ( 'NONE',  ( -57.89159099828107458, -137.6875000013656063, -3.393966926194107447 ) ) ;
#7692=CARTESIAN_POINT ( 'NONE',  ( -60.14911071818854538, -150.0625000000000000, 1.666127454062681368 ) ) ;
#7698=( LENGTH_UNIT ( ) NAMED_UNIT ( * ) SI_UNIT ( .MILLI., .METRE. ) );
#7703=CARTESIAN_POINT ( 'NONE',  ( -59.59170313451810586, -153.7500000013656063, 1.485763867205729394 ) ) ;
#7704=CARTESIAN_POINT ( 'NONE',  ( -51.19402409849444524, -142.6250000027312126, -3.242614290531456334 ) ) ;
#7711=CARTESIAN_POINT ( 'NONE',  ( -57.19623071787017210, -136.3750000013656063, 4.297418129356382899 ) ) ;
#7724=CARTESIAN_POINT ( 'NONE',  ( -53.51423613279429503, -147.2500000013656063, 4.591703134518082763 ) ) ;
#7763=CARTESIAN_POINT ( 'NONE',  ( -55.35523342533222291, -129.5625000013656063, 4.444560631937231499 ) ) ;
#7769=CARTESIAN_POINT ( 'NONE',  ( -50.01589407740564042, -153.7500000027312410, 0.3983568153799778022 ) ) ;
#7793=CARTESIAN_POINT ( 'NONE',  ( -52.53715891517739323, -138.4375000000000000, -4.819101127000233298 ) ) ;
#7795=ADVANCED_FACE ( 'NONE', ( #44732 ), #63422, .T. ) ;
#7798=DIRECTION ( 'NONE',  ( 0.000000000000000000, 1.000000000000000000, 0.000000000000000000 ) ) ;
#7809=CARTESIAN_POINT ( 'NONE',  ( -54.64476657466781973, -139.0625000013656063, -4.444560631937228834 ) ) ;
#7827=CARTESIAN_POINT ( 'NONE',  ( -50.70258187064364108, -135.3750000013656063, 2.196230717870141014 ) ) ;
#7839=CARTESIAN_POINT ( 'NONE',  ( -52.10840900171896806, -143.4375000013656063, 3.393966926194110556 ) ) ;
#7849=CARTESIAN_POINT ( 'NONE',  ( -58.80597590150559739, -152.0000000000000284, 3.242614290531460330 ) ) ;
#7850=CARTESIAN_POINT ( 'NONE',  ( -55.39835681537999790, -126.8750000000000142, 4.984105922594378235 ) ) ;
#7858=CARTESIAN_POINT ( 'NONE',  ( -57.89159099828107458, -149.6875000013656063, -3.393966926194107447 ) ) ;
#7870=EDGE_CURVE ( 'NONE', #10962, #58935, #40226, .T. ) ;
#7872=CARTESIAN_POINT ( 'NONE',  ( -56.66612745406293783, -140.4375000027311842, -5.149110718188535607 ) ) ;
#7885=CARTESIAN_POINT ( 'NONE',  ( -53.51423613279429503, -150.5000000013655779, 4.591703134518082763 ) ) ;
#7895=CARTESIAN_POINT ( 'NONE',  ( -59.98410592259440222, -153.1250000000000284, -0.3983568153799752487 ) ) ;
#7923=CARTESIAN_POINT ( 'NONE',  ( -53.33387254593733928, -138.8125000000000284, 5.149110718188519620 ) ) ;
#7934=DIRECTION ( 'NONE',  ( 0.000000000000000000, 1.000000000000000000, 0.000000000000000000 ) ) ;
#7935=CARTESIAN_POINT ( 'NONE',  ( -52.80376928212989185, -137.1250000013656063, -4.297418129356378458 ) ) ;
#7937=CARTESIAN_POINT ( 'NONE',  ( -56.66612745406270335, -129.4375000027312126, -5.149110718188516067 ) ) ;
#7963=CARTESIAN_POINT ( 'NONE',  ( -59.29741812935640155, -133.6250000013655779, -2.196230717870135685 ) ) ;
#7974=CARTESIAN_POINT ( 'NONE',  ( -59.44456063193725015, -128.8125000013656063, -0.3552334253322034230 ) ) ;
#7987=CARTESIAN_POINT ( 'NONE',  ( -55.39835681537999790, -139.0000000027312126, 4.984105922594378235 ) ) ;
#7999=CARTESIAN_POINT ( 'NONE',  ( -57.89159099828107458, -138.6875000013656347, -3.393966926194107447 ) ) ;
#8005=CARTESIAN_POINT ( 'NONE',  ( -51.75738570946856498, -148.7500000000000284, 3.805975901505576964 ) ) ;
#8015=CARTESIAN_POINT ( 'NONE',  ( -53.51423613279429503, -151.5000000013655779, 4.591703134518083651 ) ) ;
#8016=CARTESIAN_POINT ( 'NONE',  ( -60.14911071818854538, -142.1875000027312410, 1.666127454062681368 ) ) ;
#8018=VECTOR ( 'NONE', #40272, 1000.000000000000000 ) ;
#8023=CARTESIAN_POINT ( 'NONE',  ( -59.44456063193725015, -135.5625000013656063, -0.3552334253322034230 ) ) ;
#8039=CARTESIAN_POINT ( 'NONE',  ( -59.29741812935640155, -145.6250000013655779, -2.196230717870135685 ) ) ;
#8055=CARTESIAN_POINT ( 'NONE',  ( -59.81910112700027327, -149.1875000000000284, -2.462841084822540605 ) ) ;
#8084=CARTESIAN_POINT ( 'NONE',  ( -50.55543936806279248, -132.3125000013656063, 0.3552334253322060320 ) ) ;
#8091=CARTESIAN_POINT ( 'NONE',  ( -50.18089887299979068, -153.8125000027312126, 2.462841084822635640 ) ) ;
#8126=CARTESIAN_POINT ( 'NONE',  ( -59.29741812935640155, -134.8750000013656063, -2.196230717870135685 ) ) ;
#8150=CARTESIAN_POINT ( 'NONE',  ( -55.00000000000002132, -155.0000000000000284, 1.734723475976807094E-15 ) ) ;
#8160=CARTESIAN_POINT ( 'NONE',  ( -59.44456063193725015, -142.8125000013656063, -0.3552334253322034230 ) ) ;
#8164=CARTESIAN_POINT ( 'NONE',  ( -55.39835681537999790, -148.0000000027312126, 4.984105922594378235 ) ) ;
#8170=CARTESIAN_POINT ( 'NONE',  ( -60.14911071818854538, -125.0625000000000142, 1.666127454062681368 ) ) ;
#8177=CARTESIAN_POINT ( 'NONE',  ( -55.35523342533222291, -148.3125000013656063, 4.444560631937231499 ) ) ;
#8194=DIRECTION ( 'NONE',  ( 0.000000000000000000, 1.000000000000000000, 0.000000000000000000 ) ) ;
#8201=CARTESIAN_POINT ( 'NONE',  ( -57.89159099828107458, -148.9375000013656063, -3.393966926194107447 ) ) ;
#8238=CARTESIAN_POINT ( 'NONE',  ( -58.24261429053147765, -155.0000000000000284, -3.805975901505573411 ) ) ;
#8239=CARTESIAN_POINT ( 'NONE',  ( -54.60164318462004474, -139.3750000000000284, -4.984105922594373794 ) ) ;
#8250=CARTESIAN_POINT ( 'NONE',  ( -50.55543936806279248, -140.3125000013656063, 0.3552334253322060320 ) ) ;
#8252=CARTESIAN_POINT ( 'NONE',  ( -50.18089887299979068, -129.8125000027312126, 2.462841084822635640 ) ) ;
#8261=ADVANCED_FACE ( 'NONE', ( #61147 ), #52440, .F. ) ;
#8274=CARTESIAN_POINT ( 'NONE',  ( -57.89159099828107458, -131.6875000013656063, -3.393966926194107447 ) ) ;
#8284=CARTESIAN_POINT ( 'NONE',  ( -57.19623071787017210, -127.6250000013656205, 4.297418129356382899 ) ) ;
#8315=CARTESIAN_POINT ( 'NONE',  ( -56.48576386720575471, -139.7500000013656347, -4.591703134518078322 ) ) ;
#8321=CARTESIAN_POINT ( 'NONE',  ( -54.60164318462004474, -150.3750000000000284, -4.984105922594373794 ) ) ;
#8331=CARTESIAN_POINT ( 'NONE',  ( -59.29741812935640155, -149.8750000013655779, -2.196230717870135685 ) ) ;
#8332=CARTESIAN_POINT ( 'NONE',  ( -50.01589407740564042, -140.7500000027312126, 0.3983568153799778022 ) ) ;
#8339=CARTESIAN_POINT ( 'NONE',  ( -52.80376928212989185, -138.8750000013655779, -4.297418129356379346 ) ) ;
#8354=CARTESIAN_POINT ( 'NONE',  ( -55.35523342533222291, -144.3125000013656063, 4.444560631937231499 ) ) ;
#8356=CARTESIAN_POINT ( 'NONE',  ( -51.75738570946856498, -135.8750000027312410, 3.805975901505576964 ) ) ;
#8389=CARTESIAN_POINT ( 'NONE',  ( -51.75738570946856498, -140.8750000027312126, 3.805975901505576964 ) ) ;
#8399=CARTESIAN_POINT ( 'NONE',  ( -52.80376928212989185, -130.1250000013656347, -4.297418129356379346 ) ) ;
#8406=CARTESIAN_POINT ( 'NONE',  ( -57.46284108482265651, -153.0625000027312126, 4.819101127000239515 ) ) ;
#8414=CARTESIAN_POINT ( 'NONE',  ( -56.66612745406273888, -150.4375000027311842, -5.149110718188520508 ) ) ;
#8437=CARTESIAN_POINT ( 'NONE',  ( -58.80597590150559739, -145.1250000027312126, 3.242614290531460330 ) ) ;
#8440=CARTESIAN_POINT ( 'NONE',  ( -55.35523342533222291, -134.5625000013656063, 4.444560631937231499 ) ) ;
#8469=CARTESIAN_POINT ( 'NONE',  ( -58.39396692619412477, -141.6875000013656063, 2.891590998281057701 ) ) ;
#8473=CARTESIAN_POINT ( 'NONE',  ( -51.75738570946856498, -147.8750000027312126, 3.805975901505576964 ) ) ;
#8485=CARTESIAN_POINT ( 'NONE',  ( -51.60603307380591787, -143.9375000013656063, -2.891590998281053704 ) ) ;
#8510=CARTESIAN_POINT ( 'NONE',  ( -57.19623071787017210, -148.6250000013656063, 4.297418129356382899 ) ) ;
#8516=CARTESIAN_POINT ( 'NONE',  ( -58.80597590150559739, -136.1250000027312410, 3.242614290531460330 ) ) ;
#8546=CARTESIAN_POINT ( 'NONE',  ( -59.98410592259440222, -136.1250000000000284, -0.3983568153799752487 ) ) ;
#8553=CARTESIAN_POINT ( 'NONE',  ( -57.19623071787016499, -139.6250000013655779, 4.297418129356382899 ) ) ;
#8555=CARTESIAN_POINT ( 'NONE',  ( -59.98410592259440222, -128.2500000027312126, -0.3983568153799752487 ) ) ;
#8560=CARTESIAN_POINT ( 'NONE',  ( -51.75738570946856498, -150.8750000027312126, 3.805975901505576964 ) ) ;
#8564=DIRECTION ( 'NONE',  ( 0.000000000000000000, 1.000000000000000000, 0.000000000000000000 ) ) ;
#8568=CARTESIAN_POINT ( 'NONE',  ( -57.19623071787017210, -125.3750000013656205, 4.297418129356382899 ) ) ;
#8579=CARTESIAN_POINT ( 'NONE',  ( -59.29741812935640155, -130.6250000013656347, -2.196230717870135685 ) ) ;
#8580=EDGE_CURVE ( 'NONE', #46979, #24361, #55833, .T. ) ;
#8610=( BOUNDED_CURVE ( )  B_SPLINE_CURVE ( 2, ( #32960, #53826, #9445, #38406, #8516, #38708, #28126, #13654, #14275 ),
 .UNSPECIFIED., .F., .F. ) 
 B_SPLINE_CURVE_WITH_KNOTS ( ( 3, 2, 2, 2, 3 ),
 ( 0.5916666666666671182, 0.5958333333333335480, 0.6000000000000000888, 0.6041666666666665186, 0.6083333333333329485 ),
 .UNSPECIFIED. ) 
 CURVE ( )  GEOMETRIC_REPRESENTATION_ITEM ( )  RATIONAL_B_SPLINE_CURVE ( ( 0.9999999999999918954, 0.9238795325112948431, 1.000000000000000000, 0.9238795325112867385, 1.000000000000000000, 0.9238795325112867385, 1.000000000000000000, 0.9238795325112928447, 0.9999999999999938938 ) ) 
 REPRESENTATION_ITEM ( '' )  );
#8615=CARTESIAN_POINT ( 'NONE',  ( -58.39396692619412477, -151.6875000013656063, 2.891590998281057701 ) ) ;
#8619=CARTESIAN_POINT ( 'NONE',  ( -59.44456063193725015, -135.5625000013656063, -0.3552334253322034230 ) ) ;
#8623=ORIENTED_EDGE ( 'NONE', *, *, #7348, .T. ) ;
#8624=CARTESIAN_POINT ( 'NONE',  ( -50.18089887299979068, -147.6875000000000284, 2.462841084822635640 ) ) ;
#8632=CARTESIAN_POINT ( 'NONE',  ( -52.10840900171896806, -151.4375000013656063, 3.393966926194110556 ) ) ;
#8633=CARTESIAN_POINT ( 'NONE',  ( -57.46284108482265651, -142.0625000027311842, 4.819101127000239515 ) ) ;
#8641=CARTESIAN_POINT ( 'NONE',  ( -50.55543936806279248, -137.0625000013656063, 0.3552334253322060320 ) ) ;
#8647=ORIENTED_EDGE ( 'NONE', *, *, #35025, .T. ) ;
#8656=CARTESIAN_POINT ( 'NONE',  ( -52.80376928212989185, -141.8750000013655779, -4.297418129356379346 ) ) ;
#8660=( BOUNDED_CURVE ( )  B_SPLINE_CURVE ( 2, ( #48800, #53322, #28870, #33702, #4740, #18283, #58144 ),
 .UNSPECIFIED., .F., .F. ) 
 B_SPLINE_CURVE_WITH_KNOTS ( ( 3, 2, 2, 3 ),
 ( 0.6249999999999996669, 0.6291666666666664298, 0.6333333333333331927, 0.6375000000985409088 ),
 .UNSPECIFIED. ) 
 CURVE ( )  GEOMETRIC_REPRESENTATION_ITEM ( )  RATIONAL_B_SPLINE_CURVE ( ( 1.000000000000005995, 0.9238795325112806323, 1.000000000000000000, 0.9238795325112867385, 1.000000000000000000, 0.9238795325112867385, 1.000000000000000000 ) ) 
 REPRESENTATION_ITEM ( '' )  );
#8691=CARTESIAN_POINT ( 'NONE',  ( -59.44456063193725015, -153.5625000013656063, -0.3552334253322034230 ) ) ;
#8695=CARTESIAN_POINT ( 'NONE',  ( -51.75738570946856498, -149.8750000027312126, 3.805975901505576964 ) ) ;
#8698=CARTESIAN_POINT ( 'NONE',  ( -52.80376928212989185, -131.1250000013655779, -4.297418129356379346 ) ) ;
#8704=CARTESIAN_POINT ( 'NONE',  ( -53.33387254593716875, -142.8125000000000284, 5.149110718188532942 ) ) ;
#8706=CARTESIAN_POINT ( 'NONE',  ( -49.85088928181150436, -153.6875000027311842, -1.666127454062680702 ) ) ;
#8713=EDGE_CURVE ( 'NONE', #58923, #37814, #47217, .T. ) ;
#8731=CARTESIAN_POINT ( 'NONE',  ( -51.75738570946856498, -144.7500000000000284, 3.805975901505576964 ) ) ;
#8733=CARTESIAN_POINT ( 'NONE',  ( -57.89159099828107458, -153.6875000013656063, -3.393966926194107447 ) ) ;
#8745=DIRECTION ( 'NONE',  ( 0.000000000000000000, 1.000000000000000000, 0.000000000000000000 ) ) ;
#8749=CARTESIAN_POINT ( 'NONE',  ( -51.60603307380591787, -135.1875000013656063, -2.891590998281053704 ) ) ;
#8767=CARTESIAN_POINT ( 'NONE',  ( -58.24261429053147765, -144.3750000027312126, -3.805975901505573855 ) ) ;
#8777=CARTESIAN_POINT ( 'NONE',  ( -50.40829686548195099, -143.2500000013656063, -1.485763867205728284 ) ) ;
#8795=CARTESIAN_POINT ( 'NONE',  ( -51.60603307380591787, -145.9375000013656063, -2.891590998281053704 ) ) ;
#8814=CARTESIAN_POINT ( 'NONE',  ( -58.24261429053147765, -152.2500000000000284, -3.805975901505573855 ) ) ;
#8821=AXIS2_PLACEMENT_3D ( 'NONE', #32656, #12407, #7593 ) ;
#8822=CARTESIAN_POINT ( 'NONE',  ( -56.48576386720575471, -150.0000000013655779, -4.591703134518078322 ) ) ;
#8829=CARTESIAN_POINT ( 'NONE',  ( -51.75738570946856498, -147.7500000000000284, 3.805975901505576964 ) ) ;
#8844=CARTESIAN_POINT ( 'NONE',  ( -55.00000000000002132, -155.0000000000000284, 1.734723475976807094E-15 ) ) ;
#8846=CARTESIAN_POINT ( 'NONE',  ( -51.19402409849444524, -135.5000000000000284, -3.242614290531456334 ) ) ;
#8859=CARTESIAN_POINT ( 'NONE',  ( -58.24261429053147765, -135.2500000000000284, -3.805975901505573855 ) ) ;
#8865=LINE ( 'NONE', #4660, #61546 ) ;
#8867=CARTESIAN_POINT ( 'NONE',  ( -59.59170313451810586, -137.7500000013656063, 1.485763867205729394 ) ) ;
#8869=CARTESIAN_POINT ( 'NONE',  ( -52.53715891517739323, -128.5625000027311842, -4.819101127000233298 ) ) ;
#8877=CARTESIAN_POINT ( 'NONE',  ( -58.24261429053147765, -155.0000000000000284, -3.805975901505573411 ) ) ;
#8893=CARTESIAN_POINT ( 'NONE',  ( -55.35523342533222291, -130.3125000013656063, 4.444560631937231499 ) ) ;
#8894=CARTESIAN_POINT ( 'NONE',  ( -59.44456063193725015, -148.5625000013656063, -0.3552334253322034230 ) ) ;
#8923=EDGE_CURVE ( 'NONE', #9785, #55783, #9034, .T. ) ;
#8927=CARTESIAN_POINT ( 'NONE',  ( -50.40829686548195099, -152.2500000013656347, -1.485763867205728284 ) ) ;
#8931=CARTESIAN_POINT ( 'NONE',  ( -57.89159099828107458, -135.6875000013656063, -3.393966926194107447 ) ) ;
#8936=CARTESIAN_POINT ( 'NONE',  ( -56.66612745406270335, -145.3125000000000284, -5.149110718188516067 ) ) ;
#8944=CARTESIAN_POINT ( 'NONE',  ( -52.80376928212989185, -151.1250000013656347, -4.297418129356378458 ) ) ;
#8945=CARTESIAN_POINT ( 'NONE',  ( -53.33387254593733928, -138.9375000027312126, 5.149110718188519620 ) ) ;
#8948=CARTESIAN_POINT ( 'NONE',  ( -62.00000000000001421, -155.0000000000000284, 4.041451884327384114 ) ) ;
#8957=CARTESIAN_POINT ( 'NONE',  ( -59.29741812935640155, -131.6250000013655779, -2.196230717870135685 ) ) ;
#8973=CARTESIAN_POINT ( 'NONE',  ( -51.60603307380591787, -142.9375000013656063, -2.891590998281053704 ) ) ;
#9003=CARTESIAN_POINT ( 'NONE',  ( -51.75738570946856498, -155.0000000000000284, 3.805975901505577408 ) ) ;
#9006=CARTESIAN_POINT ( 'NONE',  ( -57.89159099828107458, -153.6875000013656063, -3.393966926194107447 ) ) ;
#9014=CARTESIAN_POINT ( 'NONE',  ( -55.35523342533222291, -131.5625000013656063, 4.444560631937231499 ) ) ;
#9024=CARTESIAN_POINT ( 'NONE',  ( -55.39835681537999790, -151.0000000027312410, 4.984105922594378235 ) ) ;
#9027=EDGE_LOOP ( 'NONE', ( #40370, #50237, #29498, #4465 ) ) ;
#9034=( BOUNDED_CURVE ( )  B_SPLINE_CURVE ( 2, ( #11722, #16246, #45828, #40996, #60640, #2112, #31339, #5961, #6919 ),
 .UNSPECIFIED., .F., .F. ) 
 B_SPLINE_CURVE_WITH_KNOTS ( ( 3, 2, 2, 2, 3 ),
 ( 0.04166666666666670599, 0.04583333333333337173, 0.05000000000000004441, 0.05416666666666671709, 0.05833333333333338283 ),
 .UNSPECIFIED. ) 
 CURVE ( )  GEOMETRIC_REPRESENTATION_ITEM ( )  RATIONAL_B_SPLINE_CURVE ( ( 0.9999999999999992228, 0.9238795325112875156, 1.000000000000000000, 0.9238795325112867385, 1.000000000000000000, 0.9238795325112867385, 1.000000000000000000, 0.9238795325112858503, 1.000000000000000888 ) ) 
 REPRESENTATION_ITEM ( '' )  );
#9041=VECTOR ( 'NONE', #59064, 1000.000000000000000 ) ;
#9058=CARTESIAN_POINT ( 'NONE',  ( -50.55543936806279248, -134.3125000013656063, 0.3552334253322060320 ) ) ;
#9059=CARTESIAN_POINT ( 'NONE',  ( -58.24261429053147765, -140.3750000027312126, -3.805975901505573855 ) ) ;
#9065=CARTESIAN_POINT ( 'NONE',  ( -57.78304654714001742, -135.0000000000000853, -3.610108303323515511 ) ) ;
#9078=CARTESIAN_POINT ( 'NONE',  ( -59.98410592259440222, -144.2500000027312126, -0.3983568153799752487 ) ) ;
#9090=CARTESIAN_POINT ( 'NONE',  ( -52.80376928212989185, -143.1250000013656063, -4.297418129356379346 ) ) ;
#9101=LINE ( 'NONE', #43812, #21965 ) ;
#9108=CARTESIAN_POINT ( 'NONE',  ( -58.39396692619412477, -146.4375000013656063, 2.891590998281057701 ) ) ;
#9133=CARTESIAN_POINT ( 'NONE',  ( -58.39396692619412477, -149.6875000013656063, 2.891590998281057701 ) ) ;
#9172=CARTESIAN_POINT ( 'NONE',  ( -52.53715891517739323, -132.4375000000000284, -4.819101127000233298 ) ) ;
#9183=CARTESIAN_POINT ( 'NONE',  ( -55.39835681537999790, -125.0000000027311984, 4.984105922594378235 ) ) ;
#9185=CARTESIAN_POINT ( 'NONE',  ( -50.46537964183328029, -135.0000000000000284, 0.7220904342385146002 ) ) ;
#9190=CYLINDRICAL_SURFACE ( 'NONE', #1906, 5.000000000000000000 ) ;
#9206=CARTESIAN_POINT ( 'NONE',  ( -59.44456063193725015, -130.5625000013656063, -0.3552334253322034230 ) ) ;
#9207=CARTESIAN_POINT ( 'NONE',  ( -51.60603307380591787, -145.9375000013656063, -2.891590998281053704 ) ) ;
#9232=( BOUNDED_CURVE ( )  B_SPLINE_CURVE ( 2, ( #6614, #26227, #45847, #31358, #50999, #6939, #43533, #18480, #3385 ),
 .UNSPECIFIED., .F., .F. ) 
 B_SPLINE_CURVE_WITH_KNOTS ( ( 3, 2, 2, 2, 3 ),
 ( 0.5916666666666671182, 0.5958333333333335480, 0.6000000000000000888, 0.6041666666666665186, 0.6083333333333329485 ),
 .UNSPECIFIED. ) 
 CURVE ( )  GEOMETRIC_REPRESENTATION_ITEM ( )  RATIONAL_B_SPLINE_CURVE ( ( 0.9999999999999918954, 0.9238795325112948431, 1.000000000000000000, 0.9238795325112867385, 1.000000000000000000, 0.9238795325112867385, 1.000000000000000000, 0.9238795325112928447, 0.9999999999999938938 ) ) 
 REPRESENTATION_ITEM ( '' )  );
#9239=CARTESIAN_POINT ( 'NONE',  ( -56.48576386720575471, -152.0000000013655779, -4.591703134518078322 ) ) ;
#9248=CARTESIAN_POINT ( 'NONE',  ( -51.75738570946856498, -144.7500000000000284, 3.805975901505576964 ) ) ;
#9257=CARTESIAN_POINT ( 'NONE',  ( -51.60603307380591787, -152.1875000013656063, -2.891590998281053704 ) ) ;
#9258=CARTESIAN_POINT ( 'NONE',  ( -52.53715891517739323, -137.5625000027312126, -4.819101127000233298 ) ) ;
#9266=CARTESIAN_POINT ( 'NONE',  ( -51.19402409849444524, -139.6250000027312126, -3.242614290531456334 ) ) ;
#9267=CARTESIAN_POINT ( 'NONE',  ( -53.51423613279429503, -131.2500000013656347, 4.591703134518082763 ) ) ;
#9282=CARTESIAN_POINT ( 'NONE',  ( -57.19623071787017210, -142.3750000013656063, 4.297418129356382899 ) ) ;
#9302=LINE ( 'NONE', #28917, #61724 ) ;
#9313=ORIENTED_EDGE ( 'NONE', *, *, #14581, .F. ) ;
#9314=CARTESIAN_POINT ( 'NONE',  ( -57.19623071787016499, -153.3750000013656063, 4.297418129356382899 ) ) ;
#9321=CARTESIAN_POINT ( 'NONE',  ( -50.70258187064364108, -125.3750000013656205, 2.196230717870141014 ) ) ;
#9331=CARTESIAN_POINT ( 'NONE',  ( -55.39835681537999790, -152.0000000027312410, 4.984105922594378235 ) ) ;
#9337=CARTESIAN_POINT ( 'NONE',  ( -54.60164318462004474, -150.5000000027312126, -4.984105922594373794 ) ) ;
#9351=CARTESIAN_POINT ( 'NONE',  ( -52.10840900171896806, -152.1875000013656063, 3.393966926194110556 ) ) ;
#9353=CARTESIAN_POINT ( 'NONE',  ( 0.000000000000000000, -135.0000000000000284, 0.000000000000000000 ) ) ;
#9366=CARTESIAN_POINT ( 'NONE',  ( -58.39396692619412477, -130.6875000013656063, 2.891590998281057701 ) ) ;
#9374=CARTESIAN_POINT ( 'NONE',  ( -57.46284108482265651, -139.9375000000000284, 4.819101127000238627 ) ) ;
#9395=CARTESIAN_POINT ( 'NONE',  ( -50.70258187064364108, -138.3750000013656063, 2.196230717870141014 ) ) ;
#9400=CARTESIAN_POINT ( 'NONE',  ( -58.24261429053147765, -148.3750000027312126, -3.805975901505573855 ) ) ;
#9404=EDGE_LOOP ( 'NONE', ( #48405, #52607, #40576, #25148 ) ) ;
#9413=CARTESIAN_POINT ( 'NONE',  ( -59.59170313451811296, -145.5000000013656063, 1.485763867205729394 ) ) ;
#9416=ORIENTED_EDGE ( 'NONE', *, *, #51226, .F. ) ;
#9421=EDGE_CURVE ( 'NONE', #29717, #61181, #34507, .T. ) ;
#9439=CARTESIAN_POINT ( 'NONE',  ( -53.51423613279429503, -148.5000000013655779, 4.591703134518082763 ) ) ;
#9445=CARTESIAN_POINT ( 'NONE',  ( -59.98410592259440222, -136.2500000027312126, -0.3983568153799752487 ) ) ;
#9476=CARTESIAN_POINT ( 'NONE',  ( -50.18089887299979068, -131.6875000000000568, 2.462841084822635640 ) ) ;
#9485=CARTESIAN_POINT ( 'NONE',  ( -50.18089887299979068, -126.8125000027312126, 2.462841084822635640 ) ) ;
#9493=LINE ( 'NONE', #48110, #38152 ) ;
#9515=CARTESIAN_POINT ( 'NONE',  ( -57.89159099828107458, -128.6875000013656063, -3.393966926194107447 ) ) ;
#9516=CARTESIAN_POINT ( 'NONE',  ( -57.19623071787016499, -148.3750000013656063, 4.297418129356382899 ) ) ;
#9526=ORIENTED_EDGE ( 'NONE', *, *, #14600, .F. ) ;
#9552=CARTESIAN_POINT ( 'NONE',  ( -59.29741812935640155, -151.8750000013655779, -2.196230717870135685 ) ) ;
#9557=CARTESIAN_POINT ( 'NONE',  ( -58.39396692619412477, -135.4375000013656063, 2.891590998281057701 ) ) ;
#9562=CARTESIAN_POINT ( 'NONE',  ( -58.80597590150559739, -145.0000000000000284, 3.242614290531460330 ) ) ;
#9570=CARTESIAN_POINT ( 'NONE',  ( -55.35523342533222291, -144.5625000013656063, 4.444560631937231499 ) ) ;
#9571=CARTESIAN_POINT ( 'NONE',  ( -50.01589407740564042, -139.7500000027312126, 0.3983568153799778022 ) ) ;
#9582=CARTESIAN_POINT ( 'NONE',  ( -57.19623071787017210, -132.3750000013656347, 4.297418129356382899 ) ) ;
#9593=CARTESIAN_POINT ( 'NONE',  ( -50.01589407740564042, -143.7500000027312126, 0.3983568153799778022 ) ) ;
#9597=CARTESIAN_POINT ( 'NONE',  ( -54.64476657466781973, -142.8125000013656063, -4.444560631937228834 ) ) ;
#9601=CARTESIAN_POINT ( 'NONE',  ( -51.75738570946856498, -144.7500000000000284, 3.805975901505576964 ) ) ;
#9629=CARTESIAN_POINT ( 'NONE',  ( -57.19623071787016499, -152.3750000013656063, 4.297418129356382899 ) ) ;
#9636=CARTESIAN_POINT ( 'NONE',  ( -59.29741812935640155, -127.8750000013656063, -2.196230717870135685 ) ) ;
#9646=CARTESIAN_POINT ( 'NONE',  ( -60.14911071818854538, -149.1875000027312410, 1.666127454062681368 ) ) ;
#9649=DIRECTION ( 'NONE',  ( 0.8660254037844387076, 0.000000000000000000, -0.4999999999999998890 ) ) ;
#9679=LINE ( 'NONE', #3617, #30854 ) ;
#9696=ORIENTED_EDGE ( 'NONE', *, *, #42941, .F. ) ;
#9699=CARTESIAN_POINT ( 'NONE',  ( -58.24261429053147765, -136.2500000000000284, -3.805975901505573855 ) ) ;
#9708=CARTESIAN_POINT ( 'NONE',  ( -52.80376928212989185, -141.1250000013655779, -4.297418129356379346 ) ) ;
#9728=CARTESIAN_POINT ( 'NONE',  ( -57.89159099828107458, -143.6875000013656063, -3.393966926194107447 ) ) ;
#9731=ORIENTED_EDGE ( 'NONE', *, *, #8580, .F. ) ;
#9747=CARTESIAN_POINT ( 'NONE',  ( -51.75738570946856498, -154.7500000000000284, 3.805975901505576964 ) ) ;
#9750=CARTESIAN_POINT ( 'NONE',  ( -55.35523342533222291, -145.5625000013656063, 4.444560631937231499 ) ) ;
#9771=CYLINDRICAL_SURFACE ( 'NONE', #49995, 5.000000000000000000 ) ;
#9785=VERTEX_POINT ( 'NONE', #48604 ) ;
#9788=CARTESIAN_POINT ( 'NONE',  ( -56.66612745406270335, -135.3125000000000000, -5.149110718188516067 ) ) ;
#9798=CARTESIAN_POINT ( 'NONE',  ( -57.46284108482265651, -128.0625000027312410, 4.819101127000239515 ) ) ;
#9821=CARTESIAN_POINT ( 'NONE',  ( -51.60603307380591787, -126.9375000013656063, -2.891590998281053704 ) ) ;
#9822=CARTESIAN_POINT ( 'NONE',  ( -58.39396692619412477, -146.4375000013656063, 2.891590998281057701 ) ) ;
#9833=CARTESIAN_POINT ( 'NONE',  ( -59.44456063193725015, -125.8125000013655921, -0.3552334253322034230 ) ) ;
#9852=AXIS2_PLACEMENT_3D ( 'NONE', #2976, #3291, #62140 ) ;
#9855=EDGE_CURVE ( 'NONE', #4086, #44176, #59195, .T. ) ;
#9857=ORIENTED_EDGE ( 'NONE', *, *, #58262, .T. ) ;
#9858=CARTESIAN_POINT ( 'NONE',  ( -56.48576386720575471, -151.0000000013656063, -4.591703134518078322 ) ) ;
#9869=CARTESIAN_POINT ( 'NONE',  ( -56.66612745406270335, -144.3125000000000284, -5.149110718188516067 ) ) ;
#9880=CARTESIAN_POINT ( 'NONE',  ( -52.80376928212989185, -147.1250000013656063, -4.297418129356378458 ) ) ;
#9881=CARTESIAN_POINT ( 'NONE',  ( -51.75738570946856498, -139.8750000027312126, 3.805975901505576964 ) ) ;
#9893=CARTESIAN_POINT ( 'NONE',  ( -54.60164318462004474, -153.3750000000000284, -4.984105922594373794 ) ) ;
#9894=CARTESIAN_POINT ( 'NONE',  ( -51.60603307380591787, -132.9375000013656063, -2.891590998281053704 ) ) ;
#9904=CARTESIAN_POINT ( 'NONE',  ( -49.85088928181150436, -143.6875000027312126, -1.666127454062680480 ) ) ;
#9910=CARTESIAN_POINT ( 'NONE',  ( -58.39396692619412477, -142.4375000013656063, 2.891590998281057701 ) ) ;
#9919=DIRECTION ( 'NONE',  ( -0.6485228581062915110, 0.000000000000000000, -0.7611951803011149931 ) ) ;
#9941=CARTESIAN_POINT ( 'NONE',  ( -52.80376928212989185, -153.8750000013655779, -4.297418129356378458 ) ) ;
#9949=CARTESIAN_POINT ( 'NONE',  ( -52.80376928212989185, -127.1250000013656205, -4.297418129356379346 ) ) ;
#9957=CYLINDRICAL_SURFACE ( 'NONE', #23514, 5.000000000000000000 ) ;
#9963=CARTESIAN_POINT ( 'NONE',  ( -50.18089887299979068, -148.8125000027312126, 2.462841084822635640 ) ) ;
#9968=EDGE_CURVE ( 'NONE', #24283, #19422, #35343, .T. ) ;
#9983=CARTESIAN_POINT ( 'NONE',  ( -54.64476657466781973, -152.8125000013656063, -4.444560631937228834 ) ) ;
#10008=CARTESIAN_POINT ( 'NONE',  ( -59.65692920852630010, -135.0000000000000284, 1.510532900655110256 ) ) ;
#10031=CARTESIAN_POINT ( 'NONE',  ( -55.35523342533222291, -140.5625000013656063, 4.444560631937231499 ) ) ;
#10050=CARTESIAN_POINT ( 'NONE',  ( -51.60603307380591787, -141.9375000013656063, -2.891590998281053704 ) ) ;
#10068=CARTESIAN_POINT ( 'NONE',  ( -58.24261429053147765, -150.2500000000000284, -3.805975901505573855 ) ) ;
#10071=CARTESIAN_POINT ( 'NONE',  ( -50.18089887299979068, -154.6874999999999716, 2.462841084822631199 ) ) ;
#10075=CARTESIAN_POINT ( 'NONE',  ( -50.40829686548195099, -144.2500000013656063, -1.485763867205728284 ) ) ;
#10097=DIRECTION ( 'NONE',  ( 0.000000000000000000, 0.000000000000000000, 1.000000000000000000 ) ) ;
#10112=ORIENTED_EDGE ( 'NONE', *, *, #9421, .T. ) ;
#10118=CARTESIAN_POINT ( 'NONE',  ( -56.66612745406270335, -134.3125000000000284, -5.149110718188516067 ) ) ;
#10127=CARTESIAN_POINT ( 'NONE',  ( -54.64476657466781973, -151.8125000013656063, -4.444560631937228834 ) ) ;
#10130=VECTOR ( 'NONE', #30271, 1000.000000000000000 ) ;
#10153=CARTESIAN_POINT ( 'NONE',  ( -58.39396692619412477, -127.4375000013656063, 2.891590998281057701 ) ) ;
#10154=CARTESIAN_POINT ( 'NONE',  ( -50.40829686548195099, -146.0000000013656347, -1.485763867205728284 ) ) ;
#10190=CARTESIAN_POINT ( 'NONE',  ( -55.35523342533222291, -147.5625000013656063, 4.444560631937231499 ) ) ;
#10200=CARTESIAN_POINT ( 'NONE',  ( -59.81910112700025905, -147.1875000000000000, -2.462841084822630311 ) ) ;
#10209=CARTESIAN_POINT ( 'NONE',  ( -59.59170313451810586, -145.7500000013656063, 1.485763867205729394 ) ) ;
#10211=CARTESIAN_POINT ( 'NONE',  ( -49.85088928181150436, -139.6875000027312126, -1.666127454062680702 ) ) ;
#10217=ORIENTED_EDGE ( 'NONE', *, *, #24410, .T. ) ;
#10221=CARTESIAN_POINT ( 'NONE',  ( -51.60603307380591787, -131.9375000013656063, -2.891590998281053704 ) ) ;
#10238=CARTESIAN_POINT ( 'NONE',  ( -53.51423613279429503, -136.2500000013656063, 4.591703134518082763 ) ) ;
#10254=CARTESIAN_POINT ( 'NONE',  ( -58.80597590150559739, -153.1250000027312126, 3.242614290531460330 ) ) ;
#10272=CARTESIAN_POINT ( 'NONE',  ( -59.59170313451810586, -149.5000000013656063, 1.485763867205729394 ) ) ;
#10279=CARTESIAN_POINT ( 'NONE',  ( -59.59170313451811296, -125.7500000013656347, 1.485763867205729394 ) ) ;
#10286=ORIENTED_EDGE ( 'NONE', *, *, #35111, .T. ) ;
#10289=CARTESIAN_POINT ( 'NONE',  ( -54.60164318462004474, -152.5000000027312410, -4.984105922594373794 ) ) ;
#10305=CARTESIAN_POINT ( 'NONE',  ( -59.59170313451811296, -148.5000000013655779, 1.485763867205729394 ) ) ;
#10325=FACE_OUTER_BOUND ( 'NONE', #24768, .T. ) ;
#10330=EDGE_CURVE ( 'NONE', #55783, #24283, #26325, .T. ) ;
#10331=CARTESIAN_POINT ( 'NONE',  ( -58.24086726761811406, -135.0000000000000000, -3.252698689335780102 ) ) ;
#10335=EDGE_CURVE ( 'NONE', #40878, #41738, #43956, .T. ) ;
#10354=CARTESIAN_POINT ( 'NONE',  ( -50.55543936806279248, -138.3125000013656063, 0.3552334253322060320 ) ) ;
#10361=DIRECTION ( 'NONE',  ( -0.6485228581062915110, 0.000000000000000000, -0.7611951803011149931 ) ) ;
#10363=DIRECTION ( 'NONE',  ( -0.6485228581062915110, 0.000000000000000000, -0.7611951803011149931 ) ) ;
#10373=CARTESIAN_POINT ( 'NONE',  ( -57.19623071787017210, -139.3750000013656063, 4.297418129356382899 ) ) ;
#10374=CARTESIAN_POINT ( 'NONE',  ( -48.00000000000002132, -135.0000000000000284, -4.041451884327376121 ) ) ;
#10398=CARTESIAN_POINT ( 'NONE',  ( -57.19623071787017210, -142.6250000013655779, 4.297418129356382899 ) ) ;
#10418=CARTESIAN_POINT ( 'NONE',  ( -52.53715891517739323, -145.5625000027312126, -4.819101127000233298 ) ) ;
#10427=CARTESIAN_POINT ( 'NONE',  ( -52.53715891517739323, -137.4375000000000284, -4.819101127000233298 ) ) ;
#10435=CARTESIAN_POINT ( 'NONE',  ( -50.01589407740564042, -127.6250000000000142, 0.3983568153799778022 ) ) ;
#10442=CARTESIAN_POINT ( 'NONE',  ( -50.70258187064364108, -152.1250000013656063, 2.196230717870141014 ) ) ;
#10466=CARTESIAN_POINT ( 'NONE',  ( -53.51423613279429503, -125.2500000013656347, 4.591703134518082763 ) ) ;
#10467=CARTESIAN_POINT ( 'NONE',  ( -58.39396692619412477, -144.4375000013656063, 2.891590998281057701 ) ) ;
#10506=CARTESIAN_POINT ( 'NONE',  ( -57.46284108482265651, -140.9375000000000000, 4.819101127000239515 ) ) ;
#10511=SHAPE_DEFINITION_REPRESENTATION ( #34838, #49651 ) ;
#10516=CARTESIAN_POINT ( 'NONE',  ( -51.60603307380591787, -146.1875000013656063, -2.891590998281053704 ) ) ;
#10518=CARTESIAN_POINT ( 'NONE',  ( -58.24261429053147765, -134.3750000027312126, -3.805975901505573855 ) ) ;
#10532=CARTESIAN_POINT ( 'NONE',  ( -52.10840900171896806, -128.1875000013656063, 3.393966926194110556 ) ) ;
#10534=CARTESIAN_POINT ( 'NONE',  ( -58.24261429053147765, -141.2500000000000284, -3.805975901505573855 ) ) ;
#10544=CARTESIAN_POINT ( 'NONE',  ( -51.75738570946856498, -143.8750000027312126, 3.805975901505576964 ) ) ;
#10549=CARTESIAN_POINT ( 'NONE',  ( -55.35523342533222291, -138.3125000013656063, 4.444560631937231499 ) ) ;
#10556=CARTESIAN_POINT ( 'NONE',  ( -50.70258187064364108, -132.3750000013656347, 2.196230717870141014 ) ) ;
#10568=FACE_OUTER_BOUND ( 'NONE', #9404, .T. ) ;
#10580=CARTESIAN_POINT ( 'NONE',  ( -57.89159099828107458, -150.6875000013656063, -3.393966926194107447 ) ) ;
#10587=CARTESIAN_POINT ( 'NONE',  ( -60.14911071818854538, -152.0625000000000000, 1.666127454062681368 ) ) ;
#10598=CARTESIAN_POINT ( 'NONE',  ( -56.66612745406270335, -148.4375000027312126, -5.149110718188516067 ) ) ;
#10619=CARTESIAN_POINT ( 'NONE',  ( -50.40829686548195099, -148.0000000013655779, -1.485763867205728284 ) ) ;
#10621=CARTESIAN_POINT ( 'NONE',  ( -55.00000000000002132, -155.0000000000000284, 1.734723475976807094E-15 ) ) ;
#10624=PLANE ( 'NONE',  #38688 ) ;
#10644=ORIENTED_EDGE ( 'NONE', *, *, #42935, .F. ) ;
#10650=VECTOR ( 'NONE', #28561, 1000.000000000000000 ) ;
#10651=CARTESIAN_POINT ( 'NONE',  ( -54.60164318462004474, -147.5000000027312126, -4.984105922594373794 ) ) ;
#10666=CARTESIAN_POINT ( 'NONE',  ( -56.48576386720575471, -138.0000000013656063, -4.591703134518078322 ) ) ;
#10669=EDGE_CURVE ( 'NONE', #31572, #51345, #52299, .T. ) ;
#10670=ORIENTED_EDGE ( 'NONE', *, *, #9855, .F. ) ;
#10678=CARTESIAN_POINT ( 'NONE',  ( -50.18089887299976937, -140.6875000000000284, 2.462841084822397164 ) ) ;
#10685=ADVANCED_FACE ( 'NONE', ( #33299 ), #62271, .F. ) ;
#10691=CARTESIAN_POINT ( 'NONE',  ( -54.64476657466781973, -141.8125000013656063, -4.444560631937228834 ) ) ;
#10692=CARTESIAN_POINT ( 'NONE',  ( -58.80597590150559739, -155.0000000000000284, 3.242614290531457666 ) ) ;
#10701=CARTESIAN_POINT ( 'NONE',  ( -58.24261429053147765, -147.2500000000000284, -3.805975901505573855 ) ) ;
#10719=CARTESIAN_POINT ( 'NONE',  ( -57.89159099828107458, -144.9375000013656063, -3.393966926194107447 ) ) ;
#10759=CARTESIAN_POINT ( 'NONE',  ( -54.60164318462004474, -131.3750000000000284, -4.984105922594373794 ) ) ;
#10767=CARTESIAN_POINT ( 'NONE',  ( -57.89159099828107458, -151.6875000013656063, -3.393966926194107447 ) ) ;
#10781=CARTESIAN_POINT ( 'NONE',  ( -60.14911071818854538, -147.0625000000000000, 1.666127454062681146 ) ) ;
#10786=CARTESIAN_POINT ( 'NONE',  ( -58.24261429053147765, -146.2500000000000284, -3.805975901505573855 ) ) ;
#10792=CARTESIAN_POINT ( 'NONE',  ( -59.29741812935640155, -124.6250000013656347, -2.196230717870135685 ) ) ;
#10793=CARTESIAN_POINT ( 'NONE',  ( -52.80376928212989185, -143.8750000013655779, -4.297418129356378458 ) ) ;
#10830=CARTESIAN_POINT ( 'NONE',  ( -60.14911071818854538, -143.0625000000000284, 1.666127454062681368 ) ) ;
#10838=CARTESIAN_POINT ( 'NONE',  ( -52.10840900171896806, -147.4375000013656063, 3.393966926194110556 ) ) ;
#10840=CARTESIAN_POINT ( 'NONE',  ( -54.60164318462004474, -133.5000000027312126, -4.984105922594373794 ) ) ;
#10853=CARTESIAN_POINT ( 'NONE',  ( -53.51423613279429503, -129.2500000013656347, 4.591703134518082763 ) ) ;
#10868=CARTESIAN_POINT ( 'NONE',  ( -56.48576386720575471, -138.7500000013656063, -4.591703134518078322 ) ) ;
#10879=CARTESIAN_POINT ( 'NONE',  ( -57.19623071787017210, -133.6250000013655779, 4.297418129356382899 ) ) ;
#10891=CARTESIAN_POINT ( 'NONE',  ( -55.00000000000002132, -155.0000000000000284, 1.734723475976807094E-15 ) ) ;
#10904=CARTESIAN_POINT ( 'NONE',  ( -58.39396692619412477, -149.4375000013656063, 2.891590998281057701 ) ) ;
#10911=CARTESIAN_POINT ( 'NONE',  ( -53.33387254593733928, -151.8125000000000000, 5.149110718188519620 ) ) ;
#10914=CARTESIAN_POINT ( 'NONE',  ( -58.24261429053147765, -144.2500000000000284, -3.805975901505573855 ) ) ;
#10920=CARTESIAN_POINT ( 'NONE',  ( -60.14911071818854538, -147.1875000027312126, 1.666127454062681368 ) ) ;
#10935=CARTESIAN_POINT ( 'NONE',  ( -50.01589407740564042, -143.6250000000000284, 0.3983568153799778022 ) ) ;
#10937=CARTESIAN_POINT ( 'NONE',  ( -56.48576386720575471, -150.7500000013655495, -4.591703134518078322 ) ) ;
#10962=VERTEX_POINT ( 'NONE', #26188 ) ;
#10979=CARTESIAN_POINT ( 'NONE',  ( -59.81910112700026616, -141.3125000027312126, -2.462841084822451343 ) ) ;
#10986=CARTESIAN_POINT ( 'NONE',  ( -59.59170313451811296, -133.7500000013656063, 1.485763867205729394 ) ) ;
#10993=ORIENTED_EDGE ( 'NONE', *, *, #16118, .F. ) ;
#11003=CARTESIAN_POINT ( 'NONE',  ( -59.59170313451811296, -141.5000000013656063, 1.485763867205729394 ) ) ;
#11013=VECTOR ( 'NONE', #14799, 1000.000000000000000 ) ;
#11029=CARTESIAN_POINT ( 'NONE',  ( -53.51423613279429503, -142.5000000013656347, 4.591703134518082763 ) ) ;
#11051=DIRECTION ( 'NONE',  ( -0.6485228581062915110, 0.000000000000000000, -0.7611951803011149931 ) ) ;
#11064=VECTOR ( 'NONE', #54138, 1000.000000000000000 ) ;
#11070=CARTESIAN_POINT ( 'NONE',  ( -60.14911071818854538, -149.1875000027312410, 1.666127454062681146 ) ) ;
#11075=CARTESIAN_POINT ( 'NONE',  ( -53.33387254593733928, -129.8125000000000284, 5.149110718188519620 ) ) ;
#11082=CARTESIAN_POINT ( 'NONE',  ( -57.19623071787017210, -151.3750000013656063, 4.297418129356382899 ) ) ;
#11093=CARTESIAN_POINT ( 'NONE',  ( -55.39835681537999790, -146.8750000000000284, 4.984105922594378235 ) ) ;
#11106=CARTESIAN_POINT ( 'NONE',  ( -50.40829686548195099, -126.0000000013656063, -1.485763867205728284 ) ) ;
#11107=CARTESIAN_POINT ( 'NONE',  ( -50.40829686548195099, -142.0000000013656063, -1.485763867205728284 ) ) ;
#11137=ADVANCED_FACE ( 'NONE', ( #10325 ), #45377, .F. ) ;
#11149=CARTESIAN_POINT ( 'NONE',  ( -54.60164318462004474, -143.3750000000000284, -4.984105922594373794 ) ) ;
#11160=CARTESIAN_POINT ( 'NONE',  ( -59.29741812935640155, -142.8750000013656063, -2.196230717870135685 ) ) ;
#11162=CARTESIAN_POINT ( 'NONE',  ( -55.39835681537999790, -135.0000000027312126, 4.984105922594378235 ) ) ;
#11167=CARTESIAN_POINT ( 'NONE',  ( -60.14911071818853827, -135.0625000000000284, 1.666127454062502622 ) ) ;
#11174=CARTESIAN_POINT ( 'NONE',  ( -59.59170313451811296, -127.5000000013656347, 1.485763867205729394 ) ) ;
#11188=CARTESIAN_POINT ( 'NONE',  ( -59.29741812935640155, -136.6250000013655779, -2.196230717870135685 ) ) ;
#11197=ORIENTED_EDGE ( 'NONE', *, *, #56215, .F. ) ;
#11200=CARTESIAN_POINT ( 'NONE',  ( -54.64476657466781973, -130.0625000013656063, -4.444560631937228834 ) ) ;
#11203=AXIS2_PLACEMENT_3D ( 'NONE', #7218, #26831, #41598 ) ;
#11210=EDGE_LOOP ( 'NONE', ( #27929, #11417, #62261, #63600 ) ) ;
#11230=CARTESIAN_POINT ( 'NONE',  ( -53.33387254593733928, -153.8125000000000000, 5.149110718188519620 ) ) ;
#11241=CARTESIAN_POINT ( 'NONE',  ( -49.85088928181150436, -145.6875000027311842, -1.666127454062680702 ) ) ;
#11259=CARTESIAN_POINT ( 'NONE',  ( -52.10840900171896806, -150.1875000013656063, 3.393966926194110556 ) ) ;
#11277=DIRECTION ( 'NONE',  ( 0.6485228581062915110, 0.000000000000000000, 0.7611951803011149931 ) ) ;
#11302=CARTESIAN_POINT ( 'NONE',  ( -51.60603307380591787, -136.1875000013656063, -2.891590998281053704 ) ) ;
#11324=FACE_OUTER_BOUND ( 'NONE', #55623, .T. ) ;
#11349=CARTESIAN_POINT ( 'NONE',  ( -50.40829686548195099, -140.2500000013656063, -1.485763867205728284 ) ) ;
#11366=CARTESIAN_POINT ( 'NONE',  ( -53.51423613279429503, -136.5000000013656063, 4.591703134518083651 ) ) ;
#11380=CARTESIAN_POINT ( 'NONE',  ( -59.59170313451811296, -145.7500000013655779, 1.485763867205729394 ) ) ;
#11390=CARTESIAN_POINT ( 'NONE',  ( -57.46284108482265651, -128.9375000000000284, 4.819101127000239515 ) ) ;
#11400=CARTESIAN_POINT ( 'NONE',  ( -50.70258187064364108, -154.1250000013656347, 2.196230717870141014 ) ) ;
#11417=ORIENTED_EDGE ( 'NONE', *, *, #49475, .T. ) ;
#11426=CARTESIAN_POINT ( 'NONE',  ( -51.60603307380591787, -152.1875000013656063, -2.891590998281053704 ) ) ;
#11428=CARTESIAN_POINT ( 'NONE',  ( -53.51423613279429503, -142.2500000013656063, 4.591703134518083651 ) ) ;
#11458=VERTEX_POINT ( 'NONE', #20943 ) ;
#11464=AXIS2_PLACEMENT_3D ( 'NONE', #45836, #41625, #50662 ) ;
#11465=CARTESIAN_POINT ( 'NONE',  ( -56.66612745406270335, -140.3125000000000284, -5.149110718188516067 ) ) ;
#11473=CARTESIAN_POINT ( 'NONE',  ( -51.75738570946856498, -136.8750000027312126, 3.805975901505576964 ) ) ;
#11477=CARTESIAN_POINT ( 'NONE',  ( -50.70258187064364108, -142.3750000013656063, 2.196230717870141014 ) ) ;
#11479=CARTESIAN_POINT ( 'NONE',  ( -50.01589407740564042, -134.7500000027312126, 0.3983568153799778022 ) ) ;
#11495=CARTESIAN_POINT ( 'NONE',  ( -57.19623071787017210, -127.3750000013656205, 4.297418129356382899 ) ) ;
#11509=CARTESIAN_POINT ( 'NONE',  ( -52.80376928212989185, -137.8750000013655779, -4.297418129356379346 ) ) ;
#11519=CARTESIAN_POINT ( 'NONE',  ( -52.10840900171896806, -133.4375000013656063, 3.393966926194110556 ) ) ;
#11538=VERTEX_POINT ( 'NONE', #52968 ) ;
#11546=DIRECTION ( 'NONE',  ( 0.000000000000000000, 1.000000000000000000, 0.000000000000000000 ) ) ;
#11550=CARTESIAN_POINT ( 'NONE',  ( -51.19402409849444524, -154.5000000000000284, -3.242614290531456334 ) ) ;
#11558=CARTESIAN_POINT ( 'NONE',  ( -55.35523342533222291, -152.5625000013656063, 4.444560631937231499 ) ) ;
#11560=CARTESIAN_POINT ( 'NONE',  ( -57.46284108482265651, -148.0625000027312126, 4.819101127000239515 ) ) ;
#11578=CARTESIAN_POINT ( 'NONE',  ( -54.64476657466781973, -149.8125000013656063, -4.444560631937228834 ) ) ;
#11593=CARTESIAN_POINT ( 'NONE',  ( -58.24261429053147765, -152.3750000027312126, -3.805975901505573855 ) ) ;
#11620=CARTESIAN_POINT ( 'NONE',  ( -52.10840900171896806, -136.4375000013656063, 3.393966926194110556 ) ) ;
#11625=CARTESIAN_POINT ( 'NONE',  ( -54.93493926172311603, -135.0000000000000000, -4.467806258561277666 ) ) ;
#11626=ORIENTED_EDGE ( 'NONE', *, *, #5172, .T. ) ;
#11660=CARTESIAN_POINT ( 'NONE',  ( -56.48576386720575471, -141.0000000013656063, -4.591703134518078322 ) ) ;
#11677=EDGE_CURVE ( 'NONE', #16288, #17633, #58428, .T. ) ;
#11689=CARTESIAN_POINT ( 'NONE',  ( -58.24261429053147765, -135.3750000027312410, -3.805975901505573855 ) ) ;
#11693=CARTESIAN_POINT ( 'NONE',  ( -58.39396692619412477, -145.6875000013656063, 2.891590998281057701 ) ) ;
#11706=CARTESIAN_POINT ( 'NONE',  ( -58.24261429053147765, -127.2500000000000284, -3.805975901505573855 ) ) ;
#11714=CARTESIAN_POINT ( 'NONE',  ( -59.44456063193725015, -149.5625000013656063, -0.3552334253322034230 ) ) ;
#11722=CARTESIAN_POINT ( 'NONE',  ( -51.75738570946856498, -152.8750000027312126, 3.805975901505576964 ) ) ;
#11736=CARTESIAN_POINT ( 'NONE',  ( -54.64476657466781973, -150.0625000013656063, -4.444560631937228834 ) ) ;
#11737=CARTESIAN_POINT ( 'NONE',  ( -59.29741812935640155, -143.6250000013655779, -2.196230717870135685 ) ) ;
#11740=CARTESIAN_POINT ( 'NONE',  ( -54.60164318462004474, -153.5000000027312410, -4.984105922594373794 ) ) ;
#11749=CARTESIAN_POINT ( 'NONE',  ( -58.80597590150559739, -136.0000000000000284, 3.242614290531460330 ) ) ;
#11776=CARTESIAN_POINT ( 'NONE',  ( -55.39835681537999790, -140.8750000000000284, 4.984105922594378235 ) ) ;
#11786=CARTESIAN_POINT ( 'NONE',  ( -50.40829686548195099, -143.2500000013656063, -1.485763867205728284 ) ) ;
#11788=CARTESIAN_POINT ( 'NONE',  ( -51.19402409849444524, -133.6250000027312126, -3.242614290531456334 ) ) ;
#11803=CARTESIAN_POINT ( 'NONE',  ( -53.51423613279429503, -130.2500000013656063, 4.591703134518082763 ) ) ;
#11814=CARTESIAN_POINT ( 'NONE',  ( -52.80376928212989185, -132.8750000013656063, -4.297418129356379346 ) ) ;
#11824=CARTESIAN_POINT ( 'NONE',  ( -53.51423613279429503, -128.5000000013656063, 4.591703134518082763 ) ) ;
#11839=CARTESIAN_POINT ( 'NONE',  ( -51.75738570946856498, -138.8750000027312126, 3.805975901505576964 ) ) ;
#11851=ORIENTED_EDGE ( 'NONE', *, *, #31628, .F. ) ;
#11853=CARTESIAN_POINT ( 'NONE',  ( -54.64476657466781973, -137.8125000013656063, -4.444560631937228834 ) ) ;
#11860=CARTESIAN_POINT ( 'NONE',  ( -51.75738570946856498, -154.7500000000000284, 3.805975901505576964 ) ) ;
#11870=CARTESIAN_POINT ( 'NONE',  ( -49.85088928181150436, -147.6875000027311557, -1.666127454062680702 ) ) ;
#11883=ORIENTED_EDGE ( 'NONE', *, *, #17664, .T. ) ;
#11891=CARTESIAN_POINT ( 'NONE',  ( -57.89159099828107458, -147.6875000013656063, -3.393966926194107447 ) ) ;
#11908=CARTESIAN_POINT ( 'NONE',  ( -57.46284108482265651, -152.0625000027312410, 4.819101127000238627 ) ) ;
#11923=ORIENTED_EDGE ( 'NONE', *, *, #22427, .T. ) ;
#11935=ADVANCED_FACE ( 'NONE', ( #18878, #4105 ), #24981, .T. ) ;
#11937=CARTESIAN_POINT ( 'NONE',  ( -59.29741812935640155, -133.8750000013656063, -2.196230717870135685 ) ) ;
#11941=EDGE_CURVE ( 'NONE', #19205, #38280, #44265, .T. ) ;
#11955=CARTESIAN_POINT ( 'NONE',  ( -53.33387254593723981, -146.9375000027312126, 5.149110718188528502 ) ) ;
#11960=VERTEX_POINT ( 'NONE', #34300 ) ;
#11968=CARTESIAN_POINT ( 'NONE',  ( -55.00000000000002132, -155.0000000000000284, 1.734723475976807094E-15 ) ) ;
#11981=CARTESIAN_POINT ( 'NONE',  ( -52.10840900171896806, -141.4375000013656063, 3.393966926194110556 ) ) ;
#12013=CARTESIAN_POINT ( 'NONE',  ( -53.51423613279429503, -145.5000000013656063, 4.591703134518082763 ) ) ;
#12018=ORIENTED_EDGE ( 'NONE', *, *, #34127, .F. ) ;
#12036=CARTESIAN_POINT ( 'NONE',  ( -50.70258187064364108, -148.1250000013656063, 2.196230717870141014 ) ) ;
#12060=CARTESIAN_POINT ( 'NONE',  ( -59.44456063193725015, -152.8125000013656063, -0.3552334253322034230 ) ) ;
#12100=ORIENTED_EDGE ( 'NONE', *, *, #36538, .F. ) ;
#12101=CARTESIAN_POINT ( 'NONE',  ( -51.75738570946856498, -137.7500000000000000, 3.805975901505576964 ) ) ;
#12109=CARTESIAN_POINT ( 'NONE',  ( -59.59170313451810586, -143.7500000013656063, 1.485763867205729394 ) ) ;
#12111=CARTESIAN_POINT ( 'NONE',  ( -55.39835681537999790, -129.0000000027312126, 4.984105922594378235 ) ) ;
#12126=CARTESIAN_POINT ( 'NONE',  ( -52.80376928212989185, -126.8750000013656205, -4.297418129356379346 ) ) ;
#12131=ORIENTED_EDGE ( 'NONE', *, *, #52293, .T. ) ;
#12140=CARTESIAN_POINT ( 'NONE',  ( -57.19623071787017210, -132.3750000013656347, 4.297418129356382899 ) ) ;
#12152=CARTESIAN_POINT ( 'NONE',  ( -58.39396692619412477, -126.6875000013656063, 2.891590998281057701 ) ) ;
#12183=CARTESIAN_POINT ( 'NONE',  ( -52.10840900171896806, -139.1875000013656347, 3.393966926194110556 ) ) ;
#12188=CARTESIAN_POINT ( 'NONE',  ( -49.85088928181150436, -149.5625000000000284, -1.666127454062680702 ) ) ;
#12196=CARTESIAN_POINT ( 'NONE',  ( -50.70258187064364108, -154.3750000013656063, 2.196230717870141014 ) ) ;
#12197=CARTESIAN_POINT ( 'NONE',  ( -55.39835681537999790, -142.0000000027312126, 4.984105922594378235 ) ) ;
#12207=CARTESIAN_POINT ( 'NONE',  ( -57.89159099828107458, -142.6875000013656063, -3.393966926194107447 ) ) ;
#12223=CARTESIAN_POINT ( 'NONE',  ( -54.64476657466781973, -143.8125000013656063, -4.444560631937228834 ) ) ;
#12258=EDGE_LOOP ( 'NONE', ( #32755, #24926, #5046, #37631, #62958, #34712 ) ) ;
#12269=CARTESIAN_POINT ( 'NONE',  ( -59.44456063193725015, -133.8125000013656063, -0.3552334253322034230 ) ) ;
#12285=CARTESIAN_POINT ( 'NONE',  ( -51.75738570946856498, -146.8750000027312126, 3.805975901505576964 ) ) ;
#12306=CARTESIAN_POINT ( 'NONE',  ( -52.10840900171896806, -152.1875000013656063, 3.393966926194110556 ) ) ;
#12312=AXIS2_PLACEMENT_3D ( 'NONE', #31139, #17301, #41102 ) ;
#12315=CARTESIAN_POINT ( 'NONE',  ( -50.55543936806279248, -139.3125000013656063, 0.3552334253322060320 ) ) ;
#12333=CARTESIAN_POINT ( 'NONE',  ( -52.80376928212989185, -136.1250000013656063, -4.297418129356378458 ) ) ;
#12344=CARTESIAN_POINT ( 'NONE',  ( -52.80376928212989185, -149.1250000013656063, -4.297418129356379346 ) ) ;
#12355=CARTESIAN_POINT ( 'NONE',  ( -49.85088928181150436, -127.5625000000000284, -1.666127454062680702 ) ) ;
#12362=CARTESIAN_POINT ( 'NONE',  ( -59.59170313451811296, -149.5000000013655779, 1.485763867205729394 ) ) ;
#12387=CARTESIAN_POINT ( 'NONE',  ( -55.35523342533222291, -153.5625000013656063, 4.444560631937231499 ) ) ;
#12407=DIRECTION ( 'NONE',  ( 0.000000000000000000, 1.000000000000000000, 0.000000000000000000 ) ) ;
#12410=ORIENTED_EDGE ( 'NONE', *, *, #56136, .T. ) ;
#12420=( BOUNDED_CURVE ( )  B_SPLINE_CURVE ( 2, ( #50634, #59979, #54823, #45484, #40656, #44840, #40973, #804, #59656 ),
 .UNSPECIFIED., .F., .F. ) 
 B_SPLINE_CURVE_WITH_KNOTS ( ( 3, 2, 2, 2, 3 ),
 ( 0.4416666666666670404, 0.4458333333333337478, 0.4500000000000003997, 0.4541666666666671071, 0.4583333333333337589 ),
 .UNSPECIFIED. ) 
 CURVE ( )  GEOMETRIC_REPRESENTATION_ITEM ( )  RATIONAL_B_SPLINE_CURVE ( ( 0.9999999999999928946, 0.9238795325112938439, 1.000000000000000000, 0.9238795325112867385, 1.000000000000000000, 0.9238795325112867385, 1.000000000000000000, 0.9238795325112786339, 1.000000000000008216 ) ) 
 REPRESENTATION_ITEM ( '' )  );
#12425=CARTESIAN_POINT ( 'NONE',  ( -54.60164318462004474, -136.3750000000000284, -4.984105922594373794 ) ) ;
#12433=CARTESIAN_POINT ( 'NONE',  ( -59.44456063193725015, -141.8125000013656063, -0.3552334253322034230 ) ) ;
#12435=CARTESIAN_POINT ( 'NONE',  ( -58.80597590150559739, -131.1250000027312126, 3.242614290531460330 ) ) ;
#12447=CARTESIAN_POINT ( 'NONE',  ( -56.48576386720575471, -126.7500000013655921, -4.591703134518078322 ) ) ;
#12448=( BOUNDED_CURVE ( )  B_SPLINE_CURVE ( 2, ( #50212, #16122, #1666, #54730, #1037, #59886, #10651, #5838, #25450 ),
 .UNSPECIFIED., .F., .F. ) 
 B_SPLINE_CURVE_WITH_KNOTS ( ( 3, 2, 2, 2, 3 ),
 ( 0.2083333333333335091, 0.2125000000000001610, 0.2166666666666668406, 0.2208333333333335202, 0.2250000000000001998 ),
 .UNSPECIFIED. ) 
 CURVE ( )  GEOMETRIC_REPRESENTATION_ITEM ( )  RATIONAL_B_SPLINE_CURVE ( ( 0.9999999999999970024, 0.9238795325112897361, 1.000000000000000000, 0.9238795325112867385, 1.000000000000000000, 0.9238795325112867385, 1.000000000000000000, 0.9238795325112831858, 1.000000000000003553 ) ) 
 REPRESENTATION_ITEM ( '' )  );
#12460=CARTESIAN_POINT ( 'NONE',  ( -56.48576386720575471, -134.7500000013656063, -4.591703134518078322 ) ) ;
#12471=CARTESIAN_POINT ( 'NONE',  ( -54.64476657466781973, -127.0625000013655921, -4.444560631937228834 ) ) ;
#12497=CARTESIAN_POINT ( 'NONE',  ( -52.10840900171896806, -138.1875000013656347, 3.393966926194110556 ) ) ;
#12502=CARTESIAN_POINT ( 'NONE',  ( -50.01589407740564042, -149.6250000000000284, 0.3983568153799778022 ) ) ;
#12506=CARTESIAN_POINT ( 'NONE',  ( -51.75738570946856498, -150.7500000000000284, 3.805975901505576964 ) ) ;
#12512=CARTESIAN_POINT ( 'NONE',  ( -52.10840900171896806, -153.4375000013656063, 3.393966926194110556 ) ) ;
#12513=CARTESIAN_POINT ( 'NONE',  ( -60.14911071818854538, -143.1875000027312126, 1.666127454062681368 ) ) ;
#12520=CARTESIAN_POINT ( 'NONE',  ( -59.44456063193725015, -136.5625000013656063, -0.3552334253322034230 ) ) ;
#12526=VERTEX_POINT ( 'NONE', #2458 ) ;
#12534=CARTESIAN_POINT ( 'NONE',  ( -50.70258187064364108, -146.1250000013656063, 2.196230717870141014 ) ) ;
#12561=( BOUNDED_CURVE ( )  B_SPLINE_CURVE ( 2, ( #39211, #14452, #57601, #58836, #14765, #33762, #13528, #34383, #18961, #9941, #29556, #33147, #9006, #52762, #8691, #13830, #49190, #9314, #3875, #58208, #4191, #24430, #14135, #4806, #53381, #23494, #48551, #314, #23804, #58528, #63051, #43406, #62737, #9629, #19278, #5128, #12306, #28928, #4490, #44032, #37968, #24118, #18659, #57906, #34074, #48862, #633, #970, #15423, #44673, #5445, #25710, #15737, #39526, #54657, #39845, #20243, #59488, #35354, #35045, #10580, #60131, #30519, #19912, #30192, #16052, #45004, #54975, #49821, #45322, #5765, #59164, #25383, #54339, #1289, #20572, #15096, #40178, #59815, #10272, #10904, #50142, #55308, #6097, #34713, #29876, #20887, #35680, #40490, #49506, #25063, #14344, #23701, #19484, #8894, #24000, #20128, #9516, #52956, #24310, #19801, #5337, #29759, #48127, #39409, #49393, #63564, #28820, #34584, #4078, #48441, #58726, #24955, #39728, #29123, #33654, #203, #28509, #59048, #4381, #14652, #39097, #34271, #49066, #43298, #53897, #44560, #54216, #9822, #62934, #29433, #53272, #18848, #14976, #43917, #10154, #9207, #5013, #517, #38469, #14025, #13716, #58095, #33340, #24632, #43602, #63246, #44239, #19160, #38778, #4688, #58417, #33966, #53586, #48746, #49710, #45844, #15941, #26224, #40376, #10467, #16580, #55187, #15301, #41013, #60017, #36200, #60656, #34923, #10793, #30079, #5655, #35243, #11737, #30732, #25267, #35563, #6936, #59695, #31355, #25906, #55821, #16265, #55513, #40692, #26547, #15626, #50996, #21088, #46167, #44888, #54862, #50028, #54544, #849, #11428, #2129, #1806, #59367, #11107, #21730, #31045, #20452, #40051, #50354, #6301, #30405, #5986, #25591, #45204, #1171, #21410, #20771, #45524, #1485, #60337, #35883, #50670, #6611, #16695, #17327, #12811, #61088, #26980, #17947, #46599, #55938, #51745, #41122, #56258, #52378, #41753, #21526, #56575, #52061, #8315, #57212, #36626, #61718, #41439, #36949, #17010, #3177, #36314, #12183, #27293, #62030, #45956, #61403, #2239, #32432, #60770, #7999, #31797, #46918, #13131, #1921, #32109, #27602, #51429, #12497, #22797, #2860, #31471, #22482, #21843, #11853, #47235, #7687, #7372, #42077, #2543, #22159, #51112, #17647, #37263, #37572, #42390, #56891, #32750, #7049, #26662, #46280, #39136, #28227, #43954, #58132, #43026, #14063, #52990, #23423, #47843, #29162, #24041, #47537, #48164, #38210, #62666, #57835, #63284, #8931, #13754, #8619, #23101, #9557, #28544, #14379, #43643, #13446, #62348, #4117, #23737, #18269 ),
 .UNSPECIFIED., .F., .F. ) 
 B_SPLINE_CURVE_WITH_KNOTS ( ( 3, 2, 2, 2, 2, 2, 2, 2, 2, 2, 2, 2, 2, 2, 2, 2, 2, 2, 2, 2, 2, 2, 2, 2, 2, 2, 2, 2, 2, 2, 2, 2, 2, 2, 2, 2, 2, 2, 2, 2, 2, 2, 2, 2, 2, 2, 2, 2, 2, 2, 2, 2, 2, 2, 2, 2, 2, 2, 2, 2, 2, 2, 2, 2, 2, 2, 2, 2, 2, 2, 2, 2, 2, 2, 2, 2, 2, 2, 2, 2, 2, 2, 2, 2, 2, 2, 2, 2, 2, 2, 2, 2, 2, 2, 2, 2, 2, 2, 2, 2, 2, 2, 2, 2, 2, 2, 2, 2, 2, 2, 2, 2, 2, 2, 2, 2, 2, 2, 2, 2, 2, 2, 2, 2, 2, 2, 2, 2, 2, 2, 2, 2, 2, 2, 2, 2, 2, 2, 2, 2, 2, 2, 2, 2, 2, 2, 2, 2, 2, 2, 2, 2, 2, 2, 2, 2, 3 ),
 ( 0.000000000000000000, 0.004166666666666666609, 0.008333333333333333218, 0.01250000000000000243, 0.01666666666666666644, 0.02083333333333333218, 0.02500000000000000486, 0.02916666666666666713, 0.03333333333333333287, 0.03749999999999999861, 0.04166666666666666435, 0.04583333333333333010, 0.05000000000000000971, 0.05416666666666666852, 0.05833333333333333426, 0.06250000000000000000, 0.06666666666666666574, 0.07083333333333333148, 0.07499999999999999722, 0.07916666666666666297, 0.08333333333333332871, 0.08749999999999999445, 0.09166666666666666019, 0.09583333333333333981, 0.1000000000000000194, 0.1041666666666666713, 0.1083333333333333370, 0.1124999999999999889, 0.1166666666666666685, 0.1208333333333333204, 0.1250000000000000000, 0.1291666666666666796, 0.1333333333333333315, 0.1375000000000000111, 0.1416666666666666630, 0.1458333333333333426, 0.1499999999999999944, 0.1541666666666666741, 0.1583333333333333259, 0.1625000000000000056, 0.1666666666666666574, 0.1708333333333333370, 0.1749999999999999889, 0.1791666666666666685, 0.1833333333333333204, 0.1875000000000000000, 0.1916666666666666796, 0.1958333333333333315, 0.2000000000000000389, 0.2041666666666666907, 0.2083333333333333426, 0.2124999999999999944, 0.2166666666666666741, 0.2208333333333333259, 0.2249999999999999778, 0.2291666666666666574, 0.2333333333333333370, 0.2374999999999999889, 0.2416666666666666408, 0.2458333333333332926, 0.2500000000000000000, 0.2541666666666666519, 0.2583333333333333592, 0.2625000000000000111, 0.2666666666666666630, 0.2708333333333333148, 0.2750000000000000222, 0.2791666666666666741, 0.2833333333333333259, 0.2874999999999999778, 0.2916666666666666852, 0.2958333333333333370, 0.2999999999999999889, 0.3041666666666666408, 0.3083333333333333481, 0.3125000000000000000, 0.3166666666666666519, 0.3208333333333333592, 0.3250000000000000111, 0.3291666666666666630, 0.3333333333333333148, 0.3375000000000000222, 0.3416666666666666741, 0.3458333333333333259, 0.3499999999999999778, 0.3541666666666666852, 0.3583333333333333370, 0.3624999999999999889, 0.3666666666666666408, 0.3708333333333333481, 0.3750000000000000000, 0.3791666666666666519, 0.3833333333333333592, 0.3875000000000000111, 0.3916666666666666630, 0.3958333333333333148, 0.4000000000000000777, 0.4041666666666667296, 0.4083333333333333814, 0.4125000000000000333, 0.4166666666666666852, 0.4208333333333333370, 0.4249999999999999889, 0.4291666666666666408, 0.4333333333333333481, 0.4375000000000000000, 0.4416666666666666519, 0.4458333333333333037, 0.4499999999999999556, 0.4541666666666666630, 0.4583333333333333148, 0.4625000000000000222, 0.4666666666666666741, 0.4708333333333333259, 0.4749999999999999778, 0.4791666666666666297, 0.4833333333333332815, 0.4874999999999999334, 0.4916666666666665853, 0.4958333333333333481, 0.5000000000000000000, 0.5041666666666666519, 0.5083333333333333037, 0.5124999999999999556, 0.5166666666666667185, 0.5208333333333333703, 0.5250000000000000222, 0.5291666666666666741, 0.5333333333333333259, 0.5374999999999999778, 0.5416666666666666297, 0.5458333333333332815, 0.5500000000000000444, 0.5541666666666666963, 0.5583333333333333481, 0.5625000000000000000, 0.5666666666666666519, 0.5708333333333333037, 0.5749999999999999556, 0.5791666666666667185, 0.5833333333333333703, 0.5875000000000000222, 0.5916666666666666741, 0.5958333333333333259, 0.5999999999999999778, 0.6041666666666666297, 0.6083333333333332815, 0.6125000000000000444, 0.6166666666666666963, 0.6208333333333333481, 0.6250000000000000000, 0.6291666666666666519, 0.6333333333333333037, 0.6374999999999999556, 0.6416666666666667185, 0.6458333333333333703, 0.6479166667104350186 ),
 .UNSPECIFIED. ) 
 CURVE ( )  GEOMETRIC_REPRESENTATION_ITEM ( )  RATIONAL_B_SPLINE_CURVE ( ( 1.000000000000000000, 0.9238795325112867385, 1.000000000000000000, 0.9238795325112867385, 1.000000000000000000, 0.9238795325112867385, 1.000000000000000000, 0.9238795325112867385, 1.000000000000000000, 0.9238795325112867385, 1.000000000000000000, 0.9238795325112867385, 1.000000000000000000, 0.9238795325112867385, 1.000000000000000000, 0.9238795325112867385, 1.000000000000000000, 0.9238795325112867385, 1.000000000000000000, 0.9238795325112867385, 1.000000000000000000, 0.9238795325112867385, 1.000000000000000000, 0.9238795325112867385, 1.000000000000000000, 0.9238795325112867385, 1.000000000000000000, 0.9238795325112867385, 1.000000000000000000, 0.9238795325112867385, 1.000000000000000000, 0.9238795325112867385, 1.000000000000000000, 0.9238795325112867385, 1.000000000000000000, 0.9238795325112867385, 1.000000000000000000, 0.9238795325112867385, 1.000000000000000000, 0.9238795325112867385, 1.000000000000000000, 0.9238795325112867385, 1.000000000000000000, 0.9238795325112867385, 1.000000000000000000, 0.9238795325112867385, 1.000000000000000000, 0.9238795325112867385, 1.000000000000000000, 0.9238795325112867385, 1.000000000000000000, 0.9238795325112867385, 1.000000000000000000, 0.9238795325112867385, 1.000000000000000000, 0.9238795325112867385, 1.000000000000000000, 0.9238795325112867385, 1.000000000000000000, 0.9238795325112867385, 1.000000000000000000, 0.9238795325112867385, 1.000000000000000000, 0.9238795325112867385, 1.000000000000000000, 0.9238795325112867385, 1.000000000000000000, 0.9238795325112867385, 1.000000000000000000, 0.9238795325112867385, 1.000000000000000000, 0.9238795325112867385, 1.000000000000000000, 0.9238795325112867385, 1.000000000000000000, 0.9238795325112867385, 1.000000000000000000, 0.9238795325112867385, 1.000000000000000000, 0.9238795325112867385, 1.000000000000000000, 0.9238795325112867385, 1.000000000000000000, 0.9238795325112867385, 1.000000000000000000, 0.9238795325112867385, 1.000000000000000000, 0.9238795325112867385, 1.000000000000000000, 0.9238795325112867385, 1.000000000000000000, 0.9238795325112867385, 1.000000000000000000, 0.9238795325112867385, 1.000000000000000000, 0.9238795325112867385, 1.000000000000000000, 0.9238795325112867385, 1.000000000000000000, 0.9238795325112867385, 1.000000000000000000, 0.9238795325112867385, 1.000000000000000000, 0.9238795325112867385, 1.000000000000000000, 0.9238795325112867385, 1.000000000000000000, 0.9238795325112867385, 1.000000000000000000, 0.9238795325112867385, 1.000000000000000000, 0.9238795325112867385, 1.000000000000000000, 0.9238795325112867385, 1.000000000000000000, 0.9238795325112867385, 1.000000000000000000, 0.9238795325112867385, 1.000000000000000000, 0.9238795325112867385, 1.000000000000000000, 0.9238795325112867385, 1.000000000000000000, 0.9238795325112867385, 1.000000000000000000, 0.9238795325112867385, 1.000000000000000000, 0.9238795325112867385, 1.000000000000000000, 0.9238795325112867385, 1.000000000000000000, 0.9238795325112867385, 1.000000000000000000, 0.9238795325112867385, 1.000000000000000000, 0.9238795325112867385, 1.000000000000000000, 0.9238795325112867385, 1.000000000000000000, 0.9238795325112867385, 1.000000000000000000, 0.9238795325112867385, 1.000000000000000000, 0.9238795325112867385, 1.000000000000000000, 0.9238795325112867385, 1.000000000000000000, 0.9238795325112867385, 1.000000000000000000, 0.9238795325112867385, 1.000000000000000000, 0.9238795325112867385, 1.000000000000000000, 0.9238795325112867385, 1.000000000000000000, 0.9238795325112867385, 1.000000000000000000, 0.9238795325112867385, 1.000000000000000000, 0.9238795325112867385, 1.000000000000000000, 0.9238795325112867385, 1.000000000000000000, 0.9238795325112867385, 1.000000000000000000, 0.9238795325112867385, 1.000000000000000000, 0.9238795325112867385, 1.000000000000000000, 0.9238795325112867385, 1.000000000000000000, 0.9238795325112867385, 1.000000000000000000, 0.9238795325112867385, 1.000000000000000000, 0.9238795325112867385, 1.000000000000000000, 0.9238795325112867385, 1.000000000000000000, 0.9238795325112867385, 1.000000000000000000, 0.9238795325112867385, 1.000000000000000000, 0.9238795325112867385, 1.000000000000000000, 0.9238795325112867385, 1.000000000000000000, 0.9238795325112867385, 1.000000000000000000, 0.9238795325112867385, 1.000000000000000000, 0.9238795325112867385, 1.000000000000000000, 0.9238795325112867385, 1.000000000000000000, 0.9238795325112867385, 1.000000000000000000, 0.9238795325112867385, 1.000000000000000000, 0.9238795325112867385, 1.000000000000000000, 0.9238795325112867385, 1.000000000000000000, 0.9238795325112867385, 1.000000000000000000, 0.9238795325112867385, 1.000000000000000000, 0.9238795325112867385, 1.000000000000000000, 0.9238795325112867385, 1.000000000000000000, 0.9238795325112867385, 1.000000000000000000, 0.9238795325112867385, 1.000000000000000000, 0.9238795325112867385, 1.000000000000000000, 0.9238795325112867385, 1.000000000000000000, 0.9238795325112867385, 1.000000000000000000, 0.9238795325112867385, 1.000000000000000000, 0.9238795325112867385, 1.000000000000000000, 0.9238795325112867385, 1.000000000000000000, 0.9238795325112867385, 1.000000000000000000, 0.9238795325112867385, 1.000000000000000000, 0.9238795325112867385, 1.000000000000000000, 0.9238795325112867385, 1.000000000000000000, 0.9238795325112867385, 1.000000000000000000, 0.9238795325112867385, 1.000000000000000000, 0.9238795325112867385, 1.000000000000000000, 0.9238795325112867385, 1.000000000000000000, 0.9238795325112867385, 1.000000000000000000, 0.9238795325112867385, 1.000000000000000000, 0.9238795325112867385, 1.000000000000000000, 0.9238795325112867385, 1.000000000000000000, 0.9238795325112867385, 1.000000000000000000, 0.9238795325112867385, 1.000000000000000000, 0.9238795325112867385, 1.000000000000000000, 0.9238795325112867385, 1.000000000000000000, 0.9238795325112867385, 1.000000000000000000, 0.9238795325112867385, 1.000000000000000000, 0.9238795325112867385, 1.000000000000000000, 0.9238795325112867385, 1.000000000000000000, 0.9238795325112867385, 1.000000000000000000, 0.9238795325112867385, 1.000000000000000000, 0.9238795325112867385, 1.000000000000000000, 0.9238795325112867385, 1.000000000000000000, 0.9238795325112867385, 1.000000000000000000, 0.9238795325112867385, 1.000000000000000000, 0.9238795325112867385, 1.000000000000000000, 0.9238795325112867385, 1.000000000000000000, 0.9238795325112867385, 1.000000000000000000, 0.9238795325112867385, 1.000000000000000000, 0.9238795325112867385, 1.000000000000000000, 0.9238795325112867385, 1.000000000000000000, 0.9238795325112867385, 1.000000000000000000, 0.9238795325112867385, 1.000000000000000000, 0.9238795325112867385, 1.000000000000000000, 0.9238795325112867385, 1.000000000000000000, 0.9238795325112867385, 1.000000000000000000, 0.9238795325112867385, 1.000000000000000000, 0.9238795325112867385, 1.000000000000000000, 0.9238795325112867385, 1.000000000000000000, 0.9238795325112867385, 1.000000000000000000, 0.9238795325112867385, 1.000000000000000000, 0.9619397654560437605, 0.9619397662556433692 ) ) 
 REPRESENTATION_ITEM ( '' )  );
#12562=DIRECTION ( 'NONE',  ( -0.6592143633790360502, -0.5000000000000125455, 0.5616372700549346897 ) ) ;
#12578=CARTESIAN_POINT ( 'NONE',  ( -59.59170313451811296, -129.7500000013656063, 1.485763867205729394 ) ) ;
#12585=EDGE_LOOP ( 'NONE', ( #62120, #38181, #52148, #16112 ) ) ;
#12587=CARTESIAN_POINT ( 'NONE',  ( -55.39835681537999790, -154.0000000027312410, 4.984105922594378235 ) ) ;
#12619=CARTESIAN_POINT ( 'NONE',  ( -51.75738570946856498, -144.8750000027312126, 3.805975901505576964 ) ) ;
#12622=CARTESIAN_POINT ( 'NONE',  ( -55.35523342533222291, -140.5625000013656063, 4.444560631937231499 ) ) ;
#12639=EDGE_CURVE ( 'NONE', #4656, #61181, #56402, .T. ) ;
#12654=CARTESIAN_POINT ( 'NONE',  ( -52.10840900171896806, -142.4375000013656063, 3.393966926194110556 ) ) ;
#12660=EDGE_CURVE ( 'NONE', #3805, #29717, #23511, .T. ) ;
#12669=CARTESIAN_POINT ( 'NONE',  ( -58.24261429053147765, -152.2500000000000284, -3.805975901505573855 ) ) ;
#12670=CARTESIAN_POINT ( 'NONE',  ( -52.53715891517739323, -127.4375000000000426, -4.819101127000233298 ) ) ;
#12677=CARTESIAN_POINT ( 'NONE',  ( -53.51423613279429503, -147.2500000013656063, 4.591703134518082763 ) ) ;
#12701=CARTESIAN_POINT ( 'NONE',  ( -52.80376928212989185, -151.1250000013655779, -4.297418129356379346 ) ) ;
#12716=CARTESIAN_POINT ( 'NONE',  ( -52.53715891517739323, -152.4375000000000000, -4.819101127000233298 ) ) ;
#12718=CARTESIAN_POINT ( 'NONE',  ( -58.24261429053147765, -155.0000000000000284, -3.805975901505573411 ) ) ;
#12736=CARTESIAN_POINT ( 'NONE',  ( -60.14911071818854538, -139.0625000000000284, 1.666127454062681368 ) ) ;
#12747=CARTESIAN_POINT ( 'NONE',  ( -59.59170313451810586, -139.7500000013656347, 1.485763867205729394 ) ) ;
#12749=CARTESIAN_POINT ( 'NONE',  ( -51.75738570946856498, -129.8750000027312126, 3.805975901505576964 ) ) ;
#12760=CARTESIAN_POINT ( 'NONE',  ( -59.44456063193725015, -124.5625000013655921, -0.3552334253322034230 ) ) ;
#12772=CARTESIAN_POINT ( 'NONE',  ( -59.29741812935640155, -135.6250000013655779, -2.196230717870135685 ) ) ;
#12782=CARTESIAN_POINT ( 'NONE',  ( -57.89159099828107458, -128.9375000013656063, -3.393966926194107447 ) ) ;
#12807=CARTESIAN_POINT ( 'NONE',  ( -58.39396692619412477, -153.6875000013656063, 2.891590998281057701 ) ) ;
#12811=CARTESIAN_POINT ( 'NONE',  ( -59.29741812935640155, -140.6250000013656063, -2.196230717870135685 ) ) ;
#12816=CARTESIAN_POINT ( 'NONE',  ( -55.39835681537999790, -148.8750000000000284, 4.984105922594378235 ) ) ;
#12825=CARTESIAN_POINT ( 'NONE',  ( -59.29741812935640155, -152.8750000013656063, -2.196230717870135685 ) ) ;
#12826=CARTESIAN_POINT ( 'NONE',  ( -60.14911071818854538, -141.1875000027312126, 1.666127454062681368 ) ) ;
#12833=CARTESIAN_POINT ( 'NONE',  ( -56.48576386720575471, -135.7500000013656063, -4.591703134518078322 ) ) ;
#12851=CARTESIAN_POINT ( 'NONE',  ( -58.39396692619412477, -147.4375000013656063, 2.891590998281057701 ) ) ;
#12864=CARTESIAN_POINT ( 'NONE',  ( -51.75738570946856498, -151.8750000027312126, 3.805975901505576964 ) ) ;
#12891=CARTESIAN_POINT ( 'NONE',  ( -50.70258187064364108, -132.3750000013656347, 2.196230717870141014 ) ) ;
#12896=ORIENTED_EDGE ( 'NONE', *, *, #22819, .F. ) ;
#12897=CARTESIAN_POINT ( 'NONE',  ( -54.60164318462004474, -153.5000000027312410, -4.984105922594373794 ) ) ;
#12934=CARTESIAN_POINT ( 'NONE',  ( -57.19623071787017210, -135.6250000013655779, 4.297418129356382899 ) ) ;
#12937=CARTESIAN_POINT ( 'NONE',  ( -50.01589407740564042, -145.6250000000000284, 0.3983568153799778022 ) ) ;
#12965=CARTESIAN_POINT ( 'NONE',  ( -57.89159099828107458, -143.9375000013656063, -3.393966926194107447 ) ) ;
#12973=FACE_OUTER_BOUND ( 'NONE', #32744, .T. ) ;
#12984=CARTESIAN_POINT ( 'NONE',  ( -58.39396692619412477, -148.4375000013656063, 2.891590998281057701 ) ) ;
#13015=CARTESIAN_POINT ( 'NONE',  ( -58.39396692619412477, -146.6875000013656063, 2.891590998281057701 ) ) ;
#13055=CARTESIAN_POINT ( 'NONE',  ( -51.19402409849444524, -138.5000000000000284, -3.242614290531456334 ) ) ;
#13064=CARTESIAN_POINT ( 'NONE',  ( -50.55543936806279248, -139.3125000013656063, 0.3552334253322060320 ) ) ;
#13066=CARTESIAN_POINT ( 'NONE',  ( -50.18089887299979068, -131.8125000027312126, 2.462841084822635640 ) ) ;
#13079=CARTESIAN_POINT ( 'NONE',  ( -50.40829686548195099, -127.0000000013656063, -1.485763867205728284 ) ) ;
#13092=CARTESIAN_POINT ( 'NONE',  ( -52.80376928212989185, -131.8750000013656347, -4.297418129356379346 ) ) ;
#13104=CARTESIAN_POINT ( 'NONE',  ( -50.55543936806279248, -128.3125000013656063, 0.3552334253322060320 ) ) ;
#13129=VERTEX_POINT ( 'NONE', #33842 ) ;
#13131=CARTESIAN_POINT ( 'NONE',  ( -59.59170313451810586, -138.5000000013656063, 1.485763867205729394 ) ) ;
#13137=CARTESIAN_POINT ( 'NONE',  ( -52.53715891517739323, -149.4375000000000000, -4.819101127000233298 ) ) ;
#13145=CARTESIAN_POINT ( 'NONE',  ( -58.39396692619412477, -151.6875000013656063, 2.891590998281057701 ) ) ;
#13146=CARTESIAN_POINT ( 'NONE',  ( -53.33387254593733928, -140.9375000027312126, 5.149110718188519620 ) ) ;
#13147=DIRECTION ( 'NONE',  ( 0.000000000000000000, 1.000000000000000000, 0.000000000000000000 ) ) ;
#13153=CARTESIAN_POINT ( 'NONE',  ( -56.48576386720575471, -136.7500000013655779, -4.591703134518078322 ) ) ;
#13168=CARTESIAN_POINT ( 'NONE',  ( -57.19623071787017210, -144.3750000013656063, 4.297418129356382899 ) ) ;
#13211=CARTESIAN_POINT ( 'NONE',  ( -51.75738570946856498, -144.7500000000000284, 3.805975901505576964 ) ) ;
#13212=CARTESIAN_POINT ( 'NONE',  ( -53.51423613279429503, -131.5000000013656347, 4.591703134518082763 ) ) ;
#13254=CARTESIAN_POINT ( 'NONE',  ( -50.55543936806279248, -135.3125000013656063, 0.3552334253322060320 ) ) ;
#13287=CARTESIAN_POINT ( 'NONE',  ( -50.55543936806279248, -142.3125000013656063, 0.3552334253322060320 ) ) ;
#13307=CARTESIAN_POINT ( 'NONE',  ( -59.29741812935640155, -145.6250000013655779, -2.196230717870135685 ) ) ;
#13308=CARTESIAN_POINT ( 'NONE',  ( -51.75738570946856498, -155.0000000000000284, 3.805975901505577408 ) ) ;
#13326=CARTESIAN_POINT ( 'NONE',  ( -55.39835681537999790, -143.8750000000000284, 4.984105922594378235 ) ) ;
#13333=CARTESIAN_POINT ( 'NONE',  ( -59.59170313451811296, -146.7500000013655495, 1.485763867205729394 ) ) ;
#13367=ORIENTED_EDGE ( 'NONE', *, *, #33924, .F. ) ;
#13373=CARTESIAN_POINT ( 'NONE',  ( -50.18089887299979068, -138.6875000000000284, 2.462841084822635640 ) ) ;
#13381=CARTESIAN_POINT ( 'NONE',  ( -51.60603307380591787, -139.1875000013656347, -2.891590998281053704 ) ) ;
#13383=CARTESIAN_POINT ( 'NONE',  ( -53.33387254593733928, -124.9375000027312268, 5.149110718188519620 ) ) ;
#13390=CARTESIAN_POINT ( 'NONE',  ( -55.00000000000001421, -135.0000000000000284, -8.082903768654752241 ) ) ;
#13395=CARTESIAN_POINT ( 'NONE',  ( -53.51423613279429503, -126.2500000013656063, 4.591703134518082763 ) ) ;
#13409=CARTESIAN_POINT ( 'NONE',  ( -51.60603307380591787, -127.9375000013656063, -2.891590998281053704 ) ) ;
#13418=CARTESIAN_POINT ( 'NONE',  ( -59.29741812935640155, -125.8750000013656063, -2.196230717870135685 ) ) ;
#13419=CARTESIAN_POINT ( 'NONE',  ( -51.75738570946856498, -155.0000000000000284, 3.805975901505577408 ) ) ;
#13441=CARTESIAN_POINT ( 'NONE',  ( -52.80376928212989185, -154.1250000013656347, -4.297418129356379346 ) ) ;
#13443=ORIENTED_EDGE ( 'NONE', *, *, #25296, .T. ) ;
#13446=CARTESIAN_POINT ( 'NONE',  ( -52.10840900171896806, -135.1875000013656063, 3.393966926194110556 ) ) ;
#13454=CARTESIAN_POINT ( 'NONE',  ( -51.75738570946856498, -150.7500000000000284, 3.805975901505576964 ) ) ;
#13466=CARTESIAN_POINT ( 'NONE',  ( -55.35523342533222291, -151.5625000013656063, 4.444560631937231499 ) ) ;
#13467=CARTESIAN_POINT ( 'NONE',  ( -54.60164318462004474, -142.5000000027312126, -4.984105922594373794 ) ) ;
#13476=CARTESIAN_POINT ( 'NONE',  ( -55.35523342533222291, -137.3125000013656063, 4.444560631937231499 ) ) ;
#13492=CARTESIAN_POINT ( 'NONE',  ( -57.19623071787017210, -141.3750000013656063, 4.297418129356382899 ) ) ;
#13528=CARTESIAN_POINT ( 'NONE',  ( -50.55543936806279248, -154.0625000013656347, 0.3552334253322060320 ) ) ;
#13535=CARTESIAN_POINT ( 'NONE',  ( -52.80376928212989185, -133.1250000013656063, -4.297418129356379346 ) ) ;
#13578=CARTESIAN_POINT ( 'NONE',  ( -50.70258187064364108, -135.3750000013656063, 2.196230717870141014 ) ) ;
#13607=CARTESIAN_POINT ( 'NONE',  ( -54.64476657466781973, -144.0625000013656063, -4.444560631937228834 ) ) ;
#13624=CARTESIAN_POINT ( 'NONE',  ( -55.35523342533222291, -146.3125000013656063, 4.444560631937231499 ) ) ;
#13648=CARTESIAN_POINT ( 'NONE',  ( -52.10840900171896806, -146.4375000013656063, 3.393966926194110556 ) ) ;
#13654=CARTESIAN_POINT ( 'NONE',  ( -53.33387254593751692, -135.9375000027312126, 5.149110718188503633 ) ) ;
#13671=CARTESIAN_POINT ( 'NONE',  ( -54.60164318462004474, -135.3750000000000284, -4.984105922594373794 ) ) ;
#13684=CARTESIAN_POINT ( 'NONE',  ( -51.19402409849444524, -135.5000000000000284, -3.242614290531456334 ) ) ;
#13691=CARTESIAN_POINT ( 'NONE',  ( -52.80376928212989185, -139.1250000013656063, -4.297418129356378458 ) ) ;
#13693=CARTESIAN_POINT ( 'NONE',  ( -57.46284108482265651, -125.0625000027312268, 4.819101127000239515 ) ) ;
#13697=CARTESIAN_POINT ( 'NONE',  ( -60.14911071818854538, -151.1875000027312410, 1.666127454062681146 ) ) ;
#13715=CARTESIAN_POINT ( 'NONE',  ( -56.48576386720575471, -127.7500000013655921, -4.591703134518078322 ) ) ;
#13716=CARTESIAN_POINT ( 'NONE',  ( -59.29741812935640155, -145.6250000013655779, -2.196230717870135685 ) ) ;
#13741=ORIENTED_EDGE ( 'NONE', *, *, #31183, .T. ) ;
#13750=CARTESIAN_POINT ( 'NONE',  ( -53.51423613279429503, -149.5000000013655779, 4.591703134518082763 ) ) ;
#13754=CARTESIAN_POINT ( 'NONE',  ( -59.29741812935640155, -135.6250000013655779, -2.196230717870135685 ) ) ;
#13759=CARTESIAN_POINT ( 'NONE',  ( -58.24261429053147765, -145.2500000000000284, -3.805975901505573855 ) ) ;
#13768=CARTESIAN_POINT ( 'NONE',  ( -55.35523342533222291, -148.5625000013656063, 4.444560631937231499 ) ) ;
#13769=CARTESIAN_POINT ( 'NONE',  ( -59.81910112700025905, -138.3125000027312410, -2.462841084822630311 ) ) ;
#13779=CARTESIAN_POINT ( 'NONE',  ( -57.89159099828107458, -137.6875000013656063, -3.393966926194107447 ) ) ;
#13794=CARTESIAN_POINT ( 'NONE',  ( -52.10840900171896806, -141.1875000013656063, 3.393966926194110556 ) ) ;
#13810=EDGE_CURVE ( 'NONE', #62694, #15950, #21824, .T. ) ;
#13830=CARTESIAN_POINT ( 'NONE',  ( -59.59170313451810586, -153.5000000013656063, 1.485763867205729394 ) ) ;
#13836=CARTESIAN_POINT ( 'NONE',  ( -54.64476657466781973, -132.0625000013656063, -4.444560631937228834 ) ) ;
#13844=CARTESIAN_POINT ( 'NONE',  ( -59.98410592259440222, -151.2500000027312410, -0.3983568153799752487 ) ) ;
#13865=CARTESIAN_POINT ( 'NONE',  ( -52.80376928212989185, -151.8750000013655779, -4.297418129356379346 ) ) ;
#13880=CARTESIAN_POINT ( 'NONE',  ( -59.59170313451811296, -137.7500000013656063, 1.485763867205729394 ) ) ;
#13910=CARTESIAN_POINT ( 'NONE',  ( -52.10840900171896806, -141.4375000013656063, 3.393966926194110556 ) ) ;
#13918=CARTESIAN_POINT ( 'NONE',  ( -51.19402409849444524, -150.5000000000000284, -3.242614290531456334 ) ) ;
#13919=DIRECTION ( 'NONE',  ( 1.000000000000000000, 0.000000000000000000, 0.000000000000000000 ) ) ;
#13921=( BOUNDED_CURVE ( )  B_SPLINE_CURVE ( 2, ( #10544, #53659, #9593, #9904, #15380, #24391, #35004, #19877, #43994 ),
 .UNSPECIFIED., .F., .F. ) 
 B_SPLINE_CURVE_WITH_KNOTS ( ( 3, 2, 2, 2, 3 ),
 ( 0.3416666666666669516, 0.3458333333333336035, 0.3500000000000002554, 0.3541666666666669627, 0.3583333333333336146 ),
 .UNSPECIFIED. ) 
 CURVE ( )  GEOMETRIC_REPRESENTATION_ITEM ( )  RATIONAL_B_SPLINE_CURVE ( ( 0.9999999999999948930, 0.9238795325112918455, 1.000000000000000000, 0.9238795325112867385, 1.000000000000000000, 0.9238795325112867385, 1.000000000000000000, 0.9238795325112816315, 1.000000000000005107 ) ) 
 REPRESENTATION_ITEM ( '' )  );
#13928=CARTESIAN_POINT ( 'NONE',  ( -50.40829686548195099, -144.0000000013656063, -1.485763867205728284 ) ) ;
#13943=CARTESIAN_POINT ( 'NONE',  ( -51.75738570946856498, -146.7500000000000284, 3.805975901505576964 ) ) ;
#13953=CARTESIAN_POINT ( 'NONE',  ( -50.40829686548195099, -147.2500000013656063, -1.485763867205728284 ) ) ;
#13964=CARTESIAN_POINT ( 'NONE',  ( -59.98410592259440222, -141.1250000000000284, -0.3983568153799752487 ) ) ;
#13966=DIRECTION ( 'NONE',  ( 0.6485228581062915110, 0.000000000000000000, 0.7611951803011149931 ) ) ;
#13985=CARTESIAN_POINT ( 'NONE',  ( -55.00000000000002132, -155.0000000000000284, 1.734723475976807094E-15 ) ) ;
#13990=CARTESIAN_POINT ( 'NONE',  ( -51.19402409849444524, -132.5000000000000284, -3.242614290531456334 ) ) ;
#13999=ORIENTED_EDGE ( 'NONE', *, *, #46738, .T. ) ;
#14001=CARTESIAN_POINT ( 'NONE',  ( -50.18089887299979068, -127.8125000027312268, 2.462841084822635640 ) ) ;
#14002=CARTESIAN_POINT ( 'NONE',  ( -58.24261429053147765, -152.3750000027312126, -3.805975901505573855 ) ) ;
#14003=CARTESIAN_POINT ( 'NONE',  ( -51.25318514546815862, -135.0000000000000853, 2.888716472484426312 ) ) ;
#14024=CARTESIAN_POINT ( 'NONE',  ( -51.60603307380591787, -130.9375000013656063, -2.891590998281053704 ) ) ;
#14025=CARTESIAN_POINT ( 'NONE',  ( -57.89159099828107458, -145.6875000013656063, -3.393966926194107447 ) ) ;
#14039=AXIS2_PLACEMENT_3D ( 'NONE', #41990, #51344, #17865 ) ;
#14046=CARTESIAN_POINT ( 'NONE',  ( -51.75738570946856498, -142.8750000027312126, 3.805975901505576964 ) ) ;
#14058=ORIENTED_EDGE ( 'NONE', *, *, #26298, .T. ) ;
#14059=CARTESIAN_POINT ( 'NONE',  ( -50.55543936806279248, -149.3125000013656063, 0.3552334253322060320 ) ) ;
#14063=CARTESIAN_POINT ( 'NONE',  ( -58.39396692619412477, -136.4375000013655779, 2.891590998281057701 ) ) ;
#14067=CARTESIAN_POINT ( 'NONE',  ( -54.60164318462004474, -147.3750000000000284, -4.984105922594373794 ) ) ;
#14075=CARTESIAN_POINT ( 'NONE',  ( -58.39396692619412477, -149.6875000013656063, 2.891590998281057701 ) ) ;
#14076=CARTESIAN_POINT ( 'NONE',  ( -55.39835681537999790, -139.0000000027312126, 4.984105922594378235 ) ) ;
#14089=CARTESIAN_POINT ( 'NONE',  ( -59.29741812935640155, -134.6250000013656347, -2.196230717870135685 ) ) ;
#14104=CARTESIAN_POINT ( 'NONE',  ( -50.70258187064364108, -141.1250000013655779, 2.196230717870141014 ) ) ;
#14108=CARTESIAN_POINT ( 'NONE',  ( -50.01589407740564042, -144.6250000000000284, 0.3983568153799778022 ) ) ;
#14114=CARTESIAN_POINT ( 'NONE',  ( -58.80597590150559739, -149.0000000000000284, 3.242614290531460330 ) ) ;
#14135=CARTESIAN_POINT ( 'NONE',  ( -50.55543936806279248, -153.0625000013656063, 0.3552334253322060320 ) ) ;
#14143=CARTESIAN_POINT ( 'NONE',  ( -54.64476657466781973, -127.0625000013655921, -4.444560631937228834 ) ) ;
#14152=CARTESIAN_POINT ( 'NONE',  ( -59.81910112700026616, -143.1875000000000000, -2.462841084822451343 ) ) ;
#14153=ORIENTED_EDGE ( 'NONE', *, *, #56327, .T. ) ;
#14154=CARTESIAN_POINT ( 'NONE',  ( -59.98410592259440222, -152.1250000000000284, -0.3983568153799752487 ) ) ;
#14155=CARTESIAN_POINT ( 'NONE',  ( -57.46284108482265651, -150.0625000027312126, 4.819101127000239515 ) ) ;
#14174=CARTESIAN_POINT ( 'NONE',  ( -59.44456063193725015, -153.5625000013656063, -0.3552334253322034230 ) ) ;
#14190=CARTESIAN_POINT ( 'NONE',  ( -51.60603307380591787, -136.1875000013656063, -2.891590998281053704 ) ) ;
#14191=CARTESIAN_POINT ( 'NONE',  ( -55.00000000000002132, -155.0000000000000284, 1.734723475976807094E-15 ) ) ;
#14192=CARTESIAN_POINT ( 'NONE',  ( -50.18089887299977647, -145.6875000000000284, 2.462841084822486426 ) ) ;
#14198=VERTEX_POINT ( 'NONE', #56260 ) ;
#14214=AXIS2_PLACEMENT_3D ( 'NONE', #41222, #21940, #26445 ) ;
#14219=CARTESIAN_POINT ( 'NONE',  ( -56.48576386720575471, -141.0000000013656063, -4.591703134518078322 ) ) ;
#14237=EDGE_CURVE ( 'NONE', #3805, #4656, #40808, .T. ) ;
#14239=CARTESIAN_POINT ( 'NONE',  ( -58.24261429053147765, -145.3750000027312126, -3.805975901505573855 ) ) ;
#14242=CARTESIAN_POINT ( 'NONE',  ( -52.10840900171896806, -144.1875000013656063, 3.393966926194110556 ) ) ;
#14243=LINE ( 'NONE', #18752, #31587 ) ;
#14253=CARTESIAN_POINT ( 'NONE',  ( -51.19402409849444524, -142.6250000027312126, -3.242614290531456334 ) ) ;
#14263=CARTESIAN_POINT ( 'NONE',  ( -51.75738570946856498, -143.7500000000000284, 3.805975901505576964 ) ) ;
#14270=CARTESIAN_POINT ( 'NONE',  ( -53.51423613279429503, -146.5000000013656347, 4.591703134518082763 ) ) ;
#14275=CARTESIAN_POINT ( 'NONE',  ( -51.75738570946856498, -135.8750000027312410, 3.805975901505576964 ) ) ;
#14289=CARTESIAN_POINT ( 'NONE',  ( -56.66612745406283125, -145.4375000027312126, -5.149110718188525837 ) ) ;
#14300=ORIENTED_EDGE ( 'NONE', *, *, #60309, .T. ) ;
#14307=CARTESIAN_POINT ( 'NONE',  ( -53.33387254593733928, -132.8125000000000568, 5.149110718188519620 ) ) ;
#14317=CARTESIAN_POINT ( 'NONE',  ( -53.33387254593733928, -126.9375000027312126, 5.149110718188519620 ) ) ;
#14319=CARTESIAN_POINT ( 'NONE',  ( -50.52035010823932737, -134.9999999999999147, -0.6337412764124265019 ) ) ;
#14325=FACE_OUTER_BOUND ( 'NONE', #29316, .T. ) ;
#14343=CARTESIAN_POINT ( 'NONE',  ( -50.40829686548195099, -129.0000000013656063, -1.485763867205728284 ) ) ;
#14344=CARTESIAN_POINT ( 'NONE',  ( -56.48576386720575471, -148.7500000013655779, -4.591703134518078322 ) ) ;
#14354=CARTESIAN_POINT ( 'NONE',  ( -53.51423613279429503, -125.5000000013656205, 4.591703134518082763 ) ) ;
#14374=CARTESIAN_POINT ( 'NONE',  ( -58.39396692619412477, -149.6875000013656063, 2.891590998281057701 ) ) ;
#14379=CARTESIAN_POINT ( 'NONE',  ( -55.35523342533222291, -135.3125000013656063, 4.444560631937231499 ) ) ;
#14384=CARTESIAN_POINT ( 'NONE',  ( -50.01589407740564042, -144.6250000000000284, 0.3983568153799778022 ) ) ;
#14392=CARTESIAN_POINT ( 'NONE',  ( -50.40829686548195099, -149.2500000013656063, -1.485763867205728284 ) ) ;
#14394=CARTESIAN_POINT ( 'NONE',  ( -59.81910112700025905, -139.3125000027312126, -2.462841084822630311 ) ) ;
#14405=CARTESIAN_POINT ( 'NONE',  ( -59.44456063193725015, -133.5625000013656063, -0.3552334253322034230 ) ) ;
#14408=CARTESIAN_POINT ( 'NONE',  ( -50.18089887299977647, -146.8125000027311842, 2.462841084822530835 ) ) ;
#14420=CARTESIAN_POINT ( 'NONE',  ( -55.35523342533222291, -142.3125000013656063, 4.444560631937231499 ) ) ;
#14452=CARTESIAN_POINT ( 'NONE',  ( -57.19623071787016499, -154.3750000013656063, 4.297418129356382899 ) ) ;
#14459=CARTESIAN_POINT ( 'NONE',  ( -55.35523342533222291, -125.5625000013655921, 4.444560631937231499 ) ) ;
#14470=CARTESIAN_POINT ( 'NONE',  ( -56.66612745406270335, -149.4375000027311842, -5.149110718188516067 ) ) ;
#14487=DIRECTION ( 'NONE',  ( 0.8660254037844387076, 0.000000000000000000, -0.4999999999999998890 ) ) ;
#14499=CARTESIAN_POINT ( 'NONE',  ( -54.60164318462004474, -142.3750000000000284, -4.984105922594373794 ) ) ;
#14508=CARTESIAN_POINT ( 'NONE',  ( -48.00000000000002132, -135.0000000000000284, -4.041451884327376121 ) ) ;
#14532=VECTOR ( 'NONE', #8194, 1000.000000000000000 ) ;
#14534=CARTESIAN_POINT ( 'NONE',  ( -50.55543936806279248, -140.3125000013656063, 0.3552334253322060320 ) ) ;
#14552=CARTESIAN_POINT ( 'NONE',  ( -59.44456063193725015, -145.5625000013656063, -0.3552334253322034230 ) ) ;
#14574=CARTESIAN_POINT ( 'NONE',  ( -59.29741812935640155, -145.8750000013655779, -2.196230717870135685 ) ) ;
#14581=EDGE_CURVE ( 'NONE', #15950, #54748, #60896, .T. ) ;
#14594=( BOUNDED_CURVE ( )  B_SPLINE_CURVE ( 2, ( #20996, #60246, #15849, #20683, #40601, #50899, #16164, #41228, #10701 ),
 .UNSPECIFIED., .F., .F. ) 
 B_SPLINE_CURVE_WITH_KNOTS ( ( 3, 2, 2, 2, 3 ),
 ( 0.2416666666666668628, 0.2458333333333335147, 0.2500000000000002220, 0.2541666666666668739, 0.2583333333333335813 ),
 .UNSPECIFIED. ) 
 CURVE ( )  GEOMETRIC_REPRESENTATION_ITEM ( )  RATIONAL_B_SPLINE_CURVE ( ( 0.9999999999999964473, 0.9238795325112902912, 1.000000000000000000, 0.9238795325112867385, 1.000000000000000000, 0.9238795325112867385, 1.000000000000000000, 0.9238795325112826307, 1.000000000000003997 ) ) 
 REPRESENTATION_ITEM ( '' )  );
#14600=EDGE_CURVE ( 'NONE', #52848, #38301, #12420, .T. ) ;
#14620=CARTESIAN_POINT ( 'NONE',  ( -58.24261429053147765, -134.2500000000000284, -3.805975901505573855 ) ) ;
#14629=CARTESIAN_POINT ( 'NONE',  ( -59.98410592259440222, -125.2500000027311984, -0.3983568153799752487 ) ) ;
#14631=CARTESIAN_POINT ( 'NONE',  ( -51.59932184632553032, -135.0000000000000568, 3.354125322473584525 ) ) ;
#14651=CARTESIAN_POINT ( 'NONE',  ( -52.10840900171896806, -128.1875000013656063, 3.393966926194110556 ) ) ;
#14652=CARTESIAN_POINT ( 'NONE',  ( -51.60603307380591787, -146.9375000013656063, -2.891590998281053704 ) ) ;
#14676=ADVANCED_FACE ( 'NONE', ( #27448 ), #51285, .T. ) ;
#14683=ADVANCED_FACE ( 'NONE', ( #12973 ), #57373, .F. ) ;
#14688=CARTESIAN_POINT ( 'NONE',  ( -52.10840900171896806, -152.4375000013656063, 3.393966926194110556 ) ) ;
#14694=( BOUNDED_CURVE ( )  B_SPLINE_CURVE ( 2, ( #62568, #7269, #7895, #27500, #47129, #41974, #61616, #22695, #27192 ),
 .UNSPECIFIED., .F., .F. ) 
 B_SPLINE_CURVE_WITH_KNOTS ( ( 3, 2, 2, 2, 3 ),
 ( 0.05833333333333338283, 0.06250000000000005551, 0.06666666666666672125, 0.07083333333333338699, 0.07500000000000005274 ),
 .UNSPECIFIED. ) 
 CURVE ( )  GEOMETRIC_REPRESENTATION_ITEM ( )  RATIONAL_B_SPLINE_CURVE ( ( 0.9999999999999991118, 0.9238795325112876267, 1.000000000000000000, 0.9238795325112867385, 1.000000000000000000, 0.9238795325112867385, 1.000000000000000000, 0.9238795325112857393, 1.000000000000001110 ) ) 
 REPRESENTATION_ITEM ( '' )  );
#14698=CARTESIAN_POINT ( 'NONE',  ( -49.85088928181150436, -144.5625000000000284, -1.666127454062680702 ) ) ;
#14705=CARTESIAN_POINT ( 'NONE',  ( -58.39396692619412477, -147.6875000013656063, 2.891590998281057701 ) ) ;
#14706=CARTESIAN_POINT ( 'NONE',  ( -50.18089887299979068, -137.8125000027312126, 2.462841084822635640 ) ) ;
#14718=CARTESIAN_POINT ( 'NONE',  ( -59.59170313451811296, -134.5000000013656063, 1.485763867205729394 ) ) ;
#14734=CARTESIAN_POINT ( 'NONE',  ( -57.89159099828107458, -143.6875000013656063, -3.393966926194107447 ) ) ;
#14740=ORIENTED_EDGE ( 'NONE', *, *, #25191, .T. ) ;
#14765=CARTESIAN_POINT ( 'NONE',  ( -52.10840900171896806, -154.1875000013656063, 3.393966926194110556 ) ) ;
#14772=CARTESIAN_POINT ( 'NONE',  ( -50.70258187064364108, -126.3750000013656489, 2.196230717870141014 ) ) ;
#14784=CARTESIAN_POINT ( 'NONE',  ( -57.46284108482265651, -149.0625000027312126, 4.819101127000239515 ) ) ;
#14786=EDGE_CURVE ( 'NONE', #39907, #59424, #52222, .T. ) ;
#14789=( BOUNDED_CURVE ( )  B_SPLINE_CURVE ( 2, ( #3970, #23591, #62828, #33547, #38672, #53476, #25155, #39304, #20013 ),
 .UNSPECIFIED., .F., .F. ) 
 B_SPLINE_CURVE_WITH_KNOTS ( ( 3, 2, 2, 2, 3 ),
 ( 0.3583333333333336146, 0.3625000000000002665, 0.3666666666666669183, 0.3708333333333336257, 0.3750000000000002776 ),
 .UNSPECIFIED. ) 
 CURVE ( )  GEOMETRIC_REPRESENTATION_ITEM ( )  RATIONAL_B_SPLINE_CURVE ( ( 0.9999999999999948930, 0.9238795325112918455, 1.000000000000000000, 0.9238795325112867385, 1.000000000000000000, 0.9238795325112867385, 1.000000000000000000, 0.9238795325112816315, 1.000000000000005107 ) ) 
 REPRESENTATION_ITEM ( '' )  );
#14790=DIRECTION ( 'NONE',  ( 0.000000000000000000, 1.000000000000000000, 0.000000000000000000 ) ) ;
#14799=DIRECTION ( 'NONE',  ( 0.000000000000000000, 1.000000000000000000, 0.000000000000000000 ) ) ;
#14803=CARTESIAN_POINT ( 'NONE',  ( -55.35523342533222291, -153.3125000013656063, 4.444560631937231499 ) ) ;
#14826=CARTESIAN_POINT ( 'NONE',  ( -58.80597590150559739, -135.0000000000000284, 3.242614290531460330 ) ) ;
#14827=ORIENTED_EDGE ( 'NONE', *, *, #54323, .T. ) ;
#14837=CARTESIAN_POINT ( 'NONE',  ( -57.46284108482265651, -144.0625000027312126, 4.819101127000238627 ) ) ;
#14849=CARTESIAN_POINT ( 'NONE',  ( -55.35523342533222291, -137.5625000013656063, 4.444560631937231499 ) ) ;
#14856=CARTESIAN_POINT ( 'NONE',  ( -51.75738570946856498, -150.7500000000000284, 3.805975901505576964 ) ) ;
#14866=CARTESIAN_POINT ( 'NONE',  ( -56.37266686252615955, -135.0000000000000284, -4.242180533871957593 ) ) ;
#14869=CARTESIAN_POINT ( 'NONE',  ( -55.35523342533222291, -141.3125000013656063, 4.444560631937231499 ) ) ;
#14896=CARTESIAN_POINT ( 'NONE',  ( -59.29741812935640155, -143.8750000013655779, -2.196230717870135685 ) ) ;
#14936=CARTESIAN_POINT ( 'NONE',  ( -58.24261429053147765, -132.2500000000000284, -3.805975901505573855 ) ) ;
#14941=EDGE_CURVE ( 'NONE', #34224, #28303, #30437, .T. ) ;
#14948=CARTESIAN_POINT ( 'NONE',  ( -53.51423613279429503, -152.2500000013656347, 4.591703134518082763 ) ) ;
#14950=CARTESIAN_POINT ( 'NONE',  ( -50.61409141273333745, -135.0000000000000568, -1.008919204746617782 ) ) ;
#14975=CARTESIAN_POINT ( 'NONE',  ( -55.35523342533222291, -154.5625000013656347, 4.444560631937231499 ) ) ;
#14976=CARTESIAN_POINT ( 'NONE',  ( -50.70258187064364108, -146.1250000013656063, 2.196230717870141014 ) ) ;
#14999=ORIENTED_EDGE ( 'NONE', *, *, #30650, .T. ) ;
#15009=CARTESIAN_POINT ( 'NONE',  ( -55.35523342533222291, -149.5625000013656063, 4.444560631937231499 ) ) ;
#15019=CARTESIAN_POINT ( 'NONE',  ( -60.14911071818854538, -144.0625000000000284, 1.666127454062681368 ) ) ;
#15029=CARTESIAN_POINT ( 'NONE',  ( -50.40829686548195099, -148.2500000013656347, -1.485763867205728284 ) ) ;
#15031=CARTESIAN_POINT ( 'NONE',  ( -50.01589407740564042, -138.7500000027312126, 0.3983568153799778022 ) ) ;
#15045=CARTESIAN_POINT ( 'NONE',  ( -59.29741812935640155, -133.6250000013655779, -2.196230717870135685 ) ) ;
#15056=ADVANCED_FACE ( 'NONE', ( #5863 ), #35137, .F. ) ;
#15066=CARTESIAN_POINT ( 'NONE',  ( -50.40829686548195099, -137.0000000013655779, -1.485763867205728284 ) ) ;
#15077=CARTESIAN_POINT ( 'NONE',  ( -58.24261429053147765, -153.3750000027312126, -3.805975901505573855 ) ) ;
#15096=CARTESIAN_POINT ( 'NONE',  ( -57.89159099828107458, -149.6875000013656063, -3.393966926194107447 ) ) ;
#15103=CARTESIAN_POINT ( 'NONE',  ( -50.55543936806279248, -126.3125000013655921, 0.3552334253322060320 ) ) ;
#15111=CARTESIAN_POINT ( 'NONE',  ( -59.98410592259440222, -150.1250000000000284, -0.3983568153799752487 ) ) ;
#15115=CARTESIAN_POINT ( 'NONE',  ( -56.66612745406270335, -151.4375000027311842, -5.149110718188516067 ) ) ;
#15132=CARTESIAN_POINT ( 'NONE',  ( -58.39396692619412477, -152.4375000013656063, 2.891590998281057701 ) ) ;
#15134=CARTESIAN_POINT ( 'NONE',  ( -51.75738570946856498, -148.7500000000000284, 3.805975901505576964 ) ) ;
#15145=CARTESIAN_POINT ( 'NONE',  ( -58.24261429053147765, -142.2500000000000284, -3.805975901505573855 ) ) ;
#15156=CARTESIAN_POINT ( 'NONE',  ( -59.31337900967797339, -134.9999999999999716, -1.887341660144209454 ) ) ;
#15177=CARTESIAN_POINT ( 'NONE',  ( -59.59170313451811296, -138.7500000013656063, 1.485763867205729394 ) ) ;
#15191=AXIS2_PLACEMENT_3D ( 'NONE', #62961, #546, #24027 ) ;
#15197=CARTESIAN_POINT ( 'NONE',  ( -50.40829686548195099, -142.0000000013656063, -1.485763867205728284 ) ) ;
#15221=CARTESIAN_POINT ( 'NONE',  ( -59.44456063193725015, -143.8125000013656063, -0.3552334253322034230 ) ) ;
#15239=EDGE_CURVE ( 'NONE', #55226, #35208, #4994, .T. ) ;
#15243=CARTESIAN_POINT ( 'NONE',  ( -48.00000000000002132, -135.0000000000000284, -4.041451884327376121 ) ) ;
#15244=CARTESIAN_POINT ( 'NONE',  ( -49.85088928181150436, -145.6875000027311842, -1.666127454062680480 ) ) ;
#15265=CARTESIAN_POINT ( 'NONE',  ( -53.33387254593733928, -130.8125000000000568, 5.149110718188519620 ) ) ;
#15273=CARTESIAN_POINT ( 'NONE',  ( -58.80597590150559739, -124.1250000027312126, 3.242614290531460330 ) ) ;
#15286=CARTESIAN_POINT ( 'NONE',  ( -58.24261429053147765, -145.2500000000000284, -3.805975901505573855 ) ) ;
#15287=CARTESIAN_POINT ( 'NONE',  ( -51.75738570946856498, -146.7500000000000284, 3.805975901505576964 ) ) ;
#15299=CARTESIAN_POINT ( 'NONE',  ( -52.80376928212989185, -154.1250000013656347, -4.297418129356379346 ) ) ;
#15300=B_SPLINE_CURVE_WITH_KNOTS ( 'NONE', 3,
 ( #14826, #34440, #39587, #54069, #18713, #10008, #29620, #5192, #44413, #374, #19978, #59224, #15156, #57965, #54401, #33515, #53133, #10331, #29941, #9065, #28675, #40240, #30583, #49879 ),
 .UNSPECIFIED., .F., .F.,
 ( 4, 2, 2, 2, 2, 2, 2, 2, 2, 2, 2, 4 ),
 ( 0.000000000000000000, 0.001161859418553695721, 0.001742789127830540220, 0.002323718837107384503, 0.003485578255661076971, 0.004647437674214769873, 0.005809297092768463643, 0.006390226802045317032, 0.006971156511322169555, 0.007552086220599022945, 0.008133015929875876335, 0.009294875348429583115 ),
 .UNSPECIFIED. ) ;
#15301=CARTESIAN_POINT ( 'NONE',  ( -53.51423613279429503, -144.2500000013656063, 4.591703134518083651 ) ) ;
#15333=EDGE_LOOP ( 'NONE', ( #12100, #34174, #3089, #54856 ) ) ;
#15334=CARTESIAN_POINT ( 'NONE',  ( -59.44456063193725015, -145.8125000013656063, -0.3552334253322034230 ) ) ;
#15345=CARTESIAN_POINT ( 'NONE',  ( -56.66612745406270335, -141.3125000000000000, -5.149110718188516067 ) ) ;
#15353=ORIENTED_EDGE ( 'NONE', *, *, #21754, .F. ) ;
#15354=CARTESIAN_POINT ( 'NONE',  ( -52.10840900171896806, -144.4375000013656063, 3.393966926194110556 ) ) ;
#15356=CARTESIAN_POINT ( 'NONE',  ( -52.53715891517739323, -133.5625000027312410, -4.819101127000233298 ) ) ;
#15370=CARTESIAN_POINT ( 'NONE',  ( -55.35523342533222291, -130.3125000013656063, 4.444560631937231499 ) ) ;
#15376=ORIENTED_EDGE ( 'NONE', *, *, #389, .F. ) ;
#15380=CARTESIAN_POINT ( 'NONE',  ( -51.19402409849444524, -143.6250000027312126, -3.242614290531456334 ) ) ;
#15385=CARTESIAN_POINT ( 'NONE',  ( -52.80376928212989185, -135.8750000013655779, -4.297418129356379346 ) ) ;
#15392=ORIENTED_EDGE ( 'NONE', *, *, #33369, .T. ) ;
#15394=CARTESIAN_POINT ( 'NONE',  ( -59.44456063193725015, -132.8125000013656063, -0.3552334253322034230 ) ) ;
#15404=ADVANCED_FACE ( 'NONE', ( #43734 ), #9957, .F. ) ;
#15413=EDGE_CURVE ( 'NONE', #7221, #49592, #63331, .T. ) ;
#15423=CARTESIAN_POINT ( 'NONE',  ( -58.39396692619412477, -151.4375000013656063, 2.891590998281057701 ) ) ;
#15430=EDGE_CURVE ( 'NONE', #59704, #44176, #43110, .T. ) ;
#15432=CARTESIAN_POINT ( 'NONE',  ( -55.00000000000002132, -155.0000000000000284, 1.734723475976807094E-15 ) ) ;
#15434=CARTESIAN_POINT ( 'NONE',  ( -51.60603307380591787, -126.1875000013656063, -2.891590998281053704 ) ) ;
#15443=CARTESIAN_POINT ( 'NONE',  ( -59.81910112700025905, -148.3125000027312126, -2.462841084822630311 ) ) ;
#15461=CARTESIAN_POINT ( 'NONE',  ( -50.70258187064364108, -148.1250000013656063, 2.196230717870141014 ) ) ;
#15463=CARTESIAN_POINT ( 'NONE',  ( -51.19402409849444524, -148.5000000000000284, -3.242614290531456334 ) ) ;
#15497=CARTESIAN_POINT ( 'NONE',  ( -51.75738570946856498, -149.8750000027312126, 3.805975901505576964 ) ) ;
#15509=CARTESIAN_POINT ( 'NONE',  ( -59.44456063193725015, -137.8125000013656063, -0.3552334253322034230 ) ) ;
#15513=EDGE_LOOP ( 'NONE', ( #12896, #50473, #61408, #59082 ) ) ;
#15527=CARTESIAN_POINT ( 'NONE',  ( -55.35523342533222291, -142.3125000013656063, 4.444560631937231499 ) ) ;
#15553=CARTESIAN_POINT ( 'NONE',  ( -54.64476657466781973, -145.0625000013656063, -4.444560631937228834 ) ) ;
#15554=DIRECTION ( 'NONE',  ( -0.6485228581062915110, 0.000000000000000000, -0.7611951803011149931 ) ) ;
#15593=CARTESIAN_POINT ( 'NONE',  ( -54.60164318462004474, -129.3750000000000284, -4.984105922594373794 ) ) ;
#15599=CARTESIAN_POINT ( 'NONE',  ( -59.29741812935640155, -152.6250000013656063, -2.196230717870135685 ) ) ;
#15625=CARTESIAN_POINT ( 'NONE',  ( -59.29741812935640155, -126.6250000013656489, -2.196230717870135685 ) ) ;
#15626=CARTESIAN_POINT ( 'NONE',  ( -54.64476657466781973, -142.8125000013656063, -4.444560631937228834 ) ) ;
#15639=CARTESIAN_POINT ( 'NONE',  ( -51.75738570946856498, -155.0000000000000284, 3.805975901505577408 ) ) ;
#15663=CARTESIAN_POINT ( 'NONE',  ( -53.33387254593733928, -140.8125000000000284, 5.149110718188519620 ) ) ;
#15672=CARTESIAN_POINT ( 'NONE',  ( -51.60603307380591787, -148.1875000013656063, -2.891590998281053704 ) ) ;
#15674=CARTESIAN_POINT ( 'NONE',  ( -50.18089887299979068, -133.8125000027312126, 2.462841084822635640 ) ) ;
#15687=CARTESIAN_POINT ( 'NONE',  ( -56.48576386720575471, -130.7500000013656063, -4.591703134518078322 ) ) ;
#15698=EDGE_CURVE ( 'NONE', #28303, #54373, #38693, .T. ) ;
#15703=CARTESIAN_POINT ( 'NONE',  ( -57.89159099828107458, -139.6875000013656063, -3.393966926194107447 ) ) ;
#15712=CARTESIAN_POINT ( 'NONE',  ( -53.51423613279429503, -133.5000000013656347, 4.591703134518082763 ) ) ;
#15737=CARTESIAN_POINT ( 'NONE',  ( -52.10840900171896806, -151.1875000013656063, 3.393966926194110556 ) ) ;
#15744=CARTESIAN_POINT ( 'NONE',  ( -56.66612745406270335, -152.3125000000000000, -5.149110718188516067 ) ) ;
#15755=CARTESIAN_POINT ( 'NONE',  ( -51.75738570946856498, -144.8750000027312126, 3.805975901505576964 ) ) ;
#15775=CARTESIAN_POINT ( 'NONE',  ( -59.44456063193725015, -151.5625000013656063, -0.3552334253322034230 ) ) ;
#15795=CARTESIAN_POINT ( 'NONE',  ( -59.81910112700027327, -141.1875000000000000, -2.462841084822392279 ) ) ;
#15823=CARTESIAN_POINT ( 'NONE',  ( -52.10840900171896806, -134.4375000013656063, 3.393966926194110556 ) ) ;
#15833=CARTESIAN_POINT ( 'NONE',  ( -50.75781946612335105, -135.0000000000005969, -1.372666862511563224 ) ) ;
#15841=CARTESIAN_POINT ( 'NONE',  ( -52.80376928212989185, -139.8750000013655779, -4.297418129356379346 ) ) ;
#15849=CARTESIAN_POINT ( 'NONE',  ( -50.01589407740564042, -147.6250000000000284, 0.3983568153799778022 ) ) ;
#15867=CARTESIAN_POINT ( 'NONE',  ( -59.59170313451811296, -142.7500000013656063, 1.485763867205729394 ) ) ;
#15882=CARTESIAN_POINT ( 'NONE',  ( -49.85088928181150436, -138.6875000027312126, -1.666127454062680480 ) ) ;
#15907=CARTESIAN_POINT ( 'NONE',  ( -60.14911071818854538, -129.0625000000000000, 1.666127454062681368 ) ) ;
#15914=CARTESIAN_POINT ( 'NONE',  ( -52.80376928212989185, -153.8750000013655779, -4.297418129356379346 ) ) ;
#15939=CARTESIAN_POINT ( 'NONE',  ( -56.48576386720575471, -126.7500000013655921, -4.591703134518078322 ) ) ;
#15940=( BOUNDED_CURVE ( )  B_SPLINE_CURVE ( 2, ( #48265, #39558, #34412, #24148, #38313 ),
 .UNSPECIFIED., .F., .F. ) 
 B_SPLINE_CURVE_WITH_KNOTS ( ( 3, 2, 3 ),
 ( 0.000000000000000000, 0.004166666666666670078, 0.008333333333333340157 ),
 .UNSPECIFIED. ) 
 CURVE ( )  GEOMETRIC_REPRESENTATION_ITEM ( )  RATIONAL_B_SPLINE_CURVE ( ( 1.000000000000000000, 0.9238795325112867385, 1.000000000000000000, 0.9238795325112866275, 1.000000000000000222 ) ) 
 REPRESENTATION_ITEM ( '' )  );
#15941=CARTESIAN_POINT ( 'NONE',  ( -59.29741812935640155, -144.6250000013656063, -2.196230717870135685 ) ) ;
#15950=VERTEX_POINT ( 'NONE', #3193 ) ;
#15976=CARTESIAN_POINT ( 'NONE',  ( -50.01589407740564042, -139.6250000000000284, 0.3983568153799778022 ) ) ;
#15987=CARTESIAN_POINT ( 'NONE',  ( -53.51423613279429503, -143.5000000013656063, 4.591703134518083651 ) ) ;
#15989=CARTESIAN_POINT ( 'NONE',  ( -49.85088928181150436, -134.6875000027312126, -1.666127454062680702 ) ) ;
#16003=CARTESIAN_POINT ( 'NONE',  ( -50.40829686548195099, -131.0000000013656063, -1.485763867205728284 ) ) ;
#16017=CARTESIAN_POINT ( 'NONE',  ( -59.44456063193725015, -136.5625000013656063, -0.3552334253322034230 ) ) ;
#16027=CARTESIAN_POINT ( 'NONE',  ( -52.10840900171896806, -130.4375000013656063, 3.393966926194110556 ) ) ;
#16035=CARTESIAN_POINT ( 'NONE',  ( -52.53715891517739323, -151.4375000000000284, -4.819101127000233298 ) ) ;
#16052=CARTESIAN_POINT ( 'NONE',  ( -57.19623071787016499, -150.3750000013656063, 4.297418129356382899 ) ) ;
#16059=CARTESIAN_POINT ( 'NONE',  ( -52.53715891517739323, -153.4375000000000284, -4.819101127000233298 ) ) ;
#16071=CARTESIAN_POINT ( 'NONE',  ( -59.98410592259440222, -148.2500000027312126, -0.3983568153799752487 ) ) ;
#16080=CARTESIAN_POINT ( 'NONE',  ( -55.00000000000001421, -135.0000000000000284, 8.082903768654762899 ) ) ;
#16089=CARTESIAN_POINT ( 'NONE',  ( -54.60164318462004474, -143.3750000000000284, -4.984105922594373794 ) ) ;
#16091=CARTESIAN_POINT ( 'NONE',  ( -50.55543936806279248, -148.0625000013656063, 0.3552334253322060320 ) ) ;
#16108=CARTESIAN_POINT ( 'NONE',  ( -59.98410592259440222, -152.2500000027312410, -0.3983568153799752487 ) ) ;
#16112=ORIENTED_EDGE ( 'NONE', *, *, #35304, .T. ) ;
#16118=EDGE_CURVE ( 'NONE', #29717, #29222, #8660, .T. ) ;
#16122=CARTESIAN_POINT ( 'NONE',  ( -50.18089887299978358, -147.8125000027312126, 2.462841084822545934 ) ) ;
#16128=LINE ( 'NONE', #55051, #10130 ) ;
#16139=CARTESIAN_POINT ( 'NONE',  ( -59.44456063193725015, -134.8125000013656063, -0.3552334253322034230 ) ) ;
#16141=ORIENTED_EDGE ( 'NONE', *, *, #26357, .F. ) ;
#16150=ORIENTED_EDGE ( 'NONE', *, *, #32699, .T. ) ;
#16164=CARTESIAN_POINT ( 'NONE',  ( -54.60164318462004474, -147.3750000000000284, -4.984105922594373794 ) ) ;
#16171=( BOUNDED_CURVE ( )  B_SPLINE_CURVE ( 2, ( #50466, #6405, #40794, #51642, #7576, #52585, #48058, #42917, #56472 ),
 .UNSPECIFIED., .F., .F. ) 
 B_SPLINE_CURVE_WITH_KNOTS ( ( 3, 2, 2, 2, 3 ),
 ( 0.5250000000000004663, 0.5291666666666671182, 0.5333333333333338810, 0.5375000000000005329, 0.5416666666666671848 ),
 .UNSPECIFIED. ) 
 CURVE ( )  GEOMETRIC_REPRESENTATION_ITEM ( )  RATIONAL_B_SPLINE_CURVE ( ( 0.9999999999999918954, 0.9238795325112948431, 1.000000000000000000, 0.9238795325112867385, 1.000000000000000000, 0.9238795325112867385, 1.000000000000000000, 0.9238795325112766355, 1.000000000000010214 ) ) 
 REPRESENTATION_ITEM ( '' )  );
#16182=CARTESIAN_POINT ( 'NONE',  ( -55.35523342533222291, -139.5625000013656063, 4.444560631937231499 ) ) ;
#16230=CARTESIAN_POINT ( 'NONE',  ( -58.80597590150559739, -129.0000000000000284, 3.242614290531460330 ) ) ;
#16239=CARTESIAN_POINT ( 'NONE',  ( -53.51423613279429503, -154.2500000013656063, 4.591703134518082763 ) ) ;
#16246=CARTESIAN_POINT ( 'NONE',  ( -50.18089887299979068, -152.8125000027311842, 2.462841084822613436 ) ) ;
#16264=CARTESIAN_POINT ( 'NONE',  ( -59.44456063193725015, -124.5625000013655921, -0.3552334253322034230 ) ) ;
#16265=CARTESIAN_POINT ( 'NONE',  ( -50.55543936806279248, -143.0625000013656063, 0.3552334253322060320 ) ) ;
#16286=VERTEX_POINT ( 'NONE', #32364 ) ;
#16288=VERTEX_POINT ( 'NONE', #16622 ) ;
#16293=ORIENTED_EDGE ( 'NONE', *, *, #27086, .T. ) ;
#16301=CARTESIAN_POINT ( 'NONE',  ( -49.85088928181150436, -141.5625000000000568, -1.666127454062680702 ) ) ;
#16304=DIRECTION ( 'NONE',  ( 0.000000000000000000, 1.000000000000000000, 0.000000000000000000 ) ) ;
#16310=CARTESIAN_POINT ( 'NONE',  ( -59.98410592259440222, -137.2500000027312126, -0.3983568153799752487 ) ) ;
#16313=CARTESIAN_POINT ( 'NONE',  ( -59.29741812935640155, -143.8750000013655779, -2.196230717870135685 ) ) ;
#16315=CARTESIAN_POINT ( 'NONE',  ( -49.85088928181150436, -135.6875000027312126, -1.666127454062680702 ) ) ;
#16329=CARTESIAN_POINT ( 'NONE',  ( -58.39396692619412477, -127.4375000013656063, 2.891590998281057701 ) ) ;
#16332=CARTESIAN_POINT ( 'NONE',  ( -49.85088928181150436, -140.6875000027312410, -1.666127454062680480 ) ) ;
#16342=CARTESIAN_POINT ( 'NONE',  ( -59.59170313451811296, -139.5000000013656063, 1.485763867205729394 ) ) ;
#16353=CARTESIAN_POINT ( 'NONE',  ( -59.29741812935640155, -132.8750000013656063, -2.196230717870135685 ) ) ;
#16385=CARTESIAN_POINT ( 'NONE',  ( -59.81910112700025905, -153.1875000000000284, -2.462841084822630311 ) ) ;
#16393=CARTESIAN_POINT ( 'NONE',  ( -57.19623071787016499, -152.6250000013656063, 4.297418129356382899 ) ) ;
#16395=CARTESIAN_POINT ( 'NONE',  ( -55.39835681537999790, -146.0000000027312126, 4.984105922594378235 ) ) ;
#16415=CARTESIAN_POINT ( 'NONE',  ( -59.29741812935640155, -150.6250000013656063, -2.196230717870135685 ) ) ;
#16429=EDGE_CURVE ( 'NONE', #49453, #59631, #34187, .T. ) ;
#16439=PRODUCT_DEFINITION_FORMATION_WITH_SPECIFIED_SOURCE ( 'ANY', '', #19399, .NOT_KNOWN. ) ;
#16451=CARTESIAN_POINT ( 'NONE',  ( -55.39835681537999790, -141.0000000027312126, 4.984105922594378235 ) ) ;
#16458=CARTESIAN_POINT ( 'NONE',  ( -50.40829686548195099, -135.2500000013656347, -1.485763867205728284 ) ) ;
#16483=AXIS2_PLACEMENT_3D ( 'NONE', #14191, #48603, #4543 ) ;
#16500=CARTESIAN_POINT ( 'NONE',  ( -50.40829686548195099, -138.2500000013656063, -1.485763867205728284 ) ) ;
#16520=CARTESIAN_POINT ( 'NONE',  ( -58.39396692619412477, -136.6875000013656063, 2.891590998281057701 ) ) ;
#16533=CARTESIAN_POINT ( 'NONE',  ( -57.19623071787017210, -147.6250000013655779, 4.297418129356382899 ) ) ;
#16544=CARTESIAN_POINT ( 'NONE',  ( -51.75738570946856498, -127.7500000000000284, 3.805975901505576964 ) ) ;
#16552=CARTESIAN_POINT ( 'NONE',  ( -51.60603307380591787, -149.9375000013656063, -2.891590998281053704 ) ) ;
#16579=CARTESIAN_POINT ( 'NONE',  ( -55.35523342533222291, -150.5625000013656063, 4.444560631937231499 ) ) ;
#16580=CARTESIAN_POINT ( 'NONE',  ( -57.19623071787016499, -144.3750000013656063, 4.297418129356382899 ) ) ;
#16592=CARTESIAN_POINT ( 'NONE',  ( -60.14911071818854538, -136.0625000000000000, 1.666127454062681146 ) ) ;
#16593=EDGE_CURVE ( 'NONE', #39445, #4086, #8865, .T. ) ;
#16595=CARTESIAN_POINT ( 'NONE',  ( -49.85088928181150436, -152.5625000000000284, -1.666127454062680480 ) ) ;
#16616=CARTESIAN_POINT ( 'NONE',  ( -59.81910112700025905, -141.1875000000000000, -2.462841084822630311 ) ) ;
#16622=CARTESIAN_POINT ( 'NONE',  ( -58.24261429053147765, -136.3750000027312126, -3.805975901505573855 ) ) ;
#16625=CARTESIAN_POINT ( 'NONE',  ( -54.64476657466781973, -143.0625000013656063, -4.444560631937228834 ) ) ;
#16628=CARTESIAN_POINT ( 'NONE',  ( -59.98410592259440222, -134.2500000027312126, -0.3983568153799752487 ) ) ;
#16641=CARTESIAN_POINT ( 'NONE',  ( -59.44456063193725015, -130.5625000013656063, -0.3552334253322034230 ) ) ;
#16647=CARTESIAN_POINT ( 'NONE',  ( -49.85088928181150436, -139.5624999999999716, -1.666127454062680480 ) ) ;
#16654=CARTESIAN_POINT ( 'NONE',  ( -57.89159099828107458, -135.6875000013656063, -3.393966926194107447 ) ) ;
#16663=ORIENTED_EDGE ( 'NONE', *, *, #2696, .F. ) ;
#16666=CARTESIAN_POINT ( 'NONE',  ( -57.19623071787017210, -132.6250000013656347, 4.297418129356382899 ) ) ;
#16695=CARTESIAN_POINT ( 'NONE',  ( -56.48576386720575471, -140.7500000013655779, -4.591703134518078322 ) ) ;
#16701=CARTESIAN_POINT ( 'NONE',  ( -58.24261429053147765, -153.2500000000000284, -3.805975901505573855 ) ) ;
#16706=SURFACE_STYLE_FILL_AREA ( #7381 ) ;
#16712=CARTESIAN_POINT ( 'NONE',  ( -51.75738570946856498, -145.8750000027312126, 3.805975901505576964 ) ) ;
#16730=CARTESIAN_POINT ( 'NONE',  ( -60.14911071818854538, -138.0625000000000000, 1.666127454062681146 ) ) ;
#16731=CARTESIAN_POINT ( 'NONE',  ( -54.64476657466781973, -146.8125000013656063, -4.444560631937228834 ) ) ;
#16733=CARTESIAN_POINT ( 'NONE',  ( -58.24261429053147765, -148.2500000000000284, -3.805975901505573855 ) ) ;
#16774=CARTESIAN_POINT ( 'NONE',  ( -58.39396692619412477, -135.6875000013656063, 2.891590998281057701 ) ) ;
#16796=ORIENTED_EDGE ( 'NONE', *, *, #45704, .F. ) ;
#16814=CARTESIAN_POINT ( 'NONE',  ( -59.44456063193725015, -141.8125000013656063, -0.3552334253322034230 ) ) ;
#16834=CARTESIAN_POINT ( 'NONE',  ( -55.35523342533222291, -136.5625000013656063, 4.444560631937231499 ) ) ;
#16846=CARTESIAN_POINT ( 'NONE',  ( -59.59170313451811296, -147.7500000013655779, 1.485763867205729394 ) ) ;
#16853=CARTESIAN_POINT ( 'NONE',  ( -59.98410592259440222, -149.2500000027312126, -0.3983568153799752487 ) ) ;
#16862=EDGE_CURVE ( 'NONE', #54373, #40878, #27256, .T. ) ;
#16868=CARTESIAN_POINT ( 'NONE',  ( -59.44456063193725015, -147.5625000013656063, -0.3552334253322034230 ) ) ;
#16892=CARTESIAN_POINT ( 'NONE',  ( -57.19623071787017210, -151.6250000013656063, 4.297418129356382899 ) ) ;
#16907=CARTESIAN_POINT ( 'NONE',  ( -51.75738570946856498, -152.7500000000000284, 3.805975901505576964 ) ) ;
#16934=CARTESIAN_POINT ( 'NONE',  ( -59.98410592259440222, -139.1250000000000284, -0.3983568153799752487 ) ) ;
#16945=CARTESIAN_POINT ( 'NONE',  ( -58.39396692619412477, -142.6875000013656063, 2.891590998281057701 ) ) ;
#16947=CARTESIAN_POINT ( 'NONE',  ( -53.33387254593733928, -130.9375000027312126, 5.149110718188519620 ) ) ;
#16963=CARTESIAN_POINT ( 'NONE',  ( -53.33387254593716875, -141.9375000027312126, 5.149110718188532942 ) ) ;
#16967=CARTESIAN_POINT ( 'NONE',  ( -56.66612745406293783, -139.3125000000000284, -5.149110718188535607 ) ) ;
#16974=CARTESIAN_POINT ( 'NONE',  ( -50.55543936806279248, -134.0625000013656063, 0.3552334253322060320 ) ) ;
#16983=( BOUNDED_CURVE ( )  B_SPLINE_CURVE ( 2, ( #6597, #32540, #17755, #52167, #51851, #7793, #27396, #45510, #37371 ),
 .UNSPECIFIED., .F., .F. ) 
 B_SPLINE_CURVE_WITH_KNOTS ( ( 3, 2, 2, 2, 3 ),
 ( 0.5416666666666671848, 0.5458333333333338366, 0.5500000000000004885, 0.5541666666666671404, 0.5583333333333337922 ),
 .UNSPECIFIED. ) 
 CURVE ( )  GEOMETRIC_REPRESENTATION_ITEM ( )  RATIONAL_B_SPLINE_CURVE ( ( 0.9999999999999898970, 0.9238795325112968415, 1.000000000000000000, 0.9238795325112867385, 1.000000000000000000, 0.9238795325112867385, 1.000000000000000000, 0.9238795325112786339, 1.000000000000008216 ) ) 
 REPRESENTATION_ITEM ( '' )  );
#16984=CARTESIAN_POINT ( 'NONE',  ( -59.29741812935640155, -126.8750000013656205, -2.196230717870135685 ) ) ;
#17006=CARTESIAN_POINT ( 'NONE',  ( -59.29741812935640155, -153.8750000013655779, -2.196230717870135685 ) ) ;
#17010=CARTESIAN_POINT ( 'NONE',  ( -57.19623071787016499, -139.3750000013656063, 4.297418129356382899 ) ) ;
#17016=CARTESIAN_POINT ( 'NONE',  ( -59.98410592259440222, -152.1250000000000284, -0.3983568153799752487 ) ) ;
#17028=CARTESIAN_POINT ( 'NONE',  ( -56.66612745406270335, -141.4375000027312410, -5.149110718188516067 ) ) ;
#17036=CARTESIAN_POINT ( 'NONE',  ( -56.48576386720575471, -141.7500000013656063, -4.591703134518078322 ) ) ;
#17043=CARTESIAN_POINT ( 'NONE',  ( -58.24261429053147765, -150.3750000027312126, -3.805975901505573855 ) ) ;
#17048=DIRECTION ( 'NONE',  ( -0.6485228581062915110, 0.000000000000000000, -0.7611951803011149931 ) ) ;
#17050=CARTESIAN_POINT ( 'NONE',  ( -58.39396692619412477, -145.4375000013656063, 2.891590998281057701 ) ) ;
#17063=( BOUNDED_SURFACE ( )  B_SPLINE_SURFACE ( 1, 2, ( 
 ( #22155, #17943, #52680, #17643, #41749, #47230, #3173, #42386, #62026, #13441, #61398, #33066, #41435, #17006, #2856, #36621, #12807, #42073, #32428, #56254, #31793, #51425, #7368, #46595, #33998, #47839, #28853, #43328, #39131, #53305, #23419, #19196, #58758, #48781, #34306, #63279, #14688, #62969, #23733, #8927, #44273, #53929, #33684, #9239, #43637, #9552, #38809, #33372, #8615, #19517, #29157, #43022, #39446, #4723, #24349, #19833, #63597, #4113, #29468, #9858, #48475, #58451, #18582, #43949, #49101, #3798, #18885, #38500, #58128, #5047, #38205, #62662, #53621, #57830, #28223, #24665, #4411, #24035, #235, #34623, #14374, #59083, #15009, #13750, #52986, #28540, #14059, #48160, #2697, #12344, #46118, #6566, #31312, #31955, #6889, #61560, #2387, #21363, #51587, #1760, #7525, #49423, #31643, #27136, #26181, #26504, #2081, #40966, #21997, #60614, #39757, #16846, #29790, #16533, #10190, #55464, #36789, #46751, #45800, #24985, #56093, #50628, #50948, #60926, #31001, #22316, #5367, #44592, #34957, #36156, #56421, #21687, #552, #41918, #17494, #54248, #41591, #20161, #59402, #55777, #36466, #61242, #15334, #11380, #11693, #41277, #51277, #12013, #7210, #26822, #46441, #17164, #3960, #37420, #42550, #33224, #23580, #23886, #42238, #28077, #32270, #28387, #43176, #37116, #3338, #62189, #51898, #47694, #57985, #4268, #13607, #42865, #12965, #48318, #52843, #32590, #48006, #63133, #3646, #52215, #7839, #22954, #18110, #8777, #62818, #9090, #57054, #56734, #47075, #57681, #8160, #22639, #37732, #27759, #57366, #27441, #12654, #23258, #13287, #3023, #52535, #61880, #28698, #17796, #47387, #62511, #32912, #18427, #8469, #38049, #18734, #38359, #13910, #33538, #53153, #43488, #399, #9708, #4570, #14219, #5213, #45087, #58613, #20001, #25145, #54746, #10031, #29644, #49277, #48944, #14534, #29312, #49588, #5530, #24832, #4892, #44438, #24516, #19365, #34803, #44117, #38661, #717, #39930, #48631, #81, #34462, #44756, #43800, #24193, #39609, #53465, #54092, #34153, #58300, #15177, #20328, #59247, #54425, #33846, #59576, #9395, #10354, #19681, #29005, #29963, #63447, #10666, #38976, #53775, #15509, #39293, #35130, #58920, #14849, #30282, #49902, #5856, #25464, #19044, #26423, #46040, #55385, #50230, #59902, #50872, #27060, #40574, #2005, #7131, #36716, #55707, #11620, #31240, #30927, #60215, #11302, #31566, #51199, #6816, #50553, #21608, #6497, #1372, #16774, #26109, #20658, #46363, #21920, #30606, #45729, #16458, #26747, #25794, #6178, #41203, #35436, #36077, #16139, #40262, #60847, #2317, #36391, #56022, #15823, #41518, #61170, #51515, #1052, #17093, #55062, #56347, #35761, #11937, #12269, #10986, #45405, #1680, #31881, #7452, #20973, #21282, #40889, #60535, #62745, #13535, #47000, #52142, #42790, #33155, #33456, #51821, #37653, #41841, #37977, #52769, #46678, #12891, #8084, #61488, #57296, #3882, #13836, #23180, #52463, #22565, #57915, #62434, #42163, #57608, #9014, #13212, #61799, #17420, #32510, #27688, #18352, #8698, #18666, #2948, #2624, #56660, #3571, #17725, #32191, #47314, #37341, #3266, #37034, #28310, #47927, #23501, #53073, #8399, #22241, #22878, #56974, #43104, #42471, #12578, #32834, #38288, #7763, #27366, #27999, #62113, #18031, #47618, #28934, #641, #54349, #53704, #29244, #3, #29566, #19606, #53390, #28625, #39533, #49197, #63057, #59495, #5137, #24753, #39852, #19919, #24125, #49513, #34720, #9636, #39218, #38584, #44358, #321, #23811, #19286, #43726, #63370, #59171, #58215, #18969, #9949, #14143, #48242, #5452, #48869, #4815, #20250, #54664, #24436, #44039, #58843, #25070, #14772, #15103, #38901, #15434, #35052, #44680, #34391, #58537, #54017, #4198, #10279, #43414, #29884, #14459, #33770, #34081, #9321, #48558, #4497, #51117, #25719, #26035, #1607, #20895, #41129, #60138, #59823, #36004 ),
 ( #30199, #49828, #54982, #45329, #11860, #45649, #977, #55635, #11550, #31167, #50799, #60776, #1299, #2244, #45963, #6735, #40497, #26344, #21205, #11230, #50149, #40811, #1927, #45011, #60459, #16059, #5772, #21532, #16701, #16385, #36319, #25390, #31476, #7054, #61093, #36632, #55945, #20580, #26667, #6104, #46287, #21848, #40187, #15744, #35688, #41444, #17016, #10587, #55316, #35359, #50484, #10911, #30526, #30855, #6423, #52383, #23106, #43031, #61409, #47240, #51436, #47542, #62352, #56264, #22487, #61725, #7377, #3184, #13454, #23429, #32756, #62036, #32114, #3806, #8321, #51750, #3492, #18592, #22802, #7692, #26985, #42082, #37269, #27920, #42710, #28233, #12502, #12188, #2549, #13137, #27298, #41759, #56896, #46923, #17653, #46604, #31802, #42395, #12816, #22164, #8005, #17332, #47848, #36954, #2868, #17953, #32437, #37577, #56582, #52066, #27608, #57217, #18275, #37901, #57531, #33076, #52688, #8624, #62671, #33381, #24359, #562, #14067, #39142, #44284, #10200, #29168, #48792, #4734, #4421, #33695, #28863, #5057, #24676, #43960, #48485, #63607, #24046, #38509, #53939, #43648, #57840, #19843, #59093, #4122, #63288, #53631, #246, #62980, #23744, #58137, #43337, #38820, #53314, #19206, #8936, #13759, #19527, #58461, #52996, #9562, #28550, #29801, #48169, #9248, #58768, #14384, #14698, #18895, #34008, #34315, #9869, #29479, #49112, #39458, #15019, #34634, #54260, #49434, #5377, #24994, #38217, #44602, #21124, #26258, #55863, #11149, #30771, #50392, #50071, #59737, #10830, #50709, #6652, #25948, #30444, #45563, #6027, #20495, #35924, #25631, #39767, #1844, #41049, #49751, #45245, #35603, #45881, #44932, #5696, #1521, #54585, #55227, #35280, #59414, #16301, #21449, #6341, #60378, #15345, #60696, #16616, #6975, #46204, #36235, #10506, #11776, #15663, #40731, #31394, #34969, #30121, #54902, #51033, #55553, #11465, #1213, #25311, #60052, #26586, #20171, #40094, #20810, #31086, #888, #40413, #15976, #56819, #61008, #57138, #8239, #2165, #32036, #7613, #16934, #12736, #23032, #32994, #42318, #7923, #41676, #13373, #61958, #61327, #13055, #28158, #32359, #17249, #36548, #51672, #46835, #17880, #32672, #37820, #22079, #21771, #12101, #22721, #61643, #31725, #27528, #51981, #47158, #3104, #37500, #56502, #51357, #56180, #52304, #41364, #36872, #27841, #47463, #57449, #3415, #42635, #62277, #27218, #12425, #2783, #18199, #52611, #8546, #22404, #7297, #42002, #2469, #26908, #17575, #46527, #37194, #4975, #13684, #33619, #63211, #9788, #8859, #33303, #29084, #18514, #19124, #62897, #23351, #43879, #53858, #58380, #24275, #3729, #49031, #24598, #34545, #10118, #14620, #38136, #44204, #43257, #48714, #34232, #62594, #57761, #23661, #169, #63527, #38742, #18811, #52921, #23963, #19768, #29396, #48089, #53238, #19448, #39377, #54179, #28475, #14307, #42951, #39063, #59008, #47774, #13990, #9172, #4044, #33929, #14936, #38433, #58692, #53552, #58060, #28786, #48402, #4344, #43566, #9476, #4653, #44846, #24919, #59661, #10759, #45490, #60301, #1772, #49677, #29724, #39692, #50317, #5622, #15265, #30371, #25235, #54828, #485, #49356, #20738, #49992, #44525, #45171, #20087, #21373, #59332, #809, #59984, #35210, #11075, #5301, #20416, #40016, #40982, #1453, #25874, #15593, #21054, #40341, #5945, #25551, #15907, #16230, #11390, #40661, #36167, #55151, #34889, #1138, #35527, #35850, #30698, #54512, #6267, #55475, #31010, #50639, #6577, #26192, #45811, #60624, #30048, #16544, #55788, #10435, #12355, #46764, #12670, #2709, #36480, #11706, #22651, #32282, #46130, #42561, #51910, #7850, #22964, #3033, #7224, #32600, #17807, #36801, #22329, #21699, #27453, #47086, #6901, #2398, #26839, #46453, #42250, #41290, #2097, #56746, #60939, #31325, #52225, #31968, #56433, #3347, #37745, #51604, #7536, #41930, #8170, #61572 ) ),
 .UNSPECIFIED., .F., .F., .F. ) 
 B_SPLINE_SURFACE_WITH_KNOTS ( ( 2, 2 ),
 ( 3, 2, 2, 2, 2, 2, 2, 2, 2, 2, 2, 2, 2, 2, 2, 2, 2, 2, 2, 2, 2, 2, 2, 2, 2, 2, 2, 2, 2, 2, 2, 2, 2, 2, 2, 2, 2, 2, 2, 2, 2, 2, 2, 2, 2, 2, 2, 2, 2, 2, 2, 2, 2, 2, 2, 2, 2, 2, 2, 2, 2, 2, 2, 2, 2, 2, 2, 2, 2, 2, 2, 2, 2, 2, 2, 2, 2, 2, 2, 2, 2, 2, 2, 2, 2, 2, 2, 2, 2, 2, 2, 2, 2, 2, 2, 2, 2, 2, 2, 2, 2, 2, 2, 2, 2, 2, 2, 2, 2, 2, 2, 2, 2, 2, 2, 2, 2, 2, 2, 2, 2, 2, 2, 2, 2, 2, 2, 2, 2, 2, 2, 2, 2, 2, 2, 2, 2, 2, 2, 2, 2, 2, 2, 2, 2, 2, 2, 2, 2, 2, 2, 2, 2, 2, 2, 2, 2, 2, 2, 2, 2, 2, 2, 2, 2, 2, 2, 2, 2, 2, 2, 2, 2, 2, 2, 2, 2, 2, 2, 2, 2, 2, 2, 2, 2, 2, 2, 2, 2, 2, 2, 2, 2, 2, 2, 2, 2, 2, 2, 2, 2, 2, 2, 2, 2, 2, 2, 2, 2, 2, 2, 2, 2, 2, 2, 2, 2, 2, 2, 2, 2, 2, 2, 2, 2, 2, 2, 2, 2, 2, 2, 2, 2, 2, 2, 2, 2, 2, 2, 2, 3 ),
 ( 0.000000000000000000, 1.000000000000000000 ),
 ( 0.000000000000000000, 0.004166666666666666609, 0.008333333333333333218, 0.01250000000000000069, 0.01666666666666666644, 0.02083333333333333218, 0.02500000000000000139, 0.02916666666666666713, 0.03333333333333333287, 0.03749999999999999861, 0.04166666666666666435, 0.04583333333333333010, 0.05000000000000000278, 0.05416666666666666852, 0.05833333333333333426, 0.06250000000000000000, 0.06666666666666666574, 0.07083333333333333148, 0.07499999999999999722, 0.07916666666666666297, 0.08333333333333332871, 0.08749999999999999445, 0.09166666666666666019, 0.09583333333333333981, 0.1000000000000000056, 0.1041666666666666713, 0.1083333333333333370, 0.1125000000000000028, 0.1166666666666666685, 0.1208333333333333343, 0.1250000000000000000, 0.1291666666666666796, 0.1333333333333333315, 0.1375000000000000111, 0.1416666666666666630, 0.1458333333333333426, 0.1499999999999999944, 0.1541666666666666741, 0.1583333333333333259, 0.1625000000000000056, 0.1666666666666666574, 0.1708333333333333370, 0.1749999999999999889, 0.1791666666666666685, 0.1833333333333333204, 0.1875000000000000000, 0.1916666666666666796, 0.1958333333333333315, 0.2000000000000000111, 0.2041666666666666630, 0.2083333333333333426, 0.2124999999999999944, 0.2166666666666666741, 0.2208333333333333259, 0.2250000000000000056, 0.2291666666666666574, 0.2333333333333333370, 0.2374999999999999889, 0.2416666666666666685, 0.2458333333333333204, 0.2500000000000000000, 0.2541666666666666519, 0.2583333333333333592, 0.2625000000000000111, 0.2666666666666666630, 0.2708333333333333148, 0.2750000000000000222, 0.2791666666666666741, 0.2833333333333333259, 0.2874999999999999778, 0.2916666666666666852, 0.2958333333333333370, 0.2999999999999999889, 0.3041666666666666408, 0.3083333333333333481, 0.3125000000000000000, 0.3166666666666666519, 0.3208333333333333592, 0.3250000000000000111, 0.3291666666666666630, 0.3333333333333333148, 0.3375000000000000222, 0.3416666666666666741, 0.3458333333333333259, 0.3499999999999999778, 0.3541666666666666852, 0.3583333333333333370, 0.3624999999999999889, 0.3666666666666666408, 0.3708333333333333481, 0.3750000000000000000, 0.3791666666666666519, 0.3833333333333333592, 0.3875000000000000111, 0.3916666666666666630, 0.3958333333333333148, 0.4000000000000000222, 0.4041666666666666741, 0.4083333333333333259, 0.4124999999999999778, 0.4166666666666666852, 0.4208333333333333370, 0.4249999999999999889, 0.4291666666666666408, 0.4333333333333333481, 0.4375000000000000000, 0.4416666666666666519, 0.4458333333333333592, 0.4500000000000000111, 0.4541666666666666630, 0.4583333333333333148, 0.4625000000000000222, 0.4666666666666666741, 0.4708333333333333259, 0.4749999999999999778, 0.4791666666666666852, 0.4833333333333333370, 0.4874999999999999889, 0.4916666666666666408, 0.4958333333333333481, 0.5000000000000000000, 0.5041666666666666519, 0.5083333333333333037, 0.5124999999999999556, 0.5166666666666667185, 0.5208333333333333703, 0.5250000000000000222, 0.5291666666666666741, 0.5333333333333333259, 0.5374999999999999778, 0.5416666666666666297, 0.5458333333333332815, 0.5500000000000000444, 0.5541666666666666963, 0.5583333333333333481, 0.5625000000000000000, 0.5666666666666666519, 0.5708333333333333037, 0.5749999999999999556, 0.5791666666666667185, 0.5833333333333333703, 0.5875000000000000222, 0.5916666666666666741, 0.5958333333333333259, 0.5999999999999999778, 0.6041666666666666297, 0.6083333333333332815, 0.6125000000000000444, 0.6166666666666666963, 0.6208333333333333481, 0.6250000000000000000, 0.6291666666666666519, 0.6333333333333333037, 0.6374999999999999556, 0.6416666666666667185, 0.6458333333333333703, 0.6500000000000000222, 0.6541666666666666741, 0.6583333333333333259, 0.6624999999999999778, 0.6666666666666666297, 0.6708333333333332815, 0.6750000000000000444, 0.6791666666666666963, 0.6833333333333333481, 0.6875000000000000000, 0.6916666666666666519, 0.6958333333333333037, 0.6999999999999999556, 0.7041666666666667185, 0.7083333333333333703, 0.7125000000000000222, 0.7166666666666666741, 0.7208333333333333259, 0.7249999999999999778, 0.7291666666666666297, 0.7333333333333332815, 0.7375000000000000444, 0.7416666666666666963, 0.7458333333333333481, 0.7500000000000000000, 0.7541666666666666519, 0.7583333333333333037, 0.7624999999999999556, 0.7666666666666667185, 0.7708333333333333703, 0.7750000000000000222, 0.7791666666666666741, 0.7833333333333333259, 0.7874999999999999778, 0.7916666666666666297, 0.7958333333333332815, 0.8000000000000000444, 0.8041666666666666963, 0.8083333333333333481, 0.8125000000000000000, 0.8166666666666666519, 0.8208333333333333037, 0.8249999999999999556, 0.8291666666666667185, 0.8333333333333333703, 0.8375000000000000222, 0.8416666666666666741, 0.8458333333333333259, 0.8499999999999999778, 0.8541666666666666297, 0.8583333333333332815, 0.8625000000000000444, 0.8666666666666666963, 0.8708333333333333481, 0.8750000000000000000, 0.8791666666666666519, 0.8833333333333333037, 0.8874999999999999556, 0.8916666666666667185, 0.8958333333333333703, 0.9000000000000000222, 0.9041666666666666741, 0.9083333333333333259, 0.9124999999999999778, 0.9166666666666666297, 0.9208333333333332815, 0.9250000000000000444, 0.9291666666666666963, 0.9333333333333333481, 0.9375000000000000000, 0.9416666666666666519, 0.9458333333333333037, 0.9499999999999999556, 0.9541666666666667185, 0.9583333333333333703, 0.9625000000000000222, 0.9666666666666666741, 0.9708333333333333259, 0.9749999999999999778, 0.9791666666666666297, 0.9833333333333332815, 0.9875000000000000444, 0.9916666666666666963, 0.9958333333333333481, 1.000000000000000000 ),
 .UNSPECIFIED. ) 
 GEOMETRIC_REPRESENTATION_ITEM ( )  RATIONAL_B_SPLINE_SURFACE ( (
 ( 1.000000000000000000, 0.9238795325112867385, 1.000000000000000000, 0.9238795325112867385, 1.000000000000000000, 0.9238795325112867385, 1.000000000000000000, 0.9238795325112867385, 1.000000000000000000, 0.9238795325112867385, 1.000000000000000000, 0.9238795325112867385, 1.000000000000000000, 0.9238795325112867385, 1.000000000000000000, 0.9238795325112867385, 1.000000000000000000, 0.9238795325112867385, 1.000000000000000000, 0.9238795325112867385, 1.000000000000000000, 0.9238795325112867385, 1.000000000000000000, 0.9238795325112867385, 1.000000000000000000, 0.9238795325112867385, 1.000000000000000000, 0.9238795325112867385, 1.000000000000000000, 0.9238795325112867385, 1.000000000000000000, 0.9238795325112867385, 1.000000000000000000, 0.9238795325112867385, 1.000000000000000000, 0.9238795325112867385, 1.000000000000000000, 0.9238795325112867385, 1.000000000000000000, 0.9238795325112867385, 1.000000000000000000, 0.9238795325112867385, 1.000000000000000000, 0.9238795325112867385, 1.000000000000000000, 0.9238795325112867385, 1.000000000000000000, 0.9238795325112867385, 1.000000000000000000, 0.9238795325112867385, 1.000000000000000000, 0.9238795325112867385, 1.000000000000000000, 0.9238795325112867385, 1.000000000000000000, 0.9238795325112867385, 1.000000000000000000, 0.9238795325112867385, 1.000000000000000000, 0.9238795325112867385, 1.000000000000000000, 0.9238795325112867385, 1.000000000000000000, 0.9238795325112867385, 1.000000000000000000, 0.9238795325112867385, 1.000000000000000000, 0.9238795325112867385, 1.000000000000000000, 0.9238795325112867385, 1.000000000000000000, 0.9238795325112867385, 1.000000000000000000, 0.9238795325112867385, 1.000000000000000000, 0.9238795325112867385, 1.000000000000000000, 0.9238795325112867385, 1.000000000000000000, 0.9238795325112867385, 1.000000000000000000, 0.9238795325112867385, 1.000000000000000000, 0.9238795325112867385, 1.000000000000000000, 0.9238795325112867385, 1.000000000000000000, 0.9238795325112867385, 1.000000000000000000, 0.9238795325112867385, 1.000000000000000000, 0.9238795325112867385, 1.000000000000000000, 0.9238795325112867385, 1.000000000000000000, 0.9238795325112867385, 1.000000000000000000, 0.9238795325112867385, 1.000000000000000000, 0.9238795325112867385, 1.000000000000000000, 0.9238795325112867385, 1.000000000000000000, 0.9238795325112867385, 1.000000000000000000, 0.9238795325112867385, 1.000000000000000000, 0.9238795325112867385, 1.000000000000000000, 0.9238795325112867385, 1.000000000000000000, 0.9238795325112867385, 1.000000000000000000, 0.9238795325112867385, 1.000000000000000000, 0.9238795325112867385, 1.000000000000000000, 0.9238795325112867385, 1.000000000000000000, 0.9238795325112867385, 1.000000000000000000, 0.9238795325112867385, 1.000000000000000000, 0.9238795325112867385, 1.000000000000000000, 0.9238795325112867385, 1.000000000000000000, 0.9238795325112867385, 1.000000000000000000, 0.9238795325112867385, 1.000000000000000000, 0.9238795325112867385, 1.000000000000000000, 0.9238795325112867385, 1.000000000000000000, 0.9238795325112867385, 1.000000000000000000, 0.9238795325112867385, 1.000000000000000000, 0.9238795325112867385, 1.000000000000000000, 0.9238795325112867385, 1.000000000000000000, 0.9238795325112867385, 1.000000000000000000, 0.9238795325112867385, 1.000000000000000000, 0.9238795325112867385, 1.000000000000000000, 0.9238795325112867385, 1.000000000000000000, 0.9238795325112867385, 1.000000000000000000, 0.9238795325112867385, 1.000000000000000000, 0.9238795325112867385, 1.000000000000000000, 0.9238795325112867385, 1.000000000000000000, 0.9238795325112867385, 1.000000000000000000, 0.9238795325112867385, 1.000000000000000000, 0.9238795325112867385, 1.000000000000000000, 0.9238795325112867385, 1.000000000000000000, 0.9238795325112867385, 1.000000000000000000, 0.9238795325112867385, 1.000000000000000000, 0.9238795325112867385, 1.000000000000000000, 0.9238795325112867385, 1.000000000000000000, 0.9238795325112867385, 1.000000000000000000, 0.9238795325112867385, 1.000000000000000000, 0.9238795325112867385, 1.000000000000000000, 0.9238795325112867385, 1.000000000000000000, 0.9238795325112867385, 1.000000000000000000, 0.9238795325112867385, 1.000000000000000000, 0.9238795325112867385, 1.000000000000000000, 0.9238795325112867385, 1.000000000000000000, 0.9238795325112867385, 1.000000000000000000, 0.9238795325112867385, 1.000000000000000000, 0.9238795325112867385, 1.000000000000000000, 0.9238795325112867385, 1.000000000000000000, 0.9238795325112867385, 1.000000000000000000, 0.9238795325112867385, 1.000000000000000000, 0.9238795325112867385, 1.000000000000000000, 0.9238795325112867385, 1.000000000000000000, 0.9238795325112867385, 1.000000000000000000, 0.9238795325112867385, 1.000000000000000000, 0.9238795325112867385, 1.000000000000000000, 0.9238795325112867385, 1.000000000000000000, 0.9238795325112867385, 1.000000000000000000, 0.9238795325112867385, 1.000000000000000000, 0.9238795325112867385, 1.000000000000000000, 0.9238795325112867385, 1.000000000000000000, 0.9238795325112867385, 1.000000000000000000, 0.9238795325112867385, 1.000000000000000000, 0.9238795325112867385, 1.000000000000000000, 0.9238795325112867385, 1.000000000000000000, 0.9238795325112867385, 1.000000000000000000, 0.9238795325112867385, 1.000000000000000000, 0.9238795325112867385, 1.000000000000000000, 0.9238795325112867385, 1.000000000000000000, 0.9238795325112867385, 1.000000000000000000, 0.9238795325112867385, 1.000000000000000000, 0.9238795325112867385, 1.000000000000000000, 0.9238795325112867385, 1.000000000000000000, 0.9238795325112867385, 1.000000000000000000, 0.9238795325112867385, 1.000000000000000000, 0.9238795325112867385, 1.000000000000000000, 0.9238795325112867385, 1.000000000000000000, 0.9238795325112867385, 1.000000000000000000, 0.9238795325112867385, 1.000000000000000000, 0.9238795325112867385, 1.000000000000000000, 0.9238795325112867385, 1.000000000000000000, 0.9238795325112867385, 1.000000000000000000, 0.9238795325112867385, 1.000000000000000000, 0.9238795325112867385, 1.000000000000000000, 0.9238795325112867385, 1.000000000000000000, 0.9238795325112867385, 1.000000000000000000, 0.9238795325112867385, 1.000000000000000000, 0.9238795325112867385, 1.000000000000000000, 0.9238795325112867385, 1.000000000000000000, 0.9238795325112867385, 1.000000000000000000, 0.9238795325112867385, 1.000000000000000000, 0.9238795325112867385, 1.000000000000000000, 0.9238795325112867385, 1.000000000000000000, 0.9238795325112867385, 1.000000000000000000, 0.9238795325112867385, 1.000000000000000000, 0.9238795325112867385, 1.000000000000000000, 0.9238795325112867385, 1.000000000000000000, 0.9238795325112867385, 1.000000000000000000, 0.9238795325112867385, 1.000000000000000000, 0.9238795325112867385, 1.000000000000000000, 0.9238795325112867385, 1.000000000000000000, 0.9238795325112867385, 1.000000000000000000, 0.9238795325112867385, 1.000000000000000000, 0.9238795325112867385, 1.000000000000000000, 0.9238795325112867385, 1.000000000000000000, 0.9238795325112867385, 1.000000000000000000, 0.9238795325112867385, 1.000000000000000000, 0.9238795325112867385, 1.000000000000000000, 0.9238795325112867385, 1.000000000000000000, 0.9238795325112867385, 1.000000000000000000, 0.9238795325112867385, 1.000000000000000000, 0.9238795325112867385, 1.000000000000000000, 0.9238795325112867385, 1.000000000000000000, 0.9238795325112867385, 1.000000000000000000, 0.9238795325112867385, 1.000000000000000000, 0.9238795325112867385, 1.000000000000000000, 0.9238795325112867385, 1.000000000000000000, 0.9238795325112867385, 1.000000000000000000, 0.9238795325112867385, 1.000000000000000000, 0.9238795325112867385, 1.000000000000000000, 0.9238795325112867385, 1.000000000000000000, 0.9238795325112867385, 1.000000000000000000, 0.9238795325112867385, 1.000000000000000000, 0.9238795325112867385, 1.000000000000000000, 0.9238795325112867385, 1.000000000000000000, 0.9238795325112867385, 1.000000000000000000, 0.9238795325112867385, 1.000000000000000000, 0.9238795325112867385, 1.000000000000000000, 0.9238795325112867385, 1.000000000000000000, 0.9238795325112867385, 1.000000000000000000, 0.9238795325112867385, 1.000000000000000000, 0.9238795325112867385, 1.000000000000000000, 0.9238795325112867385, 1.000000000000000000, 0.9238795325112867385, 1.000000000000000000, 0.9238795325112867385, 1.000000000000000000, 0.9238795325112867385, 1.000000000000000000, 0.9238795325112867385, 1.000000000000000000, 0.9238795325112867385, 1.000000000000000000, 0.9238795325112867385, 1.000000000000000000, 0.9238795325112867385, 1.000000000000000000, 0.9238795325112867385, 1.000000000000000000, 0.9238795325112867385, 1.000000000000000000, 0.9238795325112867385, 1.000000000000000000, 0.9238795325112867385, 1.000000000000000000, 0.9238795325112867385, 1.000000000000000000, 0.9238795325112867385, 1.000000000000000000, 0.9238795325112867385, 1.000000000000000000, 0.9238795325112867385, 1.000000000000000000, 0.9238795325112867385, 1.000000000000000000, 0.9238795325112867385, 1.000000000000000000, 0.9238795325112867385, 1.000000000000000000, 0.9238795325112867385, 1.000000000000000000, 0.9238795325112867385, 1.000000000000000000, 0.9238795325112867385, 1.000000000000000000, 0.9238795325112867385, 1.000000000000000000, 0.9238795325112867385, 1.000000000000000000, 0.9238795325112867385, 1.000000000000000000, 0.9238795325112867385, 1.000000000000000000, 0.9238795325112867385, 1.000000000000000000, 0.9238795325112867385, 1.000000000000000000, 0.9238795325112867385, 1.000000000000000000, 0.9238795325112867385, 1.000000000000000000, 0.9238795325112867385, 1.000000000000000000, 0.9238795325112867385, 1.000000000000000000, 0.9238795325112867385, 1.000000000000000000, 0.9238795325112867385, 1.000000000000000000, 0.9238795325112867385, 1.000000000000000000, 0.9238795325112867385, 1.000000000000000000, 0.9238795325112867385, 1.000000000000000000, 0.9238795325112867385, 1.000000000000000000, 0.9238795325112867385, 1.000000000000000000, 0.9238795325112867385, 1.000000000000000000, 0.9238795325112867385, 1.000000000000000000, 0.9238795325112867385, 1.000000000000000000, 0.9238795325112867385, 1.000000000000000000, 0.9238795325112867385, 1.000000000000000000, 0.9238795325112867385, 1.000000000000000000, 0.9238795325112867385, 1.000000000000000000, 0.9238795325112867385, 1.000000000000000000, 0.9238795325112867385, 1.000000000000000000, 0.9238795325112867385, 1.000000000000000000, 0.9238795325112867385, 1.000000000000000000, 0.9238795325112867385, 1.000000000000000000, 0.9238795325112867385, 1.000000000000000000, 0.9238795325112867385, 1.000000000000000000, 0.9238795325112867385, 1.000000000000000000, 0.9238795325112867385, 1.000000000000000000, 0.9238795325112867385, 1.000000000000000000, 0.9238795325112867385, 1.000000000000000000, 0.9238795325112867385, 1.000000000000000000),
 ( 1.000000000000000000, 0.9238795325112867385, 1.000000000000000000, 0.9238795325112867385, 1.000000000000000000, 0.9238795325112867385, 1.000000000000000000, 0.9238795325112867385, 1.000000000000000000, 0.9238795325112867385, 1.000000000000000000, 0.9238795325112867385, 1.000000000000000000, 0.9238795325112867385, 1.000000000000000000, 0.9238795325112867385, 1.000000000000000000, 0.9238795325112867385, 1.000000000000000000, 0.9238795325112867385, 1.000000000000000000, 0.9238795325112867385, 1.000000000000000000, 0.9238795325112867385, 1.000000000000000000, 0.9238795325112867385, 1.000000000000000000, 0.9238795325112867385, 1.000000000000000000, 0.9238795325112867385, 1.000000000000000000, 0.9238795325112867385, 1.000000000000000000, 0.9238795325112867385, 1.000000000000000000, 0.9238795325112867385, 1.000000000000000000, 0.9238795325112867385, 1.000000000000000000, 0.9238795325112867385, 1.000000000000000000, 0.9238795325112867385, 1.000000000000000000, 0.9238795325112867385, 1.000000000000000000, 0.9238795325112867385, 1.000000000000000000, 0.9238795325112867385, 1.000000000000000000, 0.9238795325112867385, 1.000000000000000000, 0.9238795325112867385, 1.000000000000000000, 0.9238795325112867385, 1.000000000000000000, 0.9238795325112867385, 1.000000000000000000, 0.9238795325112867385, 1.000000000000000000, 0.9238795325112867385, 1.000000000000000000, 0.9238795325112867385, 1.000000000000000000, 0.9238795325112867385, 1.000000000000000000, 0.9238795325112867385, 1.000000000000000000, 0.9238795325112867385, 1.000000000000000000, 0.9238795325112867385, 1.000000000000000000, 0.9238795325112867385, 1.000000000000000000, 0.9238795325112867385, 1.000000000000000000, 0.9238795325112867385, 1.000000000000000000, 0.9238795325112867385, 1.000000000000000000, 0.9238795325112867385, 1.000000000000000000, 0.9238795325112867385, 1.000000000000000000, 0.9238795325112867385, 1.000000000000000000, 0.9238795325112867385, 1.000000000000000000, 0.9238795325112867385, 1.000000000000000000, 0.9238795325112867385, 1.000000000000000000, 0.9238795325112867385, 1.000000000000000000, 0.9238795325112867385, 1.000000000000000000, 0.9238795325112867385, 1.000000000000000000, 0.9238795325112867385, 1.000000000000000000, 0.9238795325112867385, 1.000000000000000000, 0.9238795325112867385, 1.000000000000000000, 0.9238795325112867385, 1.000000000000000000, 0.9238795325112867385, 1.000000000000000000, 0.9238795325112867385, 1.000000000000000000, 0.9238795325112867385, 1.000000000000000000, 0.9238795325112867385, 1.000000000000000000, 0.9238795325112867385, 1.000000000000000000, 0.9238795325112867385, 1.000000000000000000, 0.9238795325112867385, 1.000000000000000000, 0.9238795325112867385, 1.000000000000000000, 0.9238795325112867385, 1.000000000000000000, 0.9238795325112867385, 1.000000000000000000, 0.9238795325112867385, 1.000000000000000000, 0.9238795325112867385, 1.000000000000000000, 0.9238795325112867385, 1.000000000000000000, 0.9238795325112867385, 1.000000000000000000, 0.9238795325112867385, 1.000000000000000000, 0.9238795325112867385, 1.000000000000000000, 0.9238795325112867385, 1.000000000000000000, 0.9238795325112867385, 1.000000000000000000, 0.9238795325112867385, 1.000000000000000000, 0.9238795325112867385, 1.000000000000000000, 0.9238795325112867385, 1.000000000000000000, 0.9238795325112867385, 1.000000000000000000, 0.9238795325112867385, 1.000000000000000000, 0.9238795325112867385, 1.000000000000000000, 0.9238795325112867385, 1.000000000000000000, 0.9238795325112867385, 1.000000000000000000, 0.9238795325112867385, 1.000000000000000000, 0.9238795325112867385, 1.000000000000000000, 0.9238795325112867385, 1.000000000000000000, 0.9238795325112867385, 1.000000000000000000, 0.9238795325112867385, 1.000000000000000000, 0.9238795325112867385, 1.000000000000000000, 0.9238795325112867385, 1.000000000000000000, 0.9238795325112867385, 1.000000000000000000, 0.9238795325112867385, 1.000000000000000000, 0.9238795325112867385, 1.000000000000000000, 0.9238795325112867385, 1.000000000000000000, 0.9238795325112867385, 1.000000000000000000, 0.9238795325112867385, 1.000000000000000000, 0.9238795325112867385, 1.000000000000000000, 0.9238795325112867385, 1.000000000000000000, 0.9238795325112867385, 1.000000000000000000, 0.9238795325112867385, 1.000000000000000000, 0.9238795325112867385, 1.000000000000000000, 0.9238795325112867385, 1.000000000000000000, 0.9238795325112867385, 1.000000000000000000, 0.9238795325112867385, 1.000000000000000000, 0.9238795325112867385, 1.000000000000000000, 0.9238795325112867385, 1.000000000000000000, 0.9238795325112867385, 1.000000000000000000, 0.9238795325112867385, 1.000000000000000000, 0.9238795325112867385, 1.000000000000000000, 0.9238795325112867385, 1.000000000000000000, 0.9238795325112867385, 1.000000000000000000, 0.9238795325112867385, 1.000000000000000000, 0.9238795325112867385, 1.000000000000000000, 0.9238795325112867385, 1.000000000000000000, 0.9238795325112867385, 1.000000000000000000, 0.9238795325112867385, 1.000000000000000000, 0.9238795325112867385, 1.000000000000000000, 0.9238795325112867385, 1.000000000000000000, 0.9238795325112867385, 1.000000000000000000, 0.9238795325112867385, 1.000000000000000000, 0.9238795325112867385, 1.000000000000000000, 0.9238795325112867385, 1.000000000000000000, 0.9238795325112867385, 1.000000000000000000, 0.9238795325112867385, 1.000000000000000000, 0.9238795325112867385, 1.000000000000000000, 0.9238795325112867385, 1.000000000000000000, 0.9238795325112867385, 1.000000000000000000, 0.9238795325112867385, 1.000000000000000000, 0.9238795325112867385, 1.000000000000000000, 0.9238795325112867385, 1.000000000000000000, 0.9238795325112867385, 1.000000000000000000, 0.9238795325112867385, 1.000000000000000000, 0.9238795325112867385, 1.000000000000000000, 0.9238795325112867385, 1.000000000000000000, 0.9238795325112867385, 1.000000000000000000, 0.9238795325112867385, 1.000000000000000000, 0.9238795325112867385, 1.000000000000000000, 0.9238795325112867385, 1.000000000000000000, 0.9238795325112867385, 1.000000000000000000, 0.9238795325112867385, 1.000000000000000000, 0.9238795325112867385, 1.000000000000000000, 0.9238795325112867385, 1.000000000000000000, 0.9238795325112867385, 1.000000000000000000, 0.9238795325112867385, 1.000000000000000000, 0.9238795325112867385, 1.000000000000000000, 0.9238795325112867385, 1.000000000000000000, 0.9238795325112867385, 1.000000000000000000, 0.9238795325112867385, 1.000000000000000000, 0.9238795325112867385, 1.000000000000000000, 0.9238795325112867385, 1.000000000000000000, 0.9238795325112867385, 1.000000000000000000, 0.9238795325112867385, 1.000000000000000000, 0.9238795325112867385, 1.000000000000000000, 0.9238795325112867385, 1.000000000000000000, 0.9238795325112867385, 1.000000000000000000, 0.9238795325112867385, 1.000000000000000000, 0.9238795325112867385, 1.000000000000000000, 0.9238795325112867385, 1.000000000000000000, 0.9238795325112867385, 1.000000000000000000, 0.9238795325112867385, 1.000000000000000000, 0.9238795325112867385, 1.000000000000000000, 0.9238795325112867385, 1.000000000000000000, 0.9238795325112867385, 1.000000000000000000, 0.9238795325112867385, 1.000000000000000000, 0.9238795325112867385, 1.000000000000000000, 0.9238795325112867385, 1.000000000000000000, 0.9238795325112867385, 1.000000000000000000, 0.9238795325112867385, 1.000000000000000000, 0.9238795325112867385, 1.000000000000000000, 0.9238795325112867385, 1.000000000000000000, 0.9238795325112867385, 1.000000000000000000, 0.9238795325112867385, 1.000000000000000000, 0.9238795325112867385, 1.000000000000000000, 0.9238795325112867385, 1.000000000000000000, 0.9238795325112867385, 1.000000000000000000, 0.9238795325112867385, 1.000000000000000000, 0.9238795325112867385, 1.000000000000000000, 0.9238795325112867385, 1.000000000000000000, 0.9238795325112867385, 1.000000000000000000, 0.9238795325112867385, 1.000000000000000000, 0.9238795325112867385, 1.000000000000000000, 0.9238795325112867385, 1.000000000000000000, 0.9238795325112867385, 1.000000000000000000, 0.9238795325112867385, 1.000000000000000000, 0.9238795325112867385, 1.000000000000000000, 0.9238795325112867385, 1.000000000000000000, 0.9238795325112867385, 1.000000000000000000, 0.9238795325112867385, 1.000000000000000000, 0.9238795325112867385, 1.000000000000000000, 0.9238795325112867385, 1.000000000000000000, 0.9238795325112867385, 1.000000000000000000, 0.9238795325112867385, 1.000000000000000000, 0.9238795325112867385, 1.000000000000000000, 0.9238795325112867385, 1.000000000000000000, 0.9238795325112867385, 1.000000000000000000, 0.9238795325112867385, 1.000000000000000000, 0.9238795325112867385, 1.000000000000000000, 0.9238795325112867385, 1.000000000000000000, 0.9238795325112867385, 1.000000000000000000, 0.9238795325112867385, 1.000000000000000000, 0.9238795325112867385, 1.000000000000000000, 0.9238795325112867385, 1.000000000000000000, 0.9238795325112867385, 1.000000000000000000, 0.9238795325112867385, 1.000000000000000000, 0.9238795325112867385, 1.000000000000000000, 0.9238795325112867385, 1.000000000000000000, 0.9238795325112867385, 1.000000000000000000, 0.9238795325112867385, 1.000000000000000000, 0.9238795325112867385, 1.000000000000000000, 0.9238795325112867385, 1.000000000000000000, 0.9238795325112867385, 1.000000000000000000, 0.9238795325112867385, 1.000000000000000000, 0.9238795325112867385, 1.000000000000000000, 0.9238795325112867385, 1.000000000000000000, 0.9238795325112867385, 1.000000000000000000, 0.9238795325112867385, 1.000000000000000000, 0.9238795325112867385, 1.000000000000000000, 0.9238795325112867385, 1.000000000000000000, 0.9238795325112867385, 1.000000000000000000, 0.9238795325112867385, 1.000000000000000000, 0.9238795325112867385, 1.000000000000000000, 0.9238795325112867385, 1.000000000000000000, 0.9238795325112867385, 1.000000000000000000, 0.9238795325112867385, 1.000000000000000000, 0.9238795325112867385, 1.000000000000000000, 0.9238795325112867385, 1.000000000000000000, 0.9238795325112867385, 1.000000000000000000, 0.9238795325112867385, 1.000000000000000000, 0.9238795325112867385, 1.000000000000000000, 0.9238795325112867385, 1.000000000000000000, 0.9238795325112867385, 1.000000000000000000, 0.9238795325112867385, 1.000000000000000000, 0.9238795325112867385, 1.000000000000000000, 0.9238795325112867385, 1.000000000000000000, 0.9238795325112867385, 1.000000000000000000, 0.9238795325112867385, 1.000000000000000000, 0.9238795325112867385, 1.000000000000000000, 0.9238795325112867385, 1.000000000000000000, 0.9238795325112867385, 1.000000000000000000, 0.9238795325112867385, 1.000000000000000000, 0.9238795325112867385, 1.000000000000000000, 0.9238795325112867385, 1.000000000000000000, 0.9238795325112867385, 1.000000000000000000, 0.9238795325112867385, 1.000000000000000000, 0.9238795325112867385, 1.000000000000000000) ) ) 
 REPRESENTATION_ITEM ( '' )  SURFACE ( )  );
#17093=CARTESIAN_POINT ( 'NONE',  ( -52.80376928212989185, -134.1250000013656347, -4.297418129356379346 ) ) ;
#17136=CARTESIAN_POINT ( 'NONE',  ( -52.10840900171896806, -139.4375000013656063, 3.393966926194110556 ) ) ;
#17164=CARTESIAN_POINT ( 'NONE',  ( -50.40829686548195099, -145.2500000013656347, -1.485763867205728284 ) ) ;
#17184=CARTESIAN_POINT ( 'NONE',  ( -59.29741812935640155, -149.6250000013655779, -2.196230717870135685 ) ) ;
#17208=CARTESIAN_POINT ( 'NONE',  ( -57.89159099828107458, -152.9375000013656063, -3.393966926194107447 ) ) ;
#17231=FACE_OUTER_BOUND ( 'NONE', #30934, .T. ) ;
#17249=CARTESIAN_POINT ( 'NONE',  ( -56.66612745406270335, -138.3125000000000000, -5.149110718188516067 ) ) ;
#17252=EDGE_LOOP ( 'NONE', ( #3423, #42844, #31379, #39314 ) ) ;
#17259=CARTESIAN_POINT ( 'NONE',  ( -50.70258187064364108, -144.3750000013656063, 2.196230717870141014 ) ) ;
#17261=CARTESIAN_POINT ( 'NONE',  ( -51.19402409849444524, -131.6250000027312126, -3.242614290531456334 ) ) ;
#17286=CARTESIAN_POINT ( 'NONE',  ( -58.39396692619412477, -132.4375000013656063, 2.891590998281057701 ) ) ;
#17295=CARTESIAN_POINT ( 'NONE',  ( -50.55543936806279248, -126.3125000013655921, 0.3552334253322060320 ) ) ;
#17301=DIRECTION ( 'NONE',  ( 0.000000000000000000, 1.000000000000000000, 0.000000000000000000 ) ) ;
#17327=CARTESIAN_POINT ( 'NONE',  ( -57.89159099828107458, -140.6875000013656063, -3.393966926194107447 ) ) ;
#17332=CARTESIAN_POINT ( 'NONE',  ( -50.18089887299979068, -148.6875000000000568, 2.462841084822635640 ) ) ;
#17333=EDGE_CURVE ( 'NONE', #24403, #40939, #16171, .T. ) ;
#17343=CARTESIAN_POINT ( 'NONE',  ( -57.19623071787016499, -153.6250000013655779, 4.297418129356382899 ) ) ;
#17344=CARTESIAN_POINT ( 'NONE',  ( -56.66612745406270335, -143.4375000027312410, -5.149110718188516067 ) ) ;
#17351=CARTESIAN_POINT ( 'NONE',  ( -55.35523342533222291, -136.3125000013656063, 4.444560631937231499 ) ) ;
#17368=CARTESIAN_POINT ( 'NONE',  ( -51.60603307380591787, -146.9375000013656063, -2.891590998281053704 ) ) ;
#17372=CARTESIAN_POINT ( 'NONE',  ( -56.66612745406280993, -148.3125000000000000, -5.149110718188524061 ) ) ;
#17420=CARTESIAN_POINT ( 'NONE',  ( -50.70258187064364108, -131.3750000013656347, 2.196230717870141014 ) ) ;
#17462=CARTESIAN_POINT ( 'NONE',  ( -59.44456063193725015, -140.8125000013656063, -0.3552334253322034230 ) ) ;
#17494=CARTESIAN_POINT ( 'NONE',  ( -50.55543936806279248, -146.3125000013656063, 0.3552334253322060320 ) ) ;
#17497=EDGE_LOOP ( 'NONE', ( #57513, #18903, #16150, #18431 ) ) ;
#17499=ORIENTED_EDGE ( 'NONE', *, *, #53609, .F. ) ;
#17514=CARTESIAN_POINT ( 'NONE',  ( -57.89159099828107458, -150.6875000013656063, -3.393966926194107447 ) ) ;
#17528=DIRECTION ( 'NONE',  ( 0.000000000000000000, 1.000000000000000000, 0.000000000000000000 ) ) ;
#17539=CARTESIAN_POINT ( 'NONE',  ( -59.29741812935640155, -151.8750000013655779, -2.196230717870135685 ) ) ;
#17575=CARTESIAN_POINT ( 'NONE',  ( -51.75738570946856498, -135.7500000000000284, 3.805975901505576964 ) ) ;
#17585=CYLINDRICAL_SURFACE ( 'NONE', #53116, 5.000000000000000000 ) ;
#17586=CARTESIAN_POINT ( 'NONE',  ( -56.48576386720575471, -139.0000000013655779, -4.591703134518078322 ) ) ;
#17588=CARTESIAN_POINT ( 'NONE',  ( -58.80597590150559739, -132.1250000027312126, 3.242614290531460330 ) ) ;
#17600=CARTESIAN_POINT ( 'NONE',  ( -59.81910112700025905, -154.1875000000000284, -2.462841084822619209 ) ) ;
#17612=CARTESIAN_POINT ( 'NONE',  ( -55.35523342533222291, -134.3125000013656063, 4.444560631937231499 ) ) ;
#17620=ORIENTED_EDGE ( 'NONE', *, *, #24837, .T. ) ;
#17622=CARTESIAN_POINT ( 'NONE',  ( -52.80376928212989185, -126.1250000013656205, -4.297418129356379346 ) ) ;
#17628=CARTESIAN_POINT ( 'NONE',  ( -50.18089887299976937, -137.8125000027312126, 2.462841084822337656 ) ) ;
#17633=VERTEX_POINT ( 'NONE', #774 ) ;
#17642=ORIENTED_EDGE ( 'NONE', *, *, #63242, .T. ) ;
#17643=CARTESIAN_POINT ( 'NONE',  ( -53.51423613279429503, -154.5000000013655779, 4.591703134518082763 ) ) ;
#17647=CARTESIAN_POINT ( 'NONE',  ( -55.35523342533222291, -137.3125000013656063, 4.444560631937231499 ) ) ;
#17648=AXIS2_PLACEMENT_3D ( 'NONE', #5224, #20338, #10363 ) ;
#17653=CARTESIAN_POINT ( 'NONE',  ( -59.98410592259440222, -149.1250000000000284, -0.3983568153799752487 ) ) ;
#17662=CARTESIAN_POINT ( 'NONE',  ( -54.64476657466781973, -153.0625000013656063, -4.444560631937228834 ) ) ;
#17663=CARTESIAN_POINT ( 'NONE',  ( -49.85088928181150436, -143.6875000027312126, -1.666127454062680702 ) ) ;
#17664=EDGE_CURVE ( 'NONE', #57381, #27617, #29693, .T. ) ;
#17672=CARTESIAN_POINT ( 'NONE',  ( -52.80376928212989185, -137.8750000013655779, -4.297418129356379346 ) ) ;
#17686=CARTESIAN_POINT ( 'NONE',  ( -56.48576386720575471, -145.7500000013655779, -4.591703134518078322 ) ) ;
#17711=DIRECTION ( 'NONE',  ( -0.6485228581062915110, 0.000000000000000000, -0.7611951803011149931 ) ) ;
#17725=CARTESIAN_POINT ( 'NONE',  ( -59.59170313451811296, -130.7500000013656063, 1.485763867205729394 ) ) ;
#17755=CARTESIAN_POINT ( 'NONE',  ( -50.01589407740564042, -138.6250000000000284, 0.3983568153799778022 ) ) ;
#17768=CARTESIAN_POINT ( 'NONE',  ( -57.89159099828107458, -135.9375000013656063, -3.393966926194107447 ) ) ;
#17796=CARTESIAN_POINT ( 'NONE',  ( -56.48576386720575471, -142.0000000013656063, -4.591703134518078322 ) ) ;
#17807=CARTESIAN_POINT ( 'NONE',  ( -49.85088928181150436, -126.5625000000000426, -1.666127454062680702 ) ) ;
#17816=CARTESIAN_POINT ( 'NONE',  ( -55.35523342533222291, -150.3125000013656063, 4.444560631937231499 ) ) ;
#17834=ORIENTED_EDGE ( 'NONE', *, *, #48322, .F. ) ;
#17842=CARTESIAN_POINT ( 'NONE',  ( -50.70258187064364108, -147.3750000013656063, 2.196230717870141014 ) ) ;
#17865=DIRECTION ( 'NONE',  ( 1.387778780781445676E-15, 0.000000000000000000, -1.000000000000000000 ) ) ;
#17875=VERTEX_POINT ( 'NONE', #38872 ) ;
#17880=CARTESIAN_POINT ( 'NONE',  ( -60.14911071818854538, -138.0625000000000000, 1.666127454062681368 ) ) ;
#17889=CARTESIAN_POINT ( 'NONE',  ( -53.51423613279429503, -139.5000000013656063, 4.591703134518083651 ) ) ;
#17891=CARTESIAN_POINT ( 'NONE',  ( -57.46284108482265651, -131.0625000027312410, 4.819101127000239515 ) ) ;
#17900=CARTESIAN_POINT ( 'NONE',  ( -60.14911071818854538, -154.0625000000000000, 1.666127454062681146 ) ) ;
#17904=( BOUNDED_CURVE ( )  B_SPLINE_CURVE ( 2, ( #18869, #17628, #48145, #3157, #4097, #23720, #2840, #38486, #58113 ),
 .UNSPECIFIED., .F., .F. ) 
 B_SPLINE_CURVE_WITH_KNOTS ( ( 3, 2, 2, 2, 3 ),
 ( 0.5416666666666671848, 0.5458333333333338366, 0.5500000000000004885, 0.5541666666666671404, 0.5583333333333337922 ),
 .UNSPECIFIED. ) 
 CURVE ( )  GEOMETRIC_REPRESENTATION_ITEM ( )  RATIONAL_B_SPLINE_CURVE ( ( 0.9999999999999898970, 0.9238795325112968415, 1.000000000000000000, 0.9238795325112867385, 1.000000000000000000, 0.9238795325112867385, 1.000000000000000000, 0.9238795325112786339, 1.000000000000008216 ) ) 
 REPRESENTATION_ITEM ( '' )  );
#17914=CARTESIAN_POINT ( 'NONE',  ( -50.55543936806279248, -132.0625000013656063, 0.3552334253322060320 ) ) ;
#17923=CARTESIAN_POINT ( 'NONE',  ( -55.35523342533222291, -127.5625000013655921, 4.444560631937231499 ) ) ;
#17943=CARTESIAN_POINT ( 'NONE',  ( -57.19623071787017210, -154.6250000013656063, 4.297418129356382899 ) ) ;
#17947=CARTESIAN_POINT ( 'NONE',  ( -58.39396692619412477, -140.4375000013656063, 2.891590998281057701 ) ) ;
#17953=CARTESIAN_POINT ( 'NONE',  ( -52.53715891517739323, -148.4375000000000284, -4.819101127000233298 ) ) ;
#17962=CARTESIAN_POINT ( 'NONE',  ( -54.64476657466781973, -151.0625000013656063, -4.444560631937228834 ) ) ;
#17963=CARTESIAN_POINT ( 'NONE',  ( -50.01589407740564042, -141.7500000027312126, 0.3983568153799778022 ) ) ;
#17969=CARTESIAN_POINT ( 'NONE',  ( -59.59170313451811296, -135.5000000013656063, 1.485763867205729394 ) ) ;
#17985=CARTESIAN_POINT ( 'NONE',  ( -59.59170313451811296, -144.5000000013656063, 1.485763867205729394 ) ) ;
#18031=CARTESIAN_POINT ( 'NONE',  ( -50.55543936806279248, -129.3125000013656063, 0.3552334253322060320 ) ) ;
#18076=CARTESIAN_POINT ( 'NONE',  ( -50.40829686548195099, -137.2500000013656063, -1.485763867205728284 ) ) ;
#18086=VERTEX_POINT ( 'NONE', #33742 ) ;
#18110=CARTESIAN_POINT ( 'NONE',  ( -50.55543936806279248, -143.3125000013656063, 0.3552334253322060320 ) ) ;
#18127=CARTESIAN_POINT ( 'NONE',  ( -53.51423613279429503, -143.2500000013656063, 4.591703134518082763 ) ) ;
#18128=DIRECTION ( 'NONE',  ( 0.000000000000000000, 1.000000000000000000, 0.000000000000000000 ) ) ;
#18143=CARTESIAN_POINT ( 'NONE',  ( -50.18089887299976937, -139.6875000000000000, 2.462841084822397164 ) ) ;
#18146=CARTESIAN_POINT ( 'NONE',  ( -58.24261429053147765, -155.0000000000000284, -3.805975901505573411 ) ) ;
#18153=CARTESIAN_POINT ( 'NONE',  ( -53.51423613279429503, -149.5000000013655779, 4.591703134518082763 ) ) ;
#18178=ADVANCED_FACE ( 'NONE', ( #5746 ), #34689, .F. ) ;
#18179=ORIENTED_EDGE ( 'NONE', *, *, #38613, .T. ) ;
#18187=EDGE_CURVE ( 'NONE', #19422, #24361, #29531, .T. ) ;
#18190=( BOUNDED_CURVE ( )  B_SPLINE_CURVE ( 2, ( #44306, #60083, #24383, #43984, #49137, #39482, #6052, #20195, #19868 ),
 .UNSPECIFIED., .F., .F. ) 
 B_SPLINE_CURVE_WITH_KNOTS ( ( 3, 2, 2, 2, 3 ),
 ( 0.2583333333333335813, 0.2625000000000002331, 0.2666666666666668850, 0.2708333333333335369, 0.2750000000000002442 ),
 .UNSPECIFIED. ) 
 CURVE ( )  GEOMETRIC_REPRESENTATION_ITEM ( )  RATIONAL_B_SPLINE_CURVE ( ( 0.9999999999999958922, 0.9238795325112908463, 1.000000000000000000, 0.9238795325112867385, 1.000000000000000000, 0.9238795325112867385, 1.000000000000000000, 0.9238795325112826307, 1.000000000000003997 ) ) 
 REPRESENTATION_ITEM ( '' )  );
#18199=CARTESIAN_POINT ( 'NONE',  ( -58.24261429053147765, -136.2500000000000284, -3.805975901505573855 ) ) ;
#18201=EDGE_LOOP ( 'NONE', ( #10644, #50862, #14999, #1630 ) ) ;
#18207=CARTESIAN_POINT ( 'NONE',  ( -52.10840900171896806, -139.4375000013656063, 3.393966926194110556 ) ) ;
#18209=CARTESIAN_POINT ( 'NONE',  ( -51.75738570946856498, -128.8750000027312126, 3.805975901505576964 ) ) ;
#18220=CARTESIAN_POINT ( 'NONE',  ( -54.64476657466781973, -126.8125000013655921, -4.444560631937228834 ) ) ;
#18229=AXIS2_PLACEMENT_3D ( 'NONE', #62383, #42739, #18305 ) ;
#18231=CARTESIAN_POINT ( 'NONE',  ( -50.55543936806279248, -130.0625000013656063, 0.3552334253322060320 ) ) ;
#18244=CARTESIAN_POINT ( 'NONE',  ( -54.64476657466781973, -129.0625000013656063, -4.444560631937228834 ) ) ;
#18265=PLANE ( 'NONE',  #20017 ) ;
#18269=CARTESIAN_POINT ( 'NONE',  ( -50.75781946612335105, -135.0000000000005969, -1.372666862511563224 ) ) ;
#18275=CARTESIAN_POINT ( 'NONE',  ( -58.80597590150559739, -148.0000000000000284, 3.242614290531460330 ) ) ;
#18283=CARTESIAN_POINT ( 'NONE',  ( -57.46284108482265651, -135.0625000027312410, 4.819101127000238627 ) ) ;
#18284=ORIENTED_EDGE ( 'NONE', *, *, #542, .F. ) ;
#18285=CARTESIAN_POINT ( 'NONE',  ( -57.89159099828107458, -148.9375000013656063, -3.393966926194107447 ) ) ;
#18286=CARTESIAN_POINT ( 'NONE',  ( -52.53715891517739323, -143.5625000027312126, -4.819101127000233298 ) ) ;
#18287=VECTOR ( 'NONE', #22881, 1000.000000000000000 ) ;
#18295=CARTESIAN_POINT ( 'NONE',  ( -57.89159099828107458, -138.6875000013656347, -3.393966926194107447 ) ) ;
#18305=DIRECTION ( 'NONE',  ( -0.7611951803011147710, 0.000000000000000000, 0.6485228581062916220 ) ) ;
#18308=CYLINDRICAL_SURFACE ( 'NONE', #44804, 5.000000000000000000 ) ;
#18309=CARTESIAN_POINT ( 'NONE',  ( -56.48576386720575471, -141.7500000013656063, -4.591703134518078322 ) ) ;
#18329=DIRECTION ( 'NONE',  ( -0.6485228581062915110, 0.000000000000000000, -0.7611951803011149931 ) ) ;
#18338=FACE_OUTER_BOUND ( 'NONE', #50555, .T. ) ;
#18352=CARTESIAN_POINT ( 'NONE',  ( -51.60603307380591787, -131.1875000013656063, -2.891590998281053704 ) ) ;
#18359=CARTESIAN_POINT ( 'NONE',  ( -50.01589407740564042, -152.7500000027312410, 0.3983568153799778022 ) ) ;
#18398=CARTESIAN_POINT ( 'NONE',  ( -55.35523342533222291, -135.5625000013656063, 4.444560631937231499 ) ) ;
#18427=CARTESIAN_POINT ( 'NONE',  ( -59.59170313451811296, -141.7500000013656063, 1.485763867205729394 ) ) ;
#18431=ORIENTED_EDGE ( 'NONE', *, *, #42428, .F. ) ;
#18447=CARTESIAN_POINT ( 'NONE',  ( -50.40829686548195099, -147.0000000013655779, -1.485763867205728284 ) ) ;
#18476=CARTESIAN_POINT ( 'NONE',  ( -59.44456063193725015, -147.8125000013656063, -0.3552334253322034230 ) ) ;
#18480=CARTESIAN_POINT ( 'NONE',  ( -53.33387254593751692, -136.8125000000000284, 5.149110718188503633 ) ) ;
#18505=AXIS2_PLACEMENT_3D ( 'NONE', #50856, #6800, #42455 ) ;
#18514=CARTESIAN_POINT ( 'NONE',  ( -60.14911071818854538, -135.0625000000000284, 1.666127454062681368 ) ) ;
#18518=ADVANCED_FACE ( 'NONE', ( #30828 ), #35978, .F. ) ;
#18524=CARTESIAN_POINT ( 'NONE',  ( -54.64476657466781973, -140.0625000013656063, -4.444560631937228834 ) ) ;
#18526=CARTESIAN_POINT ( 'NONE',  ( -53.33387254593733928, -125.9375000027312268, 5.149110718188519620 ) ) ;
#18534=FACE_OUTER_BOUND ( 'NONE', #29184, .T. ) ;
#18544=ORIENTED_EDGE ( 'NONE', *, *, #50419, .F. ) ;
#18551=CARTESIAN_POINT ( 'NONE',  ( -50.70258187064364108, -128.1250000013656347, 2.196230717870141014 ) ) ;
#18568=LINE ( 'NONE', #33357, #21589 ) ;
#18575=CARTESIAN_POINT ( 'NONE',  ( -52.53715891517739323, -144.5625000027311842, -4.819101127000233298 ) ) ;
#18582=CARTESIAN_POINT ( 'NONE',  ( -59.44456063193725015, -150.8125000013656063, -0.3552334253322034230 ) ) ;
#18592=CARTESIAN_POINT ( 'NONE',  ( -59.81910112700025905, -150.1875000000000284, -2.462841084822630311 ) ) ;
#18602=CARTESIAN_POINT ( 'NONE',  ( -59.29741812935640155, -151.8750000013655779, -2.196230717870135685 ) ) ;
#18603=CARTESIAN_POINT ( 'NONE',  ( -58.24261429053147765, -139.3750000027312126, -3.805975901505573855 ) ) ;
#18610=CARTESIAN_POINT ( 'NONE',  ( -53.51423613279429503, -137.2500000013656063, 4.591703134518082763 ) ) ;
#18628=CARTESIAN_POINT ( 'NONE',  ( -50.70258187064364108, -143.1250000013656063, 2.196230717870141014 ) ) ;
#18659=CARTESIAN_POINT ( 'NONE',  ( -54.64476657466781973, -151.8125000013656063, -4.444560631937228834 ) ) ;
#18666=CARTESIAN_POINT ( 'NONE',  ( -54.64476657466781973, -131.0625000013656063, -4.444560631937228834 ) ) ;
#18673=ORIENTED_EDGE ( 'NONE', *, *, #51136, .F. ) ;
#18691=CARTESIAN_POINT ( 'NONE',  ( -59.59170313451811296, -152.5000000013655779, 1.485763867205729394 ) ) ;
#18705=CARTESIAN_POINT ( 'NONE',  ( -54.64476657466781973, -134.0625000013656063, -4.444560631937228834 ) ) ;
#18713=CARTESIAN_POINT ( 'NONE',  ( -59.54425679209026612, -135.0000000000000284, 1.880628494755099522 ) ) ;
#18714=ORIENTED_EDGE ( 'NONE', *, *, #37498, .F. ) ;
#18734=CARTESIAN_POINT ( 'NONE',  ( -55.35523342533222291, -141.5625000013656063, 4.444560631937231499 ) ) ;
#18751=CARTESIAN_POINT ( 'NONE',  ( -51.60603307380591787, -146.9375000013656063, -2.891590998281053704 ) ) ;
#18752=CARTESIAN_POINT ( 'NONE',  ( -51.75738570946856498, -155.0000000000000284, 3.805975901505577408 ) ) ;
#18761=CARTESIAN_POINT ( 'NONE',  ( -60.14911071818854538, -142.0625000000000000, 1.666127454062681146 ) ) ;
#18764=CARTESIAN_POINT ( 'NONE',  ( -50.01589407740564042, -146.6250000000000284, 0.3983568153799778022 ) ) ;
#18774=CARTESIAN_POINT ( 'NONE',  ( -50.55543936806279248, -148.3125000013656063, 0.3552334253322060320 ) ) ;
#18804=EDGE_CURVE ( 'NONE', #24403, #58682, #18568, .T. ) ;
#18811=CARTESIAN_POINT ( 'NONE',  ( -51.19402409849444524, -133.5000000000000284, -3.242614290531456334 ) ) ;
#18819=DIRECTION ( 'NONE',  ( 0.000000000000000000, 1.000000000000000000, 0.000000000000000000 ) ) ;
#18821=CARTESIAN_POINT ( 'NONE',  ( -50.40829686548195099, -137.2500000013656063, -1.485763867205728284 ) ) ;
#18823=CARTESIAN_POINT ( 'NONE',  ( -51.75738570946856498, -124.8750000027312126, 3.805975901505576964 ) ) ;
#18825=CARTESIAN_POINT ( 'NONE',  ( -50.51982268314063873, -135.0000000000000000, 1.105932492512590404 ) ) ;
#18847=CARTESIAN_POINT ( 'NONE',  ( -50.40829686548195099, -131.0000000013656063, -1.485763867205728284 ) ) ;
#18848=CARTESIAN_POINT ( 'NONE',  ( -52.10840900171896806, -146.1875000013656063, 3.393966926194110556 ) ) ;
#18869=CARTESIAN_POINT ( 'NONE',  ( -51.75738570946856498, -137.8750000027312126, 3.805975901505576964 ) ) ;
#18878=FACE_OUTER_BOUND ( 'NONE', #31348, .T. ) ;
#18885=CARTESIAN_POINT ( 'NONE',  ( -55.35523342533222291, -150.5625000013656063, 4.444560631937231499 ) ) ;
#18895=CARTESIAN_POINT ( 'NONE',  ( -51.19402409849444524, -144.5000000000000284, -3.242614290531456334 ) ) ;
#18903=ORIENTED_EDGE ( 'NONE', *, *, #44439, .T. ) ;
#18904=CARTESIAN_POINT ( 'NONE',  ( -59.29741812935640155, -150.8750000013656063, -2.196230717870135685 ) ) ;
#18905=CARTESIAN_POINT ( 'NONE',  ( -51.19402409849444524, -140.6250000027312126, -3.242614290531456334 ) ) ;
#18914=CARTESIAN_POINT ( 'NONE',  ( -59.44456063193725015, -131.5625000013656063, -0.3552334253322034230 ) ) ;
#18928=CARTESIAN_POINT ( 'NONE',  ( -50.55543936806279248, -143.0625000013656063, 0.3552334253322060320 ) ) ;
#18938=CARTESIAN_POINT ( 'NONE',  ( -51.75738570946856498, -148.7500000000000284, 3.805975901505576964 ) ) ;
#18961=CARTESIAN_POINT ( 'NONE',  ( -51.60603307380591787, -153.9375000013656063, -2.891590998281053704 ) ) ;
#18969=CARTESIAN_POINT ( 'NONE',  ( -51.60603307380591787, -127.1875000013656063, -2.891590998281053704 ) ) ;
#18976=CARTESIAN_POINT ( 'NONE',  ( -58.24261429053147765, -143.2500000000000284, -3.805975901505573855 ) ) ;
#18980=CARTESIAN_POINT ( 'NONE',  ( -54.60164318462004474, -149.5000000027312126, -4.984105922594373794 ) ) ;
#18985=LINE ( 'NONE', #48255, #41099 ) ;
#18993=CARTESIAN_POINT ( 'NONE',  ( -58.24261429053147765, -137.3750000027312126, -3.805975901505573855 ) ) ;
#18999=CARTESIAN_POINT ( 'NONE',  ( -58.39396692619412477, -154.4375000013656063, 2.891590998281057701 ) ) ;
#19001=DIRECTION ( 'NONE',  ( 0.000000000000000000, -0.000000000000000000, -1.000000000000000000 ) ) ;
#19015=CARTESIAN_POINT ( 'NONE',  ( -59.29741812935640155, -136.8750000013656063, -2.196230717870135685 ) ) ;
#19036=CARTESIAN_POINT ( 'NONE',  ( -49.85088928181150436, -136.5625000000000284, -1.666127454062680480 ) ) ;
#19044=CARTESIAN_POINT ( 'NONE',  ( -50.40829686548195099, -137.2500000013656063, -1.485763867205728284 ) ) ;
#19050=CARTESIAN_POINT ( 'NONE',  ( -53.33387254593725402, -147.9375000027312126, 5.149110718188524949 ) ) ;
#19060=CARTESIAN_POINT ( 'NONE',  ( -50.55543936806279248, -146.0625000013656063, 0.3552334253322060320 ) ) ;
#19070=CARTESIAN_POINT ( 'NONE',  ( -53.33387254593711901, -141.8124999999999432, 5.149110718188534719 ) ) ;
#19078=CARTESIAN_POINT ( 'NONE',  ( -59.98410592259440222, -144.1250000000000284, -0.3983568153799752487 ) ) ;
#19085=CARTESIAN_POINT ( 'NONE',  ( -57.19623071787017210, -146.6250000013656063, 4.297418129356382899 ) ) ;
#19124=CARTESIAN_POINT ( 'NONE',  ( -58.80597590150559739, -135.0000000000000284, 3.242614290531460330 ) ) ;
#19135=CARTESIAN_POINT ( 'NONE',  ( -54.60164318462004474, -127.5000000027312126, -4.984105922594373794 ) ) ;
#19158=CARTESIAN_POINT ( 'NONE',  ( -58.39396692619412477, -131.4375000013656063, 2.891590998281057701 ) ) ;
#19160=CARTESIAN_POINT ( 'NONE',  ( -52.10840900171896806, -145.1875000013656063, 3.393966926194110556 ) ) ;
#19179=AXIS2_PLACEMENT_3D ( 'NONE', #57489, #7647, #57174 ) ;
#19196=CARTESIAN_POINT ( 'NONE',  ( -59.59170313451811296, -152.7500000013655779, 1.485763867205729394 ) ) ;
#19205=VERTEX_POINT ( 'NONE', #12718 ) ;
#19206=CARTESIAN_POINT ( 'NONE',  ( -54.60164318462004474, -145.3750000000000284, -4.984105922594373794 ) ) ;
#19214=CARTESIAN_POINT ( 'NONE',  ( -52.80376928212989185, -149.1250000013656063, -4.297418129356378458 ) ) ;
#19215=CARTESIAN_POINT ( 'NONE',  ( -57.46284108482265651, -139.0625000027312126, 4.819101127000239515 ) ) ;
#19229=CARTESIAN_POINT ( 'NONE',  ( -51.60603307380591787, -134.9375000013656063, -2.891590998281053704 ) ) ;
#19244=CARTESIAN_POINT ( 'NONE',  ( -56.48576386720575471, -142.7500000013656063, -4.591703134518078322 ) ) ;
#19257=CARTESIAN_POINT ( 'NONE',  ( -53.33387254593731086, -152.9375000027312126, 5.149110718188520508 ) ) ;
#19278=CARTESIAN_POINT ( 'NONE',  ( -55.35523342533222291, -152.3125000013656063, 4.444560631937231499 ) ) ;
#19286=CARTESIAN_POINT ( 'NONE',  ( -53.51423613279429503, -127.5000000013656347, 4.591703134518082763 ) ) ;
#19292=CARTESIAN_POINT ( 'NONE',  ( -60.14911071818854538, -143.0625000000000284, 1.666127454062681146 ) ) ;
#19293=ORIENTED_EDGE ( 'NONE', *, *, #2696, .T. ) ;
#19296=CARTESIAN_POINT ( 'NONE',  ( -51.75738570946856498, -149.8750000027312126, 3.805975901505576964 ) ) ;
#19327=( NAMED_UNIT ( * ) PLANE_ANGLE_UNIT ( ) SI_UNIT ( $, .RADIAN. ) );
#19330=CARTESIAN_POINT ( 'NONE',  ( -51.75738570946856498, -149.7500000000000284, 3.805975901505576964 ) ) ;
#19340=CARTESIAN_POINT ( 'NONE',  ( -60.14911071818854538, -140.0625000000000000, 1.666127454062681146 ) ) ;
#19345=DIRECTION ( 'NONE',  ( 0.000000000000000000, 1.000000000000000000, 0.000000000000000000 ) ) ;
#19348=DIRECTION ( 'NONE',  ( -0.8660254037844387076, 0.000000000000000000, -0.4999999999999997780 ) ) ;
#19365=CARTESIAN_POINT ( 'NONE',  ( -59.44456063193725015, -139.8125000013656063, -0.3552334253322034230 ) ) ;
#19384=CARTESIAN_POINT ( 'NONE',  ( -56.48576386720575471, -143.7500000013656063, -4.591703134518078322 ) ) ;
#19399=PRODUCT ( 'coupler', 'coupler', '', ( #6032 ) ) ;
#19404=CARTESIAN_POINT ( 'NONE',  ( -57.46284108482265651, -143.9375000000000000, 4.819101127000238627 ) ) ;
#19406=EDGE_CURVE ( 'NONE', #56532, #58923, #48692, .T. ) ;
#19412=CARTESIAN_POINT ( 'NONE',  ( -50.55543936806279248, -143.3125000013656063, 0.3552334253322060320 ) ) ;
#19422=VERTEX_POINT ( 'NONE', #1432 ) ;
#19424=CARTESIAN_POINT ( 'NONE',  ( -58.80597590150559739, -141.0000000000000000, 3.242614290531460330 ) ) ;
#19426=CARTESIAN_POINT ( 'NONE',  ( -55.00000000000002132, -155.0000000000000284, 1.734723475976807094E-15 ) ) ;
#19429=CARTESIAN_POINT ( 'NONE',  ( -55.00000000000001421, -135.0000000000000284, -8.082903768654752241 ) ) ;
#19432=CARTESIAN_POINT ( 'NONE',  ( -51.75738570946856498, -145.8750000027312126, 3.805975901505576964 ) ) ;
#19448=CARTESIAN_POINT ( 'NONE',  ( -60.14911071818854538, -133.0625000000000284, 1.666127454062681368 ) ) ;
#19456=CARTESIAN_POINT ( 'NONE',  ( -56.66612745406278151, -149.3125000000000284, -5.149110718188523173 ) ) ;
#19459=CARTESIAN_POINT ( 'NONE',  ( -49.85088928181150436, -127.6875000027312126, -1.666127454062680702 ) ) ;
#19483=CARTESIAN_POINT ( 'NONE',  ( -56.48576386720575471, -129.7500000013656063, -4.591703134518078322 ) ) ;
#19484=CARTESIAN_POINT ( 'NONE',  ( -59.29741812935640155, -148.6250000013656063, -2.196230717870135685 ) ) ;
#19517=CARTESIAN_POINT ( 'NONE',  ( -57.19623071787017210, -151.6250000013656063, 4.297418129356382899 ) ) ;
#19527=CARTESIAN_POINT ( 'NONE',  ( -59.81910112700025905, -145.1875000000000000, -2.462841084822630311 ) ) ;
#19535=CARTESIAN_POINT ( 'NONE',  ( -59.59170313451810586, -147.7500000013656063, 1.485763867205729394 ) ) ;
#19537=CARTESIAN_POINT ( 'NONE',  ( -51.75738570946856498, -138.8750000027312126, 3.805975901505576964 ) ) ;
#19548=CARTESIAN_POINT ( 'NONE',  ( -56.66612745406273888, -153.3125000000000284, -5.149110718188518732 ) ) ;
#19549=CARTESIAN_POINT ( 'NONE',  ( -59.44456063193725015, -134.5625000013656063, -0.3552334253322034230 ) ) ;
#19565=CARTESIAN_POINT ( 'NONE',  ( -50.40829686548195099, -143.0000000013655779, -1.485763867205728284 ) ) ;
#19589=ADVANCED_FACE ( 'NONE', ( #31627 ), #49970, .F. ) ;
#19599=FACE_OUTER_BOUND ( 'NONE', #47407, .T. ) ;
#19606=CARTESIAN_POINT ( 'NONE',  ( -59.59170313451811296, -128.7500000013656063, 1.485763867205729394 ) ) ;
#19613=CARTESIAN_POINT ( 'NONE',  ( -59.98410592259440222, -143.1250000000000284, -0.3983568153799752487 ) ) ;
#19617=CARTESIAN_POINT ( 'NONE',  ( -53.33387254593733928, -150.9375000027311842, 5.149110718188519620 ) ) ;
#19635=CARTESIAN_POINT ( 'NONE',  ( -50.55543936806279248, -154.0625000013656347, 0.3552334253322060320 ) ) ;
#19670=ORIENTED_EDGE ( 'NONE', *, *, #12639, .F. ) ;
#19681=CARTESIAN_POINT ( 'NONE',  ( -50.40829686548195099, -138.2500000013656063, -1.485763867205728284 ) ) ;
#19691=CARTESIAN_POINT ( 'NONE',  ( -50.18089887299978358, -150.6875000000000000, 2.462841084822575688 ) ) ;
#19702=CARTESIAN_POINT ( 'NONE',  ( -57.19623071787017210, -142.3750000013656063, 4.297418129356382899 ) ) ;
#19726=CARTESIAN_POINT ( 'NONE',  ( -52.80376928212989185, -145.1250000013655779, -4.297418129356379346 ) ) ;
#19752=CARTESIAN_POINT ( 'NONE',  ( -56.66612745406251861, -135.3125000000000284, -5.149110718188501856 ) ) ;
#19768=CARTESIAN_POINT ( 'NONE',  ( -56.66612745406270335, -133.3125000000000284, -5.149110718188516067 ) ) ;
#19778=CARTESIAN_POINT ( 'NONE',  ( -56.66612745406270335, -126.4375000027312410, -5.149110718188516067 ) ) ;
#19780=CARTESIAN_POINT ( 'NONE',  ( -53.50031669685712643, -135.0000000000000000, 4.660752013197171806 ) ) ;
#19783=LINE ( 'NONE', #29739, #40720 ) ;
#19800=CARTESIAN_POINT ( 'NONE',  ( -50.70258187064364108, -125.1250000013656205, 2.196230717870141014 ) ) ;
#19801=CARTESIAN_POINT ( 'NONE',  ( -52.10840900171896806, -148.1875000013656063, 3.393966926194110556 ) ) ;
#19826=ORIENTED_EDGE ( 'NONE', *, *, #39005, .T. ) ;
#19833=CARTESIAN_POINT ( 'NONE',  ( -50.40829686548195099, -151.2500000013656063, -1.485763867205728284 ) ) ;
#19843=CARTESIAN_POINT ( 'NONE',  ( -59.98410592259440222, -146.1250000000000284, -0.3983568153799752487 ) ) ;
#19852=CARTESIAN_POINT ( 'NONE',  ( -56.48576386720575471, -148.0000000013656063, -4.591703134518078322 ) ) ;
#19853=CARTESIAN_POINT ( 'NONE',  ( -50.18089887299979068, -139.8125000027312126, 2.462841084822635640 ) ) ;
#19857=CARTESIAN_POINT ( 'NONE',  ( -58.80597590150559739, -135.0000000000000284, 3.242614290531460330 ) ) ;
#19866=CARTESIAN_POINT ( 'NONE',  ( -50.70258187064364108, -134.1250000013656347, 2.196230717870141014 ) ) ;
#19868=CARTESIAN_POINT ( 'NONE',  ( -51.75738570946856498, -145.8750000027312126, 3.805975901505576964 ) ) ;
#19877=CARTESIAN_POINT ( 'NONE',  ( -56.66612745406286678, -143.4375000027312410, -5.149110718188528502 ) ) ;
#19882=CARTESIAN_POINT ( 'NONE',  ( -54.64476657466781973, -138.8125000013656063, -4.444560631937228834 ) ) ;
#19912=CARTESIAN_POINT ( 'NONE',  ( -59.59170313451810586, -150.5000000013655779, 1.485763867205729394 ) ) ;
#19919=CARTESIAN_POINT ( 'NONE',  ( -52.80376928212989185, -128.1250000013656347, -4.297418129356379346 ) ) ;
#19923=CARTESIAN_POINT ( 'NONE',  ( -58.24261429053147765, -136.3750000027312126, -3.805975901505573855 ) ) ;
#19931=CARTESIAN_POINT ( 'NONE',  ( -49.85088928181150436, -148.6875000027311842, -1.666127454062680702 ) ) ;
#19934=ORIENTED_EDGE ( 'NONE', *, *, #62817, .T. ) ;
#19943=EDGE_LOOP ( 'NONE', ( #51812, #48328, #29909, #4622 ) ) ;
#19951=DIRECTION ( 'NONE',  ( -0.000000000000000000, -1.000000000000000000, 0.000000000000000000 ) ) ;
#19972=EDGE_CURVE ( 'NONE', #45194, #47814, #38962, .T. ) ;
#19974=CARTESIAN_POINT ( 'NONE',  ( -50.01589407740564042, -151.7500000027312410, 0.3983568153799778022 ) ) ;
#19978=CARTESIAN_POINT ( 'NONE',  ( -59.71086361768055184, -135.0000000000000000, -0.7912278194080049065 ) ) ;
#19989=VERTEX_POINT ( 'NONE', #34140 ) ;
#20001=CARTESIAN_POINT ( 'NONE',  ( -59.59170313451811296, -140.7500000013655779, 1.485763867205729394 ) ) ;
#20013=CARTESIAN_POINT ( 'NONE',  ( -51.75738570946856498, -142.8750000027312126, 3.805975901505576964 ) ) ;
#20017=AXIS2_PLACEMENT_3D ( 'NONE', #26658, #7683, #27289 ) ;
#20021=CARTESIAN_POINT ( 'NONE',  ( -50.70258187064364108, -139.1250000013656063, 2.196230717870141014 ) ) ;
#20048=CARTESIAN_POINT ( 'NONE',  ( -50.40829686548195099, -143.2500000013656063, -1.485763867205728284 ) ) ;
#20071=CARTESIAN_POINT ( 'NONE',  ( -57.46284108482265651, -150.9375000000000000, 4.819101127000238627 ) ) ;
#20087=CARTESIAN_POINT ( 'NONE',  ( -59.81910112700025905, -130.1875000000000568, -2.462841084822630311 ) ) ;
#20096=CARTESIAN_POINT ( 'NONE',  ( -59.29741812935640155, -151.6250000013656063, -2.196230717870135685 ) ) ;
#20101=CARTESIAN_POINT ( 'NONE',  ( -58.24261429053147765, -146.2500000000000284, -3.805975901505573855 ) ) ;
#20127=CARTESIAN_POINT ( 'NONE',  ( -50.55543936806279248, -154.3125000013656347, 0.3552334253322060320 ) ) ;
#20128=CARTESIAN_POINT ( 'NONE',  ( -58.39396692619412477, -148.4375000013656063, 2.891590998281057701 ) ) ;
#20136=EDGE_CURVE ( 'NONE', #32525, #39907, #12448, .T. ) ;
#20161=CARTESIAN_POINT ( 'NONE',  ( -52.80376928212989185, -146.1250000013656063, -4.297418129356379346 ) ) ;
#20171=CARTESIAN_POINT ( 'NONE',  ( -58.80597590150559739, -140.0000000000000284, 3.242614290531460330 ) ) ;
#20180=CARTESIAN_POINT ( 'NONE',  ( -58.39396692619412477, -144.6875000013656063, 2.891590998281057701 ) ) ;
#20182=CARTESIAN_POINT ( 'NONE',  ( -52.53715891517739323, -135.5625000027311842, -4.819101127000233298 ) ) ;
#20193=CARTESIAN_POINT ( 'NONE',  ( -52.10840900171896806, -132.1875000013656063, 3.393966926194110556 ) ) ;
#20195=CARTESIAN_POINT ( 'NONE',  ( -53.33387254593723270, -145.9375000027312410, 5.149110718188528502 ) ) ;
#20210=CARTESIAN_POINT ( 'NONE',  ( -50.55543936806279248, -137.0625000013656063, 0.3552334253322060320 ) ) ;
#20217=ADVANCED_FACE ( 'NONE', ( #31226 ), #46026, .F. ) ;
#20219=CARTESIAN_POINT ( 'NONE',  ( -57.89159099828107458, -133.9375000013656063, -3.393966926194107447 ) ) ;
#20243=CARTESIAN_POINT ( 'NONE',  ( -51.60603307380591787, -150.9375000013656063, -2.891590998281053704 ) ) ;
#20249=FACE_OUTER_BOUND ( 'NONE', #25996, .T. ) ;
#20250=CARTESIAN_POINT ( 'NONE',  ( -59.59170313451811296, -126.7500000013655921, 1.485763867205729394 ) ) ;
#20256=CARTESIAN_POINT ( 'NONE',  ( -50.18089887299976937, -136.8125000027311842, 2.462841084822337656 ) ) ;
#20263=CARTESIAN_POINT ( 'NONE',  ( -58.24261429053147765, -150.3750000027312126, -3.805975901505573855 ) ) ;
#20279=CARTESIAN_POINT ( 'NONE',  ( -51.75738570946856498, -143.7500000000000284, 3.805975901505576964 ) ) ;
#20281=CARTESIAN_POINT ( 'NONE',  ( -59.44456063193725015, -149.5625000013656063, -0.3552334253322034230 ) ) ;
#20283=CARTESIAN_POINT ( 'NONE',  ( -49.85088928181150436, -148.5625000000000000, -1.666127454062680480 ) ) ;
#20289=ORIENTED_EDGE ( 'NONE', *, *, #8713, .T. ) ;
#20301=CARTESIAN_POINT ( 'NONE',  ( -51.19402409849444524, -151.6250000027312126, -3.242614290531456334 ) ) ;
#20327=EDGE_CURVE ( 'NONE', #12526, #52748, #37326, .T. ) ;
#20328=CARTESIAN_POINT ( 'NONE',  ( -58.39396692619412477, -138.6875000013656347, 2.891590998281057701 ) ) ;
#20335=CARTESIAN_POINT ( 'NONE',  ( -50.96713099277813797, -135.0000000000000568, -1.923792341520001115 ) ) ;
#20338=DIRECTION ( 'NONE',  ( 0.000000000000000000, 1.000000000000000000, 0.000000000000000000 ) ) ;
#20347=CARTESIAN_POINT ( 'NONE',  ( -50.55543936806279248, -142.0625000013656063, 0.3552334253322060320 ) ) ;
#20375=CARTESIAN_POINT ( 'NONE',  ( -53.51423613279429503, -144.5000000013656063, 4.591703134518082763 ) ) ;
#20389=CARTESIAN_POINT ( 'NONE',  ( -58.24261429053147765, -138.3750000027312126, -3.805975901505573855 ) ) ;
#20399=CARTESIAN_POINT ( 'NONE',  ( -58.24261429053147765, -151.2500000000000284, -3.805975901505573855 ) ) ;
#20407=CARTESIAN_POINT ( 'NONE',  ( -51.75738570946856498, -137.7500000000000000, 3.805975901505576964 ) ) ;
#20416=CARTESIAN_POINT ( 'NONE',  ( -50.18089887299979068, -129.6875000000000568, 2.462841084822635640 ) ) ;
#20424=CARTESIAN_POINT ( 'NONE',  ( -52.80376928212989185, -152.8750000013656063, -4.297418129356379346 ) ) ;
#20450=CARTESIAN_POINT ( 'NONE',  ( -54.64476657466781973, -126.8125000013655921, -4.444560631937228834 ) ) ;
#20452=CARTESIAN_POINT ( 'NONE',  ( -54.64476657466781973, -141.8125000013656063, -4.444560631937228834 ) ) ;
#20465=DIRECTION ( 'NONE',  ( 0.000000000000000000, 1.000000000000000000, 0.000000000000000000 ) ) ;
#20481=ADVANCED_FACE ( 'NONE', ( #18338 ), #22226, .F. ) ;
#20495=CARTESIAN_POINT ( 'NONE',  ( -50.01589407740564042, -142.6250000000000284, 0.3983568153799778022 ) ) ;
#20505=CARTESIAN_POINT ( 'NONE',  ( -59.29741812935640155, -145.8750000013655779, -2.196230717870135685 ) ) ;
#20507=CARTESIAN_POINT ( 'NONE',  ( -59.81910112700025905, -133.3125000027312410, -2.462841084822630311 ) ) ;
#20521=CARTESIAN_POINT ( 'NONE',  ( -50.55543936806279248, -129.0625000013656063, 0.3552334253322060320 ) ) ;
#20538=CARTESIAN_POINT ( 'NONE',  ( -50.70258187064364108, -139.1250000013656063, 2.196230717870141014 ) ) ;
#20547=CARTESIAN_POINT ( 'NONE',  ( -55.35523342533222291, -132.5625000013656063, 4.444560631937231499 ) ) ;
#20564=ADVANCED_FACE ( 'NONE', ( #49951 ), #21015, .F. ) ;
#20572=CARTESIAN_POINT ( 'NONE',  ( -56.48576386720575471, -149.7500000013656063, -4.591703134518078322 ) ) ;
#20580=CARTESIAN_POINT ( 'NONE',  ( -50.18089887299979068, -152.6875000000000284, 2.462841084822635640 ) ) ;
#20589=CARTESIAN_POINT ( 'NONE',  ( -55.00000000000002132, -155.0000000000000284, 1.734723475976807094E-15 ) ) ;
#20591=CARTESIAN_POINT ( 'NONE',  ( -50.01589407740564042, -145.7500000027312126, 0.3983568153799778022 ) ) ;
#20594=ORIENTED_EDGE ( 'NONE', *, *, #12639, .T. ) ;
#20609=CARTESIAN_POINT ( 'NONE',  ( -53.33387254593703375, -137.8124999999999716, 5.149110718188541824 ) ) ;
#20610=CARTESIAN_POINT ( 'NONE',  ( -53.51423613279429503, -148.2500000013656063, 4.591703134518082763 ) ) ;
#20614=CYLINDRICAL_SURFACE ( 'NONE', #1778, 5.000000000000000000 ) ;
#20618=( GEOMETRIC_REPRESENTATION_CONTEXT ( 3 ) GLOBAL_UNCERTAINTY_ASSIGNED_CONTEXT ( ( #28519 ) ) GLOBAL_UNIT_ASSIGNED_CONTEXT ( ( #41093, #19327, #53740 ) ) REPRESENTATION_CONTEXT ( 'NONE', 'WORKASPACE' ) );
#20658=CARTESIAN_POINT ( 'NONE',  ( -55.35523342533222291, -135.5625000013656063, 4.444560631937231499 ) ) ;
#20675=CARTESIAN_POINT ( 'NONE',  ( -52.80376928212989185, -141.8750000013655779, -4.297418129356379346 ) ) ;
#20683=CARTESIAN_POINT ( 'NONE',  ( -49.85088928181150436, -147.5625000000000000, -1.666127454062680480 ) ) ;
#20702=CARTESIAN_POINT ( 'NONE',  ( -52.80376928212989185, -143.1250000013656063, -4.297418129356379346 ) ) ;
#20738=CARTESIAN_POINT ( 'NONE',  ( -52.53715891517739323, -130.4375000000000284, -4.819101127000233298 ) ) ;
#20745=CARTESIAN_POINT ( 'NONE',  ( -58.24261429053147765, -124.3750000027312126, -3.805975901505573855 ) ) ;
#20770=CARTESIAN_POINT ( 'NONE',  ( -52.10840900171896806, -126.1875000013656063, 3.393966926194110556 ) ) ;
#20771=CARTESIAN_POINT ( 'NONE',  ( -52.10840900171896806, -141.1875000013656063, 3.393966926194110556 ) ) ;
#20809=ORIENTED_EDGE ( 'NONE', *, *, #49475, .F. ) ;
#20810=CARTESIAN_POINT ( 'NONE',  ( -55.39835681537999790, -139.8750000000000284, 4.984105922594378235 ) ) ;
#20822=CARTESIAN_POINT ( 'NONE',  ( -59.29741812935640155, -146.8750000013656063, -2.196230717870135685 ) ) ;
#20824=CARTESIAN_POINT ( 'NONE',  ( -54.60164318462004474, -135.5000000027312126, -4.984105922594373794 ) ) ;
#20837=CARTESIAN_POINT ( 'NONE',  ( -59.59170313451811296, -130.5000000013656063, 1.485763867205729394 ) ) ;
#20852=CARTESIAN_POINT ( 'NONE',  ( -59.44456063193725015, -137.5625000013656063, -0.3552334253322034230 ) ) ;
#20863=CARTESIAN_POINT ( 'NONE',  ( -50.55543936806279248, -131.3125000013656063, 0.3552334253322060320 ) ) ;
#20887=CARTESIAN_POINT ( 'NONE',  ( -50.55543936806279248, -149.0625000013656063, 0.3552334253322060320 ) ) ;
#20895=CARTESIAN_POINT ( 'NONE',  ( -57.89159099828107458, -124.9375000013656063, -3.393966926194107447 ) ) ;
#20905=CARTESIAN_POINT ( 'NONE',  ( -58.24261429053147765, -148.3750000027312126, -3.805975901505573855 ) ) ;
#20923=CARTESIAN_POINT ( 'NONE',  ( -52.80376928212989185, -150.8750000013656063, -4.297418129356379346 ) ) ;
#20943=CARTESIAN_POINT ( 'NONE',  ( -58.24261429053147765, -153.3750000027312126, -3.805975901505573855 ) ) ;
#20950=EDGE_CURVE ( 'NONE', #24283, #46979, #9679, .T. ) ;
#20973=CARTESIAN_POINT ( 'NONE',  ( -52.10840900171896806, -133.4375000013656063, 3.393966926194110556 ) ) ;
#20979=CARTESIAN_POINT ( 'NONE',  ( -54.06206593695552698, -135.0000000000000284, -4.368617065816306599 ) ) ;
#20989=CARTESIAN_POINT ( 'NONE',  ( -50.70258187064364108, -142.1250000013656063, 2.196230717870141014 ) ) ;
#20996=CARTESIAN_POINT ( 'NONE',  ( -51.75738570946856498, -147.7500000000000284, 3.805975901505576964 ) ) ;
#21013=CARTESIAN_POINT ( 'NONE',  ( -53.51423613279429503, -141.5000000013656063, 4.591703134518082763 ) ) ;
#21014=( BOUNDED_CURVE ( )  B_SPLINE_CURVE ( 2, ( #15134, #44711, #674, #20283, #15463, #45682, #41800, #17372, #16733 ),
 .UNSPECIFIED., .F., .F. ) 
 B_SPLINE_CURVE_WITH_KNOTS ( ( 3, 2, 2, 2, 3 ),
 ( 0.2083333333333335091, 0.2125000000000001610, 0.2166666666666668406, 0.2208333333333335202, 0.2250000000000001998 ),
 .UNSPECIFIED. ) 
 CURVE ( )  GEOMETRIC_REPRESENTATION_ITEM ( )  RATIONAL_B_SPLINE_CURVE ( ( 0.9999999999999970024, 0.9238795325112897361, 1.000000000000000000, 0.9238795325112867385, 1.000000000000000000, 0.9238795325112867385, 1.000000000000000000, 0.9238795325112831858, 1.000000000000003553 ) ) 
 REPRESENTATION_ITEM ( '' )  );
#21015=CYLINDRICAL_SURFACE ( 'NONE', #37017, 5.000000000000000000 ) ;
#21048=CARTESIAN_POINT ( 'NONE',  ( -50.18089887299976937, -137.6875000000000284, 2.462841084822337656 ) ) ;
#21054=CARTESIAN_POINT ( 'NONE',  ( -56.66612745406270335, -129.3125000000000284, -5.149110718188516067 ) ) ;
#21057=ORIENTED_EDGE ( 'NONE', *, *, #19406, .T. ) ;
#21062=CARTESIAN_POINT ( 'NONE',  ( -55.35523342533222291, -152.3125000013656063, 4.444560631937231499 ) ) ;
#21074=CARTESIAN_POINT ( 'NONE',  ( -59.81910112700026616, -147.1874999999999716, -2.462841084822510851 ) ) ;
#21076=CARTESIAN_POINT ( 'NONE',  ( -58.80597590150559739, -154.5625000013656347, 3.242614290531460330 ) ) ;
#21087=CARTESIAN_POINT ( 'NONE',  ( -51.60603307380591787, -124.9375000013656063, -2.891590998281053704 ) ) ;
#21088=CARTESIAN_POINT ( 'NONE',  ( -57.89159099828107458, -142.6875000013656063, -3.393966926194107447 ) ) ;
#21124=CARTESIAN_POINT ( 'NONE',  ( -49.85088928181150436, -143.5625000000000568, -1.666127454062680702 ) ) ;
#21128=VERTEX_POINT ( 'NONE', #9059 ) ;
#21135=CARTESIAN_POINT ( 'NONE',  ( -59.59170313451810586, -140.7500000013655779, 1.485763867205729394 ) ) ;
#21137=CARTESIAN_POINT ( 'NONE',  ( -58.24261429053147765, -135.3750000027312410, -3.805975901505573855 ) ) ;
#21151=CARTESIAN_POINT ( 'NONE',  ( -58.39396692619412477, -129.4375000013656063, 2.891590998281057701 ) ) ;
#21164=CARTESIAN_POINT ( 'NONE',  ( -54.64476657466781973, -136.8125000013656063, -4.444560631937228834 ) ) ;
#21173=CARTESIAN_POINT ( 'NONE',  ( -55.35523342533222291, -131.5625000013656063, 4.444560631937231499 ) ) ;
#21182=CARTESIAN_POINT ( 'NONE',  ( -51.75738570946856498, -151.7500000000000284, 3.805975901505576964 ) ) ;
#21205=CARTESIAN_POINT ( 'NONE',  ( -55.39835681537999790, -153.8750000000000284, 4.984105922594378235 ) ) ;
#21214=CARTESIAN_POINT ( 'NONE',  ( -56.48576386720575471, -154.0000000013656063, -4.591703134518078322 ) ) ;
#21216=CARTESIAN_POINT ( 'NONE',  ( -56.66612745406270335, -147.4375000027311842, -5.149110718188516067 ) ) ;
#21217=CIRCLE ( 'NONE', #1717, 5.000000000000000000 ) ;
#21225=ADVANCED_FACE ( 'NONE', ( #38020 ), #34123, .F. ) ;
#21237=CARTESIAN_POINT ( 'NONE',  ( -57.19623071787017210, -149.3750000013656347, 4.297418129356382899 ) ) ;
#21239=LINE ( 'NONE', #22201, #61991 ) ;
#21272=AXIS2_PLACEMENT_3D ( 'NONE', #30560, #6137, #49548 ) ;
#21282=CARTESIAN_POINT ( 'NONE',  ( -50.70258187064364108, -133.3750000013656063, 2.196230717870141014 ) ) ;
#21316=AXIS2_PLACEMENT_3D ( 'NONE', #24870, #58645, #28424 ) ;
#21331=CARTESIAN_POINT ( 'NONE',  ( -55.35523342533222291, -138.5625000013656063, 4.444560631937231499 ) ) ;
#21349=CARTESIAN_POINT ( 'NONE',  ( -54.64476657466781973, -136.0625000013656063, -4.444560631937228834 ) ) ;
#21363=CARTESIAN_POINT ( 'NONE',  ( -57.19623071787017210, -148.6250000013656063, 4.297418129356382899 ) ) ;
#21373=CARTESIAN_POINT ( 'NONE',  ( -59.98410592259440222, -130.1250000000000284, -0.3983568153799752487 ) ) ;
#21381=CARTESIAN_POINT ( 'NONE',  ( -57.89159099828107458, -152.6875000013656063, -3.393966926194107447 ) ) ;
#21409=CARTESIAN_POINT ( 'NONE',  ( -59.29741812935640155, -150.8750000013656063, -2.196230717870135685 ) ) ;
#21410=CARTESIAN_POINT ( 'NONE',  ( -53.51423613279429503, -141.2500000013656063, 4.591703134518083651 ) ) ;
#21422=CARTESIAN_POINT ( 'NONE',  ( -59.81910112700024484, -136.1875000000000284, -2.462841084822808835 ) ) ;
#21449=CARTESIAN_POINT ( 'NONE',  ( -51.19402409849444524, -141.5000000000000284, -3.242614290531456334 ) ) ;
#21457=EDGE_LOOP ( 'NONE', ( #30693, #24022, #11883, #31068 ) ) ;
#21459=CARTESIAN_POINT ( 'NONE',  ( -55.35523342533222291, -142.5625000013656063, 4.444560631937231499 ) ) ;
#21461=CARTESIAN_POINT ( 'NONE',  ( -58.80597590150559739, -135.1250000027312410, 3.242614290531460330 ) ) ;
#21473=CARTESIAN_POINT ( 'NONE',  ( -57.89159099828107458, -130.6875000013656063, -3.393966926194107447 ) ) ;
#21476=CARTESIAN_POINT ( 'NONE',  ( -58.80597590150559739, -142.1250000027312126, 3.242614290531460330 ) ) ;
#21488=CARTESIAN_POINT ( 'NONE',  ( -59.59170313451811296, -133.5000000013656347, 1.485763867205729394 ) ) ;
#21500=CARTESIAN_POINT ( 'NONE',  ( -51.60603307380591787, -133.1875000013656063, -2.891590998281053704 ) ) ;
#21526=CARTESIAN_POINT ( 'NONE',  ( -51.60603307380591787, -139.9375000013656063, -2.891590998281053704 ) ) ;
#21532=CARTESIAN_POINT ( 'NONE',  ( -56.66612745406270335, -153.3125000000000000, -5.149110718188516067 ) ) ;
#21536=SHAPE_REPRESENTATION_RELATIONSHIP ( 'NONE' , 'NONE' ,  #49651, #60912 ) ;
#21543=CARTESIAN_POINT ( 'NONE',  ( -53.33387254593733928, -144.9375000027312126, 5.149110718188519620 ) ) ;
#21561=CARTESIAN_POINT ( 'NONE',  ( -58.24261429053147765, -138.2500000000000000, -3.805975901505573855 ) ) ;
#21562=CARTESIAN_POINT ( 'NONE',  ( -59.44456063193725015, -148.5625000013656063, -0.3552334253322034230 ) ) ;
#21584=ORIENTED_EDGE ( 'NONE', *, *, #32699, .F. ) ;
#21589=VECTOR ( 'NONE', #28208, 1000.000000000000000 ) ;
#21608=CARTESIAN_POINT ( 'NONE',  ( -59.29741812935640155, -135.8750000013655779, -2.196230717870135685 ) ) ;
#21609=EDGE_CURVE ( 'NONE', #42590, #2645, #48138, .T. ) ;
#21630=CYLINDRICAL_SURFACE ( 'NONE', #14214, 5.000000000000000000 ) ;
#21652=CARTESIAN_POINT ( 'NONE',  ( -57.19623071787017210, -140.6250000013656063, 4.297418129356382899 ) ) ;
#21687=CARTESIAN_POINT ( 'NONE',  ( -53.51423613279429503, -146.5000000013656347, 4.591703134518082763 ) ) ;
#21699=CARTESIAN_POINT ( 'NONE',  ( -54.60164318462004474, -126.3750000000000142, -4.984105922594373794 ) ) ;
#21706=CARTESIAN_POINT ( 'NONE',  ( -54.64476657466781973, -149.8125000013656063, -4.444560631937228834 ) ) ;
#21729=CARTESIAN_POINT ( 'NONE',  ( -51.60603307380591787, -151.1875000013656063, -2.891590998281053704 ) ) ;
#21730=CARTESIAN_POINT ( 'NONE',  ( -51.60603307380591787, -141.9375000013656063, -2.891590998281053704 ) ) ;
#21754=EDGE_CURVE ( 'NONE', #26446, #41301, #25281, .T. ) ;
#21771=CARTESIAN_POINT ( 'NONE',  ( -53.33387254593733928, -137.8125000000000000, 5.149110718188519620 ) ) ;
#21781=CARTESIAN_POINT ( 'NONE',  ( -54.64476657466781973, -144.0625000013656063, -4.444560631937228834 ) ) ;
#21783=CARTESIAN_POINT ( 'NONE',  ( -60.14911071818854538, -130.1875000027312410, 1.666127454062681368 ) ) ;
#21794=CARTESIAN_POINT ( 'NONE',  ( -52.10840900171896806, -129.1875000013656063, 3.393966926194110556 ) ) ;
#21806=CYLINDRICAL_SURFACE ( 'NONE', #19179, 5.000000000000000000 ) ;
#21807=CARTESIAN_POINT ( 'NONE',  ( -50.40829686548195099, -134.0000000013656063, -1.485763867205728284 ) ) ;
#21814=ORIENTED_EDGE ( 'NONE', *, *, #44439, .F. ) ;
#21816=CARTESIAN_POINT ( 'NONE',  ( -51.60603307380591787, -129.1875000013656063, -2.891590998281053704 ) ) ;
#21824=( BOUNDED_CURVE ( )  B_SPLINE_CURVE ( 2, ( #8695, #48866, #4811, #23175, #44036, #37973, #63367, #28307, #42786 ),
 .UNSPECIFIED., .F., .F. ) 
 B_SPLINE_CURVE_WITH_KNOTS ( ( 3, 2, 2, 2, 3 ),
 ( 0.1416666666666667740, 0.1458333333333334814, 0.1500000000000001332, 0.1541666666666668406, 0.1583333333333334925 ),
 .UNSPECIFIED. ) 
 CURVE ( )  GEOMETRIC_REPRESENTATION_ITEM ( )  RATIONAL_B_SPLINE_CURVE ( ( 0.9999999999999980016, 0.9238795325112887369, 1.000000000000000000, 0.9238795325112867385, 1.000000000000000000, 0.9238795325112867385, 1.000000000000000000, 0.9238795325112837409, 1.000000000000003109 ) ) 
 REPRESENTATION_ITEM ( '' )  );
#21825=DIRECTION ( 'NONE',  ( -0.8660254037844384856, 0.000000000000000000, 0.5000000000000001110 ) ) ;
#21843=CARTESIAN_POINT ( 'NONE',  ( -52.80376928212989185, -137.8750000013655779, -4.297418129356378458 ) ) ;
#21848=CARTESIAN_POINT ( 'NONE',  ( -52.53715891517739323, -152.4375000000000284, -4.819101127000233298 ) ) ;
#21852=( NAMED_UNIT ( * ) SI_UNIT ( $, .STERADIAN. ) SOLID_ANGLE_UNIT ( ) );
#21857=CARTESIAN_POINT ( 'NONE',  ( -52.10840900171896806, -154.4375000013656063, 3.393966926194110556 ) ) ;
#21859=CARTESIAN_POINT ( 'NONE',  ( -50.18089887299979068, -141.8125000027311842, 2.462841084822635640 ) ) ;
#21879=CARTESIAN_POINT ( 'NONE',  ( -59.29741812935640155, -147.6250000013655779, -2.196230717870135685 ) ) ;
#21911=EDGE_LOOP ( 'NONE', ( #23341, #29167, #21057, #62524 ) ) ;
#21920=CARTESIAN_POINT ( 'NONE',  ( -52.10840900171896806, -135.4375000013656063, 3.393966926194110556 ) ) ;
#21940=DIRECTION ( 'NONE',  ( 0.000000000000000000, 1.000000000000000000, 0.000000000000000000 ) ) ;
#21946=( BOUNDED_CURVE ( )  B_SPLINE_CURVE ( 2, ( #9400, #29009, #58618, #34158, #33851, #32916, #8164, #19050, #8473 ),
 .UNSPECIFIED., .F., .F. ) 
 B_SPLINE_CURVE_WITH_KNOTS ( ( 3, 2, 2, 2, 3 ),
 ( 0.1916666666666668462, 0.1958333333333334980, 0.2000000000000001776, 0.2041666666666668295, 0.2083333333333335091 ),
 .UNSPECIFIED. ) 
 CURVE ( )  GEOMETRIC_REPRESENTATION_ITEM ( )  RATIONAL_B_SPLINE_CURVE ( ( 0.9999999999999970024, 0.9238795325112897361, 1.000000000000000000, 0.9238795325112867385, 1.000000000000000000, 0.9238795325112867385, 1.000000000000000000, 0.9238795325112837409, 1.000000000000003109 ) ) 
 REPRESENTATION_ITEM ( '' )  );
#21949=EDGE_CURVE ( 'NONE', #17633, #4656, #24017, .T. ) ;
#21952=FACE_OUTER_BOUND ( 'NONE', #18201, .T. ) ;
#21964=CARTESIAN_POINT ( 'NONE',  ( -56.48576386720575471, -140.0000000013656063, -4.591703134518078322 ) ) ;
#21965=VECTOR ( 'NONE', #4277, 1000.000000000000000 ) ;
#21973=CARTESIAN_POINT ( 'NONE',  ( -51.75738570946856498, -146.7500000000000284, 3.805975901505576964 ) ) ;
#21976=ORIENTED_EDGE ( 'NONE', *, *, #20136, .F. ) ;
#21985=CARTESIAN_POINT ( 'NONE',  ( -59.29741812935640155, -136.8750000013656063, -2.196230717870135685 ) ) ;
#21997=CARTESIAN_POINT ( 'NONE',  ( -57.89159099828107458, -147.9375000013656063, -3.393966926194107447 ) ) ;
#22016=CARTESIAN_POINT ( 'NONE',  ( -51.60603307380591787, -147.9375000013656063, -2.891590998281053704 ) ) ;
#22041=CARTESIAN_POINT ( 'NONE',  ( -56.48576386720575471, -153.0000000013656063, -4.591703134518078322 ) ) ;
#22056=CARTESIAN_POINT ( 'NONE',  ( -55.39835681537999790, -135.8750000000000284, 4.984105922594378235 ) ) ;
#22079=CARTESIAN_POINT ( 'NONE',  ( -55.39835681537999790, -137.8750000000000284, 4.984105922594378235 ) ) ;
#22082=ORIENTED_EDGE ( 'NONE', *, *, #48092, .T. ) ;
#22090=CARTESIAN_POINT ( 'NONE',  ( -56.48576386720575471, -141.0000000013655779, -4.591703134518078322 ) ) ;
#22092=CARTESIAN_POINT ( 'NONE',  ( -60.14911071818854538, -132.1875000027312410, 1.666127454062681368 ) ) ;
#22109=CARTESIAN_POINT ( 'NONE',  ( -58.39396692619412477, -124.4375000013656063, 2.891590998281057701 ) ) ;
#22122=CARTESIAN_POINT ( 'NONE',  ( -50.70258187064364108, -134.1250000013656347, 2.196230717870141014 ) ) ;
#22131=CARTESIAN_POINT ( 'NONE',  ( -54.64476657466781973, -128.0625000013656063, -4.444560631937228834 ) ) ;
#22134=( BOUNDED_CURVE ( )  B_SPLINE_CURVE ( 2, ( #15286, #44869, #49695, #40036, #23530, #52796, #32538, #33181, #8731 ),
 .UNSPECIFIED., .F., .F. ) 
 B_SPLINE_CURVE_WITH_KNOTS ( ( 3, 2, 2, 2, 3 ),
 ( 0.3250000000000002887, 0.3291666666666669405, 0.3333333333333335924, 0.3375000000000002998, 0.3416666666666669516 ),
 .UNSPECIFIED. ) 
 CURVE ( )  GEOMETRIC_REPRESENTATION_ITEM ( )  RATIONAL_B_SPLINE_CURVE ( ( 0.9999999999999948930, 0.9238795325112918455, 1.000000000000000000, 0.9238795325112867385, 1.000000000000000000, 0.9238795325112867385, 1.000000000000000000, 0.9238795325112816315, 1.000000000000005107 ) ) 
 REPRESENTATION_ITEM ( '' )  );
#22155=CARTESIAN_POINT ( 'NONE',  ( -58.39396692619412477, -154.6875000013656063, 2.891590998281057701 ) ) ;
#22159=CARTESIAN_POINT ( 'NONE',  ( -58.39396692619412477, -137.4375000013656063, 2.891590998281057701 ) ) ;
#22164=CARTESIAN_POINT ( 'NONE',  ( -53.33387254593733928, -148.8125000000000284, 5.149110718188519620 ) ) ;
#22172=CARTESIAN_POINT ( 'NONE',  ( -57.89159099828107458, -153.9375000013656063, -3.393966926194107447 ) ) ;
#22173=CARTESIAN_POINT ( 'NONE',  ( -51.75738570946856498, -143.8750000027312126, 3.805975901505576964 ) ) ;
#22180=CARTESIAN_POINT ( 'NONE',  ( -59.44456063193725015, -138.5625000013656063, -0.3552334253322034230 ) ) ;
#22197=VECTOR ( 'NONE', #6631, 1000.000000000000000 ) ;
#22198=CARTESIAN_POINT ( 'NONE',  ( -59.59170313451811296, -147.5000000013656063, 1.485763867205729394 ) ) ;
#22201=CARTESIAN_POINT ( 'NONE',  ( -48.00000000000002132, -155.0000000000000284, -4.041451884327376121 ) ) ;
#22226=CYLINDRICAL_SURFACE ( 'NONE', #46286, 5.000000000000000000 ) ;
#22241=CARTESIAN_POINT ( 'NONE',  ( -54.64476657466781973, -130.0625000013656063, -4.444560631937228834 ) ) ;
#22285=CARTESIAN_POINT ( 'NONE',  ( -50.70258187064364108, -139.3750000013656063, 2.196230717870141014 ) ) ;
#22304=CARTESIAN_POINT ( 'NONE',  ( -59.29741812935640155, -135.8750000013655779, -2.196230717870135685 ) ) ;
#22316=CARTESIAN_POINT ( 'NONE',  ( -59.29741812935640155, -146.8750000013656063, -2.196230717870135685 ) ) ;
#22329=CARTESIAN_POINT ( 'NONE',  ( -52.53715891517739323, -126.4375000000000426, -4.819101127000233298 ) ) ;
#22340=CARTESIAN_POINT ( 'NONE',  ( -52.80376928212989185, -147.8750000013656063, -4.297418129356379346 ) ) ;
#22363=CARTESIAN_POINT ( 'NONE',  ( -59.29741812935640155, -153.8750000013655779, -2.196230717870135685 ) ) ;
#22404=CARTESIAN_POINT ( 'NONE',  ( -60.14911071818854538, -136.0625000000000284, 1.666127454062681368 ) ) ;
#22413=CARTESIAN_POINT ( 'NONE',  ( -52.10840900171896806, -143.4375000013656063, 3.393966926194110556 ) ) ;
#22415=CARTESIAN_POINT ( 'NONE',  ( -56.66612745406270335, -130.4375000027312410, -5.149110718188516067 ) ) ;
#22427=EDGE_CURVE ( 'NONE', #32079, #24403, #36686, .T. ) ;
#22442=CARTESIAN_POINT ( 'NONE',  ( -54.64476657466781973, -134.8125000013656063, -4.444560631937228834 ) ) ;
#22451=CARTESIAN_POINT ( 'NONE',  ( -50.40829686548195099, -126.2500000013656063, -1.485763867205728284 ) ) ;
#22482=CARTESIAN_POINT ( 'NONE',  ( -51.60603307380591787, -137.9375000013656063, -2.891590998281053704 ) ) ;
#22487=CARTESIAN_POINT ( 'NONE',  ( -58.80597590150559739, -151.0000000000000284, 3.242614290531460330 ) ) ;
#22495=CARTESIAN_POINT ( 'NONE',  ( -52.80376928212989185, -153.1250000013656063, -4.297418129356378458 ) ) ;
#22496=CARTESIAN_POINT ( 'NONE',  ( -59.98410592259440222, -143.2500000027312126, -0.3983568153799752487 ) ) ;
#22503=CARTESIAN_POINT ( 'NONE',  ( -51.60603307380591787, -136.9375000013655779, -2.891590998281053704 ) ) ;
#22521=CARTESIAN_POINT ( 'NONE',  ( -55.35523342533222291, -146.3125000013656063, 4.444560631937231499 ) ) ;
#22562=EDGE_CURVE ( 'NONE', #16286, #38301, #25206, .T. ) ;
#22565=CARTESIAN_POINT ( 'NONE',  ( -59.29741812935640155, -131.8750000013656347, -2.196230717870135685 ) ) ;
#22609=CARTESIAN_POINT ( 'NONE',  ( -50.40829686548195099, -136.2500000013656063, -1.485763867205728284 ) ) ;
#22618=EDGE_LOOP ( 'NONE', ( #18714, #40485, #33806, #59419 ) ) ;
#22622=CARTESIAN_POINT ( 'NONE',  ( -58.24261429053147765, -155.0000000000000284, -3.805975901505573411 ) ) ;
#22639=CARTESIAN_POINT ( 'NONE',  ( -59.59170313451811296, -142.7500000013656063, 1.485763867205729394 ) ) ;
#22642=ORIENTED_EDGE ( 'NONE', *, *, #56295, .F. ) ;
#22651=CARTESIAN_POINT ( 'NONE',  ( -59.81910112700025905, -127.1875000000000426, -2.462841084822630311 ) ) ;
#22659=CARTESIAN_POINT ( 'NONE',  ( -59.44456063193725015, -148.5625000013656063, -0.3552334253322034230 ) ) ;
#22683=CARTESIAN_POINT ( 'NONE',  ( -51.60603307380591787, -150.1875000013656063, -2.891590998281053704 ) ) ;
#22695=CARTESIAN_POINT ( 'NONE',  ( -53.33387254593731086, -152.8125000000000284, 5.149110718188520508 ) ) ;
#22721=CARTESIAN_POINT ( 'NONE',  ( -50.18089887299979068, -137.6875000000000000, 2.462841084822635640 ) ) ;
#22730=CARTESIAN_POINT ( 'NONE',  ( -50.40829686548195099, -140.2500000013656063, -1.485763867205728284 ) ) ;
#22732=CARTESIAN_POINT ( 'NONE',  ( -54.60164318462004474, -130.5000000027312126, -4.984105922594373794 ) ) ;
#22746=CARTESIAN_POINT ( 'NONE',  ( -59.29741812935640155, -124.6250000013656347, -2.196230717870135685 ) ) ;
#22750=ORIENTED_EDGE ( 'NONE', *, *, #27921, .T. ) ;
#22756=FACE_OUTER_BOUND ( 'NONE', #34708, .T. ) ;
#22757=CARTESIAN_POINT ( 'NONE',  ( -50.40829686548195099, -133.0000000013656063, -1.485763867205728284 ) ) ;
#22767=ORIENTED_EDGE ( 'NONE', *, *, #13810, .T. ) ;
#22769=CARTESIAN_POINT ( 'NONE',  ( -59.44456063193725015, -127.8125000013655921, -0.3552334253322034230 ) ) ;
#22783=CARTESIAN_POINT ( 'NONE',  ( -59.98410592259440222, -139.2500000027312126, -0.3983568153799752487 ) ) ;
#22797=CARTESIAN_POINT ( 'NONE',  ( -50.70258187064364108, -138.1250000013656063, 2.196230717870141014 ) ) ;
#22802=CARTESIAN_POINT ( 'NONE',  ( -59.98410592259440222, -150.1250000000000284, -0.3983568153799752487 ) ) ;
#22811=CARTESIAN_POINT ( 'NONE',  ( -56.48576386720575471, -151.0000000013656063, -4.591703134518078322 ) ) ;
#22812=CARTESIAN_POINT ( 'NONE',  ( -54.60164318462004474, -143.5000000027312126, -4.984105922594373794 ) ) ;
#22819=EDGE_CURVE ( 'NONE', #9785, #28712, #4252, .T. ) ;
#22823=CARTESIAN_POINT ( 'NONE',  ( -59.59170313451811296, -138.5000000013656347, 1.485763867205729394 ) ) ;
#22838=CARTESIAN_POINT ( 'NONE',  ( -50.70258187064364108, -145.1250000013655779, 2.196230717870141014 ) ) ;
#22842=CARTESIAN_POINT ( 'NONE',  ( -51.19402409849444524, -141.6250000027312126, -3.242614290531456334 ) ) ;
#22851=CARTESIAN_POINT ( 'NONE',  ( -57.46284108482265651, -148.9375000000000000, 4.819101127000238627 ) ) ;
#22878=CARTESIAN_POINT ( 'NONE',  ( -56.48576386720575471, -130.0000000013656063, -4.591703134518078322 ) ) ;
#22881=DIRECTION ( 'NONE',  ( 0.000000000000000000, 1.000000000000000000, 0.000000000000000000 ) ) ;
#22896=EDGE_CURVE ( 'NONE', #6296, #34224, #63428, .T. ) ;
#22897=CARTESIAN_POINT ( 'NONE',  ( -51.75738570946856498, -150.8750000027312126, 3.805975901505576964 ) ) ;
#22927=CARTESIAN_POINT ( 'NONE',  ( -59.59170313451811296, -136.7500000013655779, 1.485763867205729394 ) ) ;
#22935=ORIENTED_EDGE ( 'NONE', *, *, #28051, .T. ) ;
#22954=CARTESIAN_POINT ( 'NONE',  ( -50.70258187064364108, -143.3750000013656063, 2.196230717870141014 ) ) ;
#22964=CARTESIAN_POINT ( 'NONE',  ( -53.33387254593733928, -126.8125000000000568, 5.149110718188519620 ) ) ;
#22971=CARTESIAN_POINT ( 'NONE',  ( -59.59170313451811296, -143.5000000013656347, 1.485763867205729394 ) ) ;
#22983=CARTESIAN_POINT ( 'NONE',  ( -50.18089887299976937, -140.8125000027311557, 2.462841084822427362 ) ) ;
#22987=( BOUNDED_CURVE ( )  B_SPLINE_CURVE ( 2, ( #19432, #34870, #43550, #15244, #58363, #10418, #49009, #14289, #39044 ),
 .UNSPECIFIED., .F., .F. ) 
 B_SPLINE_CURVE_WITH_KNOTS ( ( 3, 2, 2, 2, 3 ),
 ( 0.2750000000000002442, 0.2791666666666668961, 0.2833333333333335480, 0.2875000000000001998, 0.2916666666666669072 ),
 .UNSPECIFIED. ) 
 CURVE ( )  GEOMETRIC_REPRESENTATION_ITEM ( )  RATIONAL_B_SPLINE_CURVE ( ( 0.9999999999999958922, 0.9238795325112908463, 1.000000000000000000, 0.9238795325112867385, 1.000000000000000000, 0.9238795325112867385, 1.000000000000000000, 0.9238795325112826307, 1.000000000000003997 ) ) 
 REPRESENTATION_ITEM ( '' )  );
#22990=CARTESIAN_POINT ( 'NONE',  ( -60.14911071818854538, -140.1875000027312126, 1.666127454062681146 ) ) ;
#22997=CARTESIAN_POINT ( 'NONE',  ( -56.48576386720575471, -149.0000000013656063, -4.591703134518078322 ) ) ;
#23029=CARTESIAN_POINT ( 'NONE',  ( -58.24261429053147765, -155.0000000000000284, -3.805975901505573411 ) ) ;
#23032=CARTESIAN_POINT ( 'NONE',  ( -58.80597590150559739, -139.0000000000000284, 3.242614290531460330 ) ) ;
#23041=CARTESIAN_POINT ( 'NONE',  ( -52.80376928212989185, -140.1250000013656347, -4.297418129356378458 ) ) ;
#23043=CARTESIAN_POINT ( 'NONE',  ( -54.60164318462004474, -129.5000000027312126, -4.984105922594373794 ) ) ;
#23054=CARTESIAN_POINT ( 'NONE',  ( -51.60603307380591787, -126.9375000013656063, -2.891590998281053704 ) ) ;
#23064=CARTESIAN_POINT ( 'NONE',  ( -56.48576386720575471, -130.7500000013656063, -4.591703134518078322 ) ) ;
#23074=CARTESIAN_POINT ( 'NONE',  ( -52.80376928212989185, -128.1250000013656347, -4.297418129356379346 ) ) ;
#23101=CARTESIAN_POINT ( 'NONE',  ( -59.59170313451810586, -135.5000000013656063, 1.485763867205729394 ) ) ;
#23106=CARTESIAN_POINT ( 'NONE',  ( -51.19402409849444524, -151.5000000000000284, -3.242614290531456334 ) ) ;
#23115=CARTESIAN_POINT ( 'NONE',  ( -52.10840900171896806, -150.4375000013656063, 3.393966926194110556 ) ) ;
#23116=CARTESIAN_POINT ( 'NONE',  ( -52.53715891517739323, -142.5625000027312126, -4.819101127000233298 ) ) ;
#23123=CARTESIAN_POINT ( 'NONE',  ( -55.35523342533222291, -135.3125000013656063, 4.444560631937231499 ) ) ;
#23133=PLANE ( 'NONE',  #18229 ) ;
#23137=CARTESIAN_POINT ( 'NONE',  ( -50.40829686548195099, -144.0000000013656063, -1.485763867205728284 ) ) ;
#23175=CARTESIAN_POINT ( 'NONE',  ( -49.85088928181150436, -149.6875000027311842, -1.666127454062680480 ) ) ;
#23180=CARTESIAN_POINT ( 'NONE',  ( -56.48576386720575471, -132.0000000013656063, -4.591703134518078322 ) ) ;
#23188=CARTESIAN_POINT ( 'NONE',  ( -50.18089887299979068, -152.8125000027311842, 2.462841084822635640 ) ) ;
#23195=CARTESIAN_POINT ( 'NONE',  ( -51.19402409849444524, -150.6250000027312126, -3.242614290531456334 ) ) ;
#23223=CARTESIAN_POINT ( 'NONE',  ( -54.64476657466781973, -136.0625000013656063, -4.444560631937228834 ) ) ;
#23258=CARTESIAN_POINT ( 'NONE',  ( -50.70258187064364108, -142.3750000013656063, 2.196230717870141014 ) ) ;
#23280=CARTESIAN_POINT ( 'NONE',  ( -52.10840900171896806, -143.1875000013656063, 3.393966926194110556 ) ) ;
#23307=CARTESIAN_POINT ( 'NONE',  ( -51.60603307380591787, -146.1875000013656063, -2.891590998281053704 ) ) ;
#23315=CARTESIAN_POINT ( 'NONE',  ( -55.39835681537999790, -147.8750000000000284, 4.984105922594378235 ) ) ;
#23338=AXIS2_PLACEMENT_3D ( 'NONE', #56395, #46415, #25840 ) ;
#23341=ORIENTED_EDGE ( 'NONE', *, *, #32775, .F. ) ;
#23350=LINE ( 'NONE', #8238, #55011 ) ;
#23351=CARTESIAN_POINT ( 'NONE',  ( -55.39835681537999790, -134.8750000000000284, 4.984105922594378235 ) ) ;
#23359=CARTESIAN_POINT ( 'NONE',  ( -50.70258187064364108, -140.3750000013656063, 2.196230717870141014 ) ) ;
#23361=CARTESIAN_POINT ( 'NONE',  ( -58.24261429053147765, -126.3750000027312126, -3.805975901505573855 ) ) ;
#23369=DIRECTION ( 'NONE',  ( -0.6485228581062915110, 0.000000000000000000, -0.7611951803011149931 ) ) ;
#23374=CARTESIAN_POINT ( 'NONE',  ( -59.44456063193725015, -125.5625000013655921, -0.3552334253322034230 ) ) ;
#23378=ORIENTED_EDGE ( 'NONE', *, *, #15239, .T. ) ;
#23387=CARTESIAN_POINT ( 'NONE',  ( -52.80376928212989185, -127.8750000013656063, -4.297418129356379346 ) ) ;
#23419=CARTESIAN_POINT ( 'NONE',  ( -59.44456063193725015, -152.8125000013656063, -0.3552334253322034230 ) ) ;
#23423=CARTESIAN_POINT ( 'NONE',  ( -55.35523342533222291, -136.3125000013656063, 4.444560631937231499 ) ) ;
#23429=CARTESIAN_POINT ( 'NONE',  ( -50.18089887299979068, -150.6875000000000284, 2.462841084822635640 ) ) ;
#23430=VECTOR ( 'NONE', #27525, 1000.000000000000000 ) ;
#23439=CARTESIAN_POINT ( 'NONE',  ( -59.59170313451810586, -148.7500000013655779, 1.485763867205729394 ) ) ;
#23440=CARTESIAN_POINT ( 'NONE',  ( -59.98410592259440222, -140.2500000027312126, -0.3983568153799752487 ) ) ;
#23446=CARTESIAN_POINT ( 'NONE',  ( -58.39396692619412477, -137.4375000013656063, 2.891590998281057701 ) ) ;
#23462=CARTESIAN_POINT ( 'NONE',  ( -55.35523342533222291, -140.3125000013656063, 4.444560631937231499 ) ) ;
#23473=CARTESIAN_POINT ( 'NONE',  ( -58.24261429053147765, -149.2500000000000284, -3.805975901505573855 ) ) ;
#23491=CARTESIAN_POINT ( 'NONE',  ( -51.75738570946856498, -146.8750000027312126, 3.805975901505576964 ) ) ;
#23494=CARTESIAN_POINT ( 'NONE',  ( -52.80376928212989185, -152.8750000013656063, -4.297418129356378458 ) ) ;
#23501=CARTESIAN_POINT ( 'NONE',  ( -50.40829686548195099, -130.2500000013656063, -1.485763867205728284 ) ) ;
#23511=( BOUNDED_CURVE ( )  B_SPLINE_CURVE ( 2, ( #43553, #54497, #45796, #26177, #35199, #55459, #25859, #45475, #11689 ),
 .UNSPECIFIED., .F., .F. ) 
 B_SPLINE_CURVE_WITH_KNOTS ( ( 3, 2, 2, 2, 3 ),
 ( 0.6083333333333329485, 0.6124999999999997113, 0.6166666666666663632, 0.6208333333333330151, 0.6249999999999996669 ),
 .UNSPECIFIED. ) 
 CURVE ( )  GEOMETRIC_REPRESENTATION_ITEM ( )  RATIONAL_B_SPLINE_CURVE ( ( 1.000000000000005995, 0.9238795325112806323, 1.000000000000000000, 0.9238795325112867385, 1.000000000000000000, 0.9238795325112867385, 1.000000000000000000, 0.9238795325112928447, 0.9999999999999938938 ) ) 
 REPRESENTATION_ITEM ( '' )  );
#23514=AXIS2_PLACEMENT_3D ( 'NONE', #58544, #54023, #4204 ) ;
#23530=CARTESIAN_POINT ( 'NONE',  ( -58.80597590150559739, -145.0000000000000284, 3.242614290531460330 ) ) ;
#23533=FACE_OUTER_BOUND ( 'NONE', #12258, .T. ) ;
#23546=CARTESIAN_POINT ( 'NONE',  ( -59.44456063193725015, -134.8125000013656063, -0.3552334253322034230 ) ) ;
#23580=CARTESIAN_POINT ( 'NONE',  ( -57.89159099828107458, -144.9375000013656063, -3.393966926194107447 ) ) ;
#23591=CARTESIAN_POINT ( 'NONE',  ( -59.81910112700026616, -143.3125000027312126, -2.462841084822481541 ) ) ;
#23597=CARTESIAN_POINT ( 'NONE',  ( -59.29741812935640155, -144.6250000013656063, -2.196230717870135685 ) ) ;
#23605=EDGE_CURVE ( 'NONE', #32079, #51190, #9302, .T. ) ;
#23625=CARTESIAN_POINT ( 'NONE',  ( -59.44456063193725015, -149.8125000013656063, -0.3552334253322034230 ) ) ;
#23648=CARTESIAN_POINT ( 'NONE',  ( -52.53715891517739323, -135.4375000000000284, -4.819101127000233298 ) ) ;
#23661=CARTESIAN_POINT ( 'NONE',  ( -51.75738570946856498, -133.7500000000000284, 3.805975901505576964 ) ) ;
#23670=CARTESIAN_POINT ( 'NONE',  ( -52.10840900171896806, -137.4375000013656063, 3.393966926194110556 ) ) ;
#23672=CARTESIAN_POINT ( 'NONE',  ( -50.01589407740564042, -125.7500000027311984, 0.3983568153799778022 ) ) ;
#23700=CARTESIAN_POINT ( 'NONE',  ( -53.51423613279429503, -131.2500000013656347, 4.591703134518082763 ) ) ;
#23701=CARTESIAN_POINT ( 'NONE',  ( -57.89159099828107458, -148.6875000013656063, -3.393966926194107447 ) ) ;
#23718=EDGE_CURVE ( 'NONE', #36394, #45194, #62017, .T. ) ;
#23720=CARTESIAN_POINT ( 'NONE',  ( -52.53715891517739323, -137.5625000027312126, -4.819101127000233298 ) ) ;
#23726=CARTESIAN_POINT ( 'NONE',  ( -50.18089887299977647, -144.8125000027312126, 2.462841084822486426 ) ) ;
#23733=CARTESIAN_POINT ( 'NONE',  ( -50.55543936806279248, -152.3125000013656063, 0.3552334253322060320 ) ) ;
#23737=CARTESIAN_POINT ( 'NONE',  ( -50.48477904491434742, -135.0324864422693736, -0.5288446712371500658 ) ) ;
#23742=ORIENTED_EDGE ( 'NONE', *, *, #16593, .T. ) ;
#23744=CARTESIAN_POINT ( 'NONE',  ( -50.18089887299979068, -145.6875000000000000, 2.462841084822635640 ) ) ;
#23750=AXIS2_PLACEMENT_3D ( 'NONE', #9353, #63091, #19001 ) ;
#23753=CARTESIAN_POINT ( 'NONE',  ( -57.19623071787016499, -148.6250000013656063, 4.297418129356382899 ) ) ;
#23754=CARTESIAN_POINT ( 'NONE',  ( -58.24261429053147765, -137.3750000027312126, -3.805975901505573855 ) ) ;
#23761=CARTESIAN_POINT ( 'NONE',  ( -56.48576386720575471, -133.7500000013656063, -4.591703134518078322 ) ) ;
#23766=ORIENTED_EDGE ( 'NONE', *, *, #50419, .T. ) ;
#23774=CARTESIAN_POINT ( 'NONE',  ( -52.10840900171896806, -140.1875000013656063, 3.393966926194110556 ) ) ;
#23804=CARTESIAN_POINT ( 'NONE',  ( -57.89159099828107458, -152.6875000013656063, -3.393966926194107447 ) ) ;
#23811=CARTESIAN_POINT ( 'NONE',  ( -55.35523342533222291, -127.5625000013655921, 4.444560631937231499 ) ) ;
#23820=CARTESIAN_POINT ( 'NONE',  ( -59.98410592259440222, -150.2500000027312126, -0.3983568153799752487 ) ) ;
#23828=CARTESIAN_POINT ( 'NONE',  ( -49.85088928181150436, -150.6875000027312126, -1.666127454062680480 ) ) ;
#23832=EDGE_CURVE ( 'NONE', #24115, #32079, #38839, .T. ) ;
#23841=CARTESIAN_POINT ( 'NONE',  ( -59.29741812935640155, -153.6250000013655779, -2.196230717870135685 ) ) ;
#23852=CARTESIAN_POINT ( 'NONE',  ( -50.01589407740564042, -142.6250000000000284, 0.3983568153799778022 ) ) ;
#23855=CARTESIAN_POINT ( 'NONE',  ( -55.35523342533222291, -137.5625000013656063, 4.444560631937231499 ) ) ;
#23861=CARTESIAN_POINT ( 'NONE',  ( -59.81910112700027327, -140.1875000000000284, -2.462841084822392279 ) ) ;
#23886=CARTESIAN_POINT ( 'NONE',  ( -59.29741812935640155, -144.8750000013655779, -2.196230717870135685 ) ) ;
#23904=CARTESIAN_POINT ( 'NONE',  ( -52.10840900171896806, -146.1875000013656063, 3.393966926194110556 ) ) ;
#23928=CARTESIAN_POINT ( 'NONE',  ( -54.64476657466781973, -149.0625000013656063, -4.444560631937228834 ) ) ;
#23961=EDGE_CURVE ( 'NONE', #26446, #32199, #6005, .T. ) ;
#23963=CARTESIAN_POINT ( 'NONE',  ( -54.60164318462004474, -133.3750000000000284, -4.984105922594373794 ) ) ;
#23966=ORIENTED_EDGE ( 'NONE', *, *, #44808, .T. ) ;
#23975=CARTESIAN_POINT ( 'NONE',  ( -52.53715891517739323, -127.5625000027312552, -4.819101127000233298 ) ) ;
#23982=FACE_OUTER_BOUND ( 'NONE', #3111, .T. ) ;
#23999=CARTESIAN_POINT ( 'NONE',  ( -57.19623071787017210, -131.3750000013656347, 4.297418129356382899 ) ) ;
#24000=CARTESIAN_POINT ( 'NONE',  ( -59.59170313451810586, -148.5000000013655779, 1.485763867205729394 ) ) ;
#24017=( BOUNDED_CURVE ( )  B_SPLINE_CURVE ( 2, ( #1818, #21422, #60669, #16592, #11749, #31367, #22056, #41648, #46812 ),
 .UNSPECIFIED., .F., .F. ) 
 B_SPLINE_CURVE_WITH_KNOTS ( ( 3, 2, 2, 2, 3 ),
 ( 0.6249999999999996669, 0.6291666666666663188, 0.6333333333333328596, 0.6374999999999995115, 0.6416666666666662744 ),
 .UNSPECIFIED. ) 
 CURVE ( )  GEOMETRIC_REPRESENTATION_ITEM ( )  RATIONAL_B_SPLINE_CURVE ( ( 1.000000000000005995, 0.9238795325112806323, 1.000000000000000000, 0.9238795325112867385, 1.000000000000000000, 0.9238795325112867385, 1.000000000000000000, 0.9238795325112948431, 0.9999999999999918954 ) ) 
 REPRESENTATION_ITEM ( '' )  );
#24022=ORIENTED_EDGE ( 'NONE', *, *, #38220, .F. ) ;
#24027=DIRECTION ( 'NONE',  ( 0.000000000000000000, -0.000000000000000000, -1.000000000000000000 ) ) ;
#24034=ORIENTED_EDGE ( 'NONE', *, *, #15413, .T. ) ;
#24035=CARTESIAN_POINT ( 'NONE',  ( -59.29741812935640155, -149.8750000013655779, -2.196230717870135685 ) ) ;
#24041=CARTESIAN_POINT ( 'NONE',  ( -50.70258187064364108, -136.1250000013656063, 2.196230717870141014 ) ) ;
#24046=CARTESIAN_POINT ( 'NONE',  ( -52.53715891517739323, -146.4375000000000000, -4.819101127000233298 ) ) ;
#24058=CARTESIAN_POINT ( 'NONE',  ( -56.48576386720575471, -150.0000000013656063, -4.591703134518078322 ) ) ;
#24059=CARTESIAN_POINT ( 'NONE',  ( -52.53715891517739323, -138.5625000027312126, -4.819101127000233298 ) ) ;
#24069=CARTESIAN_POINT ( 'NONE',  ( -50.18089887299976937, -139.8125000027312126, 2.462841084822397164 ) ) ;
#24070=CARTESIAN_POINT ( 'NONE',  ( -58.39396692619412477, -134.4375000013656063, 2.891590998281057701 ) ) ;
#24086=CARTESIAN_POINT ( 'NONE',  ( -58.39396692619412477, -141.4375000013656063, 2.891590998281057701 ) ) ;
#24115=VERTEX_POINT ( 'NONE', #49974 ) ;
#24118=CARTESIAN_POINT ( 'NONE',  ( -52.80376928212989185, -151.8750000013655779, -4.297418129356378458 ) ) ;
#24125=CARTESIAN_POINT ( 'NONE',  ( -54.64476657466781973, -128.0625000013656063, -4.444560631937228834 ) ) ;
#24131=CARTESIAN_POINT ( 'NONE',  ( -51.75738570946856498, -142.7500000000000284, 3.805975901505576964 ) ) ;
#24134=CARTESIAN_POINT ( 'NONE',  ( -57.46284108482265651, -151.9375000000000284, 4.819101127000238627 ) ) ;
#24135=CARTESIAN_POINT ( 'NONE',  ( -58.24261429053147765, -151.3750000027312126, -3.805975901505573855 ) ) ;
#24138=LINE ( 'NONE', #33471, #7147 ) ;
#24148=CARTESIAN_POINT ( 'NONE',  ( -53.33387254593733218, -153.9375000027311842, 5.149110718188519620 ) ) ;
#24152=CARTESIAN_POINT ( 'NONE',  ( -56.48576386720575471, -151.7500000013655779, -4.591703134518078322 ) ) ;
#24161=DIRECTION ( 'NONE',  ( 0.000000000000000000, 1.000000000000000000, 0.000000000000000000 ) ) ;
#24164=CARTESIAN_POINT ( 'NONE',  ( -49.85088928181150436, -142.5625000000000284, -1.666127454062680480 ) ) ;
#24167=CARTESIAN_POINT ( 'NONE',  ( -57.89159099828107458, -132.9375000013656063, -3.393966926194107447 ) ) ;
#24193=CARTESIAN_POINT ( 'NONE',  ( -52.80376928212989185, -139.1250000013656063, -4.297418129356379346 ) ) ;
#24205=CARTESIAN_POINT ( 'NONE',  ( -55.00000000000001421, -135.0000000000000284, -8.082903768654752241 ) ) ;
#24213=CARTESIAN_POINT ( 'NONE',  ( -59.59170313451811296, -144.5000000013656063, 1.485763867205729394 ) ) ;
#24223=CARTESIAN_POINT ( 'NONE',  ( -55.39835681537999790, -141.8750000000000284, 4.984105922594378235 ) ) ;
#24230=CARTESIAN_POINT ( 'NONE',  ( -60.14911071818854538, -144.0625000000000000, 1.666127454062681146 ) ) ;
#24238=CARTESIAN_POINT ( 'NONE',  ( -59.44456063193725015, -148.8125000013656063, -0.3552334253322034230 ) ) ;
#24252=DIRECTION ( 'NONE',  ( -0.000000000000000000, -1.000000000000000000, 0.000000000000000000 ) ) ;
#24272=UNCERTAINTY_MEASURE_WITH_UNIT (LENGTH_MEASURE( 1.000000000000000082E-05 ), #7698, 'distance_accuracy_value', 'NONE');
#24275=CARTESIAN_POINT ( 'NONE',  ( -50.01589407740564042, -134.6250000000000284, 0.3983568153799778022 ) ) ;
#24283=VERTEX_POINT ( 'NONE', #62501 ) ;
#24285=CARTESIAN_POINT ( 'NONE',  ( -52.53715891517739323, -125.5625000027312552, -4.819101127000233298 ) ) ;
#24309=CARTESIAN_POINT ( 'NONE',  ( -52.80376928212989185, -128.8750000013656063, -4.297418129356379346 ) ) ;
#24310=CARTESIAN_POINT ( 'NONE',  ( -53.51423613279429503, -148.2500000013656347, 4.591703134518083651 ) ) ;
#24322=CARTESIAN_POINT ( 'NONE',  ( -58.39396692619412477, -124.6875000013656063, 2.891590998281057701 ) ) ;
#24349=CARTESIAN_POINT ( 'NONE',  ( -50.55543936806279248, -151.3125000013656063, 0.3552334253322060320 ) ) ;
#24359=CARTESIAN_POINT ( 'NONE',  ( -51.19402409849444524, -147.5000000000000284, -3.242614290531456334 ) ) ;
#24361=VERTEX_POINT ( 'NONE', #37410 ) ;
#24367=CARTESIAN_POINT ( 'NONE',  ( -54.64476657466781973, -145.0625000013656063, -4.444560631937228834 ) ) ;
#24368=CARTESIAN_POINT ( 'NONE',  ( -50.18089887299979068, -138.8125000027311842, 2.462841084822635640 ) ) ;
#24381=CARTESIAN_POINT ( 'NONE',  ( -52.80376928212989185, -131.8750000013656347, -4.297418129356379346 ) ) ;
#24383=CARTESIAN_POINT ( 'NONE',  ( -59.98410592259440222, -146.2500000027312126, -0.3983568153799752487 ) ) ;
#24391=CARTESIAN_POINT ( 'NONE',  ( -52.53715891517739323, -143.5625000027312126, -4.819101127000233298 ) ) ;
#24395=CARTESIAN_POINT ( 'NONE',  ( -59.44456063193725015, -141.5625000013656063, -0.3552334253322034230 ) ) ;
#24403=VERTEX_POINT ( 'NONE', #52203 ) ;
#24407=ADVANCED_FACE ( 'NONE', ( #27750 ), #47378, .F. ) ;
#24410=EDGE_CURVE ( 'NONE', #2425, #17633, #36806, .T. ) ;
#24430=CARTESIAN_POINT ( 'NONE',  ( -50.70258187064364108, -153.1250000013656063, 2.196230717870141014 ) ) ;
#24436=CARTESIAN_POINT ( 'NONE',  ( -57.19623071787017210, -126.6250000013656489, 4.297418129356382899 ) ) ;
#24446=CARTESIAN_POINT ( 'NONE',  ( -57.46284108482265651, -152.0625000027311842, 4.819101127000239515 ) ) ;
#24448=ORIENTED_EDGE ( 'NONE', *, *, #38544, .F. ) ;
#24506=CARTESIAN_POINT ( 'NONE',  ( -56.66612745406251861, -136.3125000000000000, -5.149110718188501856 ) ) ;
#24516=CARTESIAN_POINT ( 'NONE',  ( -59.29741812935640155, -139.8750000013655779, -2.196230717870135685 ) ) ;
#24519=ORIENTED_EDGE ( 'NONE', *, *, #40264, .F. ) ;
#24526=CARTESIAN_POINT ( 'NONE',  ( -51.19402409849444524, -140.5000000000000000, -3.242614290531456334 ) ) ;
#24533=CARTESIAN_POINT ( 'NONE',  ( -51.60603307380591787, -139.9375000013656063, -2.891590998281053704 ) ) ;
#24534=CARTESIAN_POINT ( 'NONE',  ( -53.33387254593733218, -154.8125000000000000, 5.149110718188519620 ) ) ;
#24559=( BOUNDED_CURVE ( )  B_SPLINE_CURVE ( 2, ( #61660, #37210, #56836, #13697, #32375, #51999, #43275, #28172, #8560 ),
 .UNSPECIFIED., .F., .F. ) 
 B_SPLINE_CURVE_WITH_KNOTS ( ( 3, 2, 2, 2, 3 ),
 ( 0.09166666666666674346, 0.09583333333333342308, 0.1000000000000000888, 0.1041666666666667546, 0.1083333333333334203 ),
 .UNSPECIFIED. ) 
 CURVE ( )  GEOMETRIC_REPRESENTATION_ITEM ( )  RATIONAL_B_SPLINE_CURVE ( ( 0.9999999999999984457, 0.9238795325112882928, 1.000000000000000000, 0.9238795325112867385, 1.000000000000000000, 0.9238795325112867385, 1.000000000000000000, 0.9238795325112851842, 1.000000000000001554 ) ) 
 REPRESENTATION_ITEM ( '' )  );
#24560=CARTESIAN_POINT ( 'NONE',  ( -52.80376928212989185, -144.1250000013656063, -4.297418129356379346 ) ) ;
#24571=ORIENTED_EDGE ( 'NONE', *, *, #10330, .T. ) ;
#24595=VERTEX_POINT ( 'NONE', #63125 ) ;
#24598=CARTESIAN_POINT ( 'NONE',  ( -52.53715891517739323, -134.4375000000000284, -4.819101127000233298 ) ) ;
#24601=ORIENTED_EDGE ( 'NONE', *, *, #23832, .T. ) ;
#24607=CARTESIAN_POINT ( 'NONE',  ( -53.33387254593733928, -127.9375000027312126, 5.149110718188519620 ) ) ;
#24631=CARTESIAN_POINT ( 'NONE',  ( -52.80376928212989185, -126.8750000013656205, -4.297418129356379346 ) ) ;
#24632=CARTESIAN_POINT ( 'NONE',  ( -58.39396692619412477, -145.4375000013656063, 2.891590998281057701 ) ) ;
#24665=CARTESIAN_POINT ( 'NONE',  ( -56.48576386720575471, -150.0000000013655779, -4.591703134518078322 ) ) ;
#24676=CARTESIAN_POINT ( 'NONE',  ( -50.18089887299979068, -146.6875000000000284, 2.462841084822635640 ) ) ;
#24683=CARTESIAN_POINT ( 'NONE',  ( -58.39396692619412477, -146.6875000013656063, 2.891590998281057701 ) ) ;
#24685=CARTESIAN_POINT ( 'NONE',  ( -59.81910112700025905, -137.3125000027312126, -2.462841084822630311 ) ) ;
#24700=CARTESIAN_POINT ( 'NONE',  ( -55.35523342533222291, -132.3125000013656063, 4.444560631937231499 ) ) ;
#24715=CARTESIAN_POINT ( 'NONE',  ( -58.39396692619412477, -143.4375000013656063, 2.891590998281057701 ) ) ;
#24753=CARTESIAN_POINT ( 'NONE',  ( -50.40829686548195099, -128.2500000013656063, -1.485763867205728284 ) ) ;
#24766=CARTESIAN_POINT ( 'NONE',  ( -50.01589407740564042, -151.7500000027312410, 0.3983568153799778022 ) ) ;
#24768=EDGE_LOOP ( 'NONE', ( #22642, #38058, #37826, #24034 ) ) ;
#24785=CARTESIAN_POINT ( 'NONE',  ( -59.29741812935640155, -152.6250000013656063, -2.196230717870135685 ) ) ;
#24824=CARTESIAN_POINT ( 'NONE',  ( -52.53715891517739323, -136.4375000000000000, -4.819101127000233298 ) ) ;
#24832=CARTESIAN_POINT ( 'NONE',  ( -54.64476657466781973, -140.0625000013656063, -4.444560631937228834 ) ) ;
#24837=EDGE_CURVE ( 'NONE', #16286, #42590, #29822, .T. ) ;
#24854=CARTESIAN_POINT ( 'NONE',  ( -57.19623071787017210, -140.3750000013656063, 4.297418129356382899 ) ) ;
#24858=ORIENTED_EDGE ( 'NONE', *, *, #16862, .F. ) ;
#24870=CARTESIAN_POINT ( 'NONE',  ( -55.00000000000002132, -155.0000000000000284, 1.734723475976807094E-15 ) ) ;
#24881=CARTESIAN_POINT ( 'NONE',  ( -59.29741812935640155, -142.8750000013656063, -2.196230717870135685 ) ) ;
#24919=CARTESIAN_POINT ( 'NONE',  ( -51.19402409849444524, -131.5000000000000284, -3.242614290531456334 ) ) ;
#24926=ORIENTED_EDGE ( 'NONE', *, *, #51902, .F. ) ;
#24928=CARTESIAN_POINT ( 'NONE',  ( -60.14911071818854538, -124.1875000027312410, 1.666127454062681368 ) ) ;
#24930=CARTESIAN_POINT ( 'NONE',  ( -50.75781946612335105, -135.0000000000005969, -1.372666862511563224 ) ) ;
#24931=LINE ( 'NONE', #44216, #36375 ) ;
#24933=CARTESIAN_POINT ( 'NONE',  ( -51.75738570946856498, -145.7500000000000284, 3.805975901505576964 ) ) ;
#24953=CARTESIAN_POINT ( 'NONE',  ( -52.10840900171896806, -154.4375000013656063, 3.393966926194110556 ) ) ;
#24955=CARTESIAN_POINT ( 'NONE',  ( -58.39396692619412477, -147.4375000013656063, 2.891590998281057701 ) ) ;
#24980=ORIENTED_EDGE ( 'NONE', *, *, #53080, .T. ) ;
#24981=PLANE ( 'NONE',  #15191 ) ;
#24985=CARTESIAN_POINT ( 'NONE',  ( -50.40829686548195099, -147.2500000013656063, -1.485763867205728284 ) ) ;
#24994=CARTESIAN_POINT ( 'NONE',  ( -51.75738570946856498, -143.7500000000000284, 3.805975901505576964 ) ) ;
#24996=CARTESIAN_POINT ( 'NONE',  ( -58.24261429053147765, -155.0000000000000284, -3.805975901505573411 ) ) ;
#25001=CARTESIAN_POINT ( 'NONE',  ( -52.80376928212989185, -146.1250000013656063, -4.297418129356378458 ) ) ;
#25003=CARTESIAN_POINT ( 'NONE',  ( -53.33387254593733928, -135.9375000027311842, 5.149110718188519620 ) ) ;
#25016=CARTESIAN_POINT ( 'NONE',  ( -57.89159099828107458, -133.6875000013656063, -3.393966926194107447 ) ) ;
#25019=CARTESIAN_POINT ( 'NONE',  ( -52.53715891517739323, -146.5625000027311842, -4.819101127000233298 ) ) ;
#25031=CARTESIAN_POINT ( 'NONE',  ( -57.19623071787017210, -137.3750000013656063, 4.297418129356382899 ) ) ;
#25060=DIRECTION ( 'NONE',  ( 0.000000000000000000, 1.000000000000000000, 0.000000000000000000 ) ) ;
#25062=ORIENTED_EDGE ( 'NONE', *, *, #542, .T. ) ;
#25063=CARTESIAN_POINT ( 'NONE',  ( -54.64476657466781973, -148.8125000013656063, -4.444560631937228834 ) ) ;
#25070=CARTESIAN_POINT ( 'NONE',  ( -52.10840900171896806, -126.4375000013656063, 3.393966926194110556 ) ) ;
#25081=CARTESIAN_POINT ( 'NONE',  ( -51.75738570946856498, -150.8750000027312126, 3.805975901505576964 ) ) ;
#25099=CARTESIAN_POINT ( 'NONE',  ( -51.60603307380591787, -150.9375000013656063, -2.891590998281053704 ) ) ;
#25132=ORIENTED_EDGE ( 'NONE', *, *, #1728, .F. ) ;
#25135=ADVANCED_FACE ( 'NONE', ( #19599 ), #48233, .F. ) ;
#25145=CARTESIAN_POINT ( 'NONE',  ( -58.39396692619412477, -140.6875000013656063, 2.891590998281057701 ) ) ;
#25148=ORIENTED_EDGE ( 'NONE', *, *, #1467, .T. ) ;
#25152=CARTESIAN_POINT ( 'NONE',  ( -52.70900849189143855, -134.9999999999999432, -3.836432292133860944 ) ) ;
#25155=CARTESIAN_POINT ( 'NONE',  ( -55.39835681537999790, -143.0000000027312126, 4.984105922594378235 ) ) ;
#25162=CARTESIAN_POINT ( 'NONE',  ( -59.44456063193725015, -141.5625000013656063, -0.3552334253322034230 ) ) ;
#25189=CARTESIAN_POINT ( 'NONE',  ( -57.89159099828107458, -145.9375000013656063, -3.393966926194107447 ) ) ;
#25191=EDGE_CURVE ( 'NONE', #24595, #35208, #12561, .T. ) ;
#25206=LINE ( 'NONE', #22622, #4225 ) ;
#25218=CARTESIAN_POINT ( 'NONE',  ( -51.75738570946856498, -150.7500000000000284, 3.805975901505576964 ) ) ;
#25229=CARTESIAN_POINT ( 'NONE',  ( -57.46284108482265651, -149.0625000027312126, 4.819101127000238627 ) ) ;
#25235=CARTESIAN_POINT ( 'NONE',  ( -50.18089887299979068, -130.6875000000000284, 2.462841084822635640 ) ) ;
#25241=CARTESIAN_POINT ( 'NONE',  ( -52.10840900171896806, -153.1875000013656063, 3.393966926194110556 ) ) ;
#25244=DIRECTION ( 'NONE',  ( 0.000000000000000000, -1.000000000000000000, 0.000000000000000000 ) ) ;
#25266=CARTESIAN_POINT ( 'NONE',  ( -58.39396692619412477, -126.4375000013656063, 2.891590998281057701 ) ) ;
#25267=CARTESIAN_POINT ( 'NONE',  ( -59.59170313451810586, -143.5000000013656063, 1.485763867205729394 ) ) ;
#25281=LINE ( 'NONE', #15639, #32923 ) ;
#25296=EDGE_CURVE ( 'NONE', #33278, #18086, #54254, .T. ) ;
#25311=CARTESIAN_POINT ( 'NONE',  ( -59.81910112700025905, -140.1875000000000000, -2.462841084822630311 ) ) ;
#25320=CARTESIAN_POINT ( 'NONE',  ( -50.55543936806279248, -145.3125000013656063, 0.3552334253322060320 ) ) ;
#25322=CARTESIAN_POINT ( 'NONE',  ( -52.53715891517739323, -134.5625000027312126, -4.819101127000233298 ) ) ;
#25334=CARTESIAN_POINT ( 'NONE',  ( -50.70258187064364108, -128.1250000013656347, 2.196230717870141014 ) ) ;
#25350=CARTESIAN_POINT ( 'NONE',  ( -51.60603307380591787, -138.9375000013656063, -2.891590998281053704 ) ) ;
#25360=CARTESIAN_POINT ( 'NONE',  ( -54.64476657466781973, -133.0625000013656063, -4.444560631937228834 ) ) ;
#25368=CARTESIAN_POINT ( 'NONE',  ( -50.18089887299978358, -151.6875000000000284, 2.462841084822590787 ) ) ;
#25383=CARTESIAN_POINT ( 'NONE',  ( -51.60603307380591787, -149.9375000013656063, -2.891590998281053704 ) ) ;
#25390=CARTESIAN_POINT ( 'NONE',  ( -60.14911071818854538, -153.0625000000000000, 1.666127454062681368 ) ) ;
#25399=CARTESIAN_POINT ( 'NONE',  ( -51.75738570946856498, -149.7500000000000284, 3.805975901505576964 ) ) ;
#25402=CARTESIAN_POINT ( 'NONE',  ( -54.60164318462004474, -148.5000000027312126, -4.984105922594373794 ) ) ;
#25412=( BOUNDED_CURVE ( )  B_SPLINE_CURVE ( 2, ( #8767, #28375, #9078, #43166, #57975, #14837, #43478, #62805, #38651 ),
 .UNSPECIFIED., .F., .F. ) 
 B_SPLINE_CURVE_WITH_KNOTS ( ( 3, 2, 2, 2, 3 ),
 ( 0.3250000000000002887, 0.3291666666666669405, 0.3333333333333335924, 0.3375000000000002998, 0.3416666666666669516 ),
 .UNSPECIFIED. ) 
 CURVE ( )  GEOMETRIC_REPRESENTATION_ITEM ( )  RATIONAL_B_SPLINE_CURVE ( ( 0.9999999999999948930, 0.9238795325112918455, 1.000000000000000000, 0.9238795325112867385, 1.000000000000000000, 0.9238795325112867385, 1.000000000000000000, 0.9238795325112816315, 1.000000000000005107 ) ) 
 REPRESENTATION_ITEM ( '' )  );
#25418=CARTESIAN_POINT ( 'NONE',  ( -52.53715891517739323, -143.4375000000000284, -4.819101127000233298 ) ) ;
#25420=CARTESIAN_POINT ( 'NONE',  ( -50.40829686548195099, -151.0000000013656063, -1.485763867205728284 ) ) ;
#25450=CARTESIAN_POINT ( 'NONE',  ( -58.24261429053147765, -147.3750000027312126, -3.805975901505573855 ) ) ;
#25453=VERTEX_POINT ( 'NONE', #49455 ) ;
#25456=ORIENTED_EDGE ( 'NONE', *, *, #37409, .F. ) ;
#25464=CARTESIAN_POINT ( 'NONE',  ( -50.55543936806279248, -137.3125000013656063, 0.3552334253322060320 ) ) ;
#25482=CARTESIAN_POINT ( 'NONE',  ( -56.48576386720575471, -140.7500000013655779, -4.591703134518078322 ) ) ;
#25510=CARTESIAN_POINT ( 'NONE',  ( -51.60603307380591787, -143.1875000013656063, -2.891590998281053704 ) ) ;
#25551=CARTESIAN_POINT ( 'NONE',  ( -59.98410592259440222, -129.1250000000000284, -0.3983568153799752487 ) ) ;
#25562=CARTESIAN_POINT ( 'NONE',  ( -51.19402409849444524, -124.6250000027312126, -3.242614290531456334 ) ) ;
#25590=CARTESIAN_POINT ( 'NONE',  ( -53.51423613279429503, -127.2500000013656347, 4.591703134518082763 ) ) ;
#25591=CARTESIAN_POINT ( 'NONE',  ( -58.39396692619412477, -141.4375000013656063, 2.891590998281057701 ) ) ;
#25614=EDGE_LOOP ( 'NONE', ( #17834, #25456, #43988, #13741 ) ) ;
#25631=CARTESIAN_POINT ( 'NONE',  ( -51.19402409849444524, -142.5000000000000284, -3.242614290531456334 ) ) ;
#25641=CARTESIAN_POINT ( 'NONE',  ( -50.40829686548195099, -147.2500000013656063, -1.485763867205728284 ) ) ;
#25643=CARTESIAN_POINT ( 'NONE',  ( -51.19402409849444524, -135.6250000027312410, -3.242614290531456334 ) ) ;
#25646=EDGE_CURVE ( 'NONE', #25453, #7221, #58399, .T. ) ;
#25647=CARTESIAN_POINT ( 'NONE',  ( -58.24261429053147765, -155.0000000000000284, -3.805975901505573411 ) ) ;
#25652=EDGE_CURVE ( 'NONE', #15950, #40878, #9493, .T. ) ;
#25658=CARTESIAN_POINT ( 'NONE',  ( -55.35523342533222291, -129.3125000013656063, 4.444560631937231499 ) ) ;
#25666=CYLINDRICAL_SURFACE ( 'NONE', #4863, 5.000000000000000000 ) ;
#25676=CARTESIAN_POINT ( 'NONE',  ( -50.55543936806279248, -139.0625000013656063, 0.3552334253322060320 ) ) ;
#25686=CARTESIAN_POINT ( 'NONE',  ( -54.64476657466781973, -131.0625000013656063, -4.444560631937228834 ) ) ;
#25710=CARTESIAN_POINT ( 'NONE',  ( -53.51423613279429503, -151.2500000013656063, 4.591703134518083651 ) ) ;
#25717=CYLINDRICAL_SURFACE ( 'NONE', #34374, 5.000000000000000000 ) ;
#25719=CARTESIAN_POINT ( 'NONE',  ( -52.80376928212989185, -125.1250000013656205, -4.297418129356379346 ) ) ;
#25729=CARTESIAN_POINT ( 'NONE',  ( -51.19402409849444524, -147.6250000027312126, -3.242614290531456334 ) ) ;
#25745=CARTESIAN_POINT ( 'NONE',  ( -50.55543936806279248, -151.0625000013656063, 0.3552334253322060320 ) ) ;
#25787=CARTESIAN_POINT ( 'NONE',  ( -58.80597590150559739, -141.1250000027312126, 3.242614290531460330 ) ) ;
#25794=CARTESIAN_POINT ( 'NONE',  ( -52.80376928212989185, -135.1250000013656063, -4.297418129356379346 ) ) ;
#25802=( BOUNDED_CURVE ( )  B_SPLINE_CURVE ( 2, ( #62872, #15795, #13964, #63185, #19424, #38714, #58353, #53523, #1025 ),
 .UNSPECIFIED., .F., .F. ) 
 B_SPLINE_CURVE_WITH_KNOTS ( ( 3, 2, 2, 2, 3 ),
 ( 0.4583333333333337589, 0.4625000000000004663, 0.4666666666666671182, 0.4708333333333337700, 0.4750000000000004219 ),
 .UNSPECIFIED. ) 
 CURVE ( )  GEOMETRIC_REPRESENTATION_ITEM ( )  RATIONAL_B_SPLINE_CURVE ( ( 0.9999999999999918954, 0.9238795325112948431, 1.000000000000000000, 0.9238795325112867385, 1.000000000000000000, 0.9238795325112867385, 1.000000000000000000, 0.9238795325112786339, 1.000000000000008216 ) ) 
 REPRESENTATION_ITEM ( '' )  );
#25810=CARTESIAN_POINT ( 'NONE',  ( -57.89159099828107458, -139.6875000013656063, -3.393966926194107447 ) ) ;
#25833=CARTESIAN_POINT ( 'NONE',  ( -54.64476657466781973, -143.0625000013656063, -4.444560631937228834 ) ) ;
#25840=DIRECTION ( 'NONE',  ( -0.6485228581062915110, 0.000000000000000000, -0.7611951803011149931 ) ) ;
#25859=CARTESIAN_POINT ( 'NONE',  ( -54.60164318462004474, -135.5000000027312126, -4.984105922594373794 ) ) ;
#25863=ADVANCED_FACE ( 'NONE', ( #63545 ), #47791, .F. ) ;
#25874=CARTESIAN_POINT ( 'NONE',  ( -52.53715891517739323, -129.4375000000000568, -4.819101127000233298 ) ) ;
#25881=CARTESIAN_POINT ( 'NONE',  ( -57.89159099828107458, -153.6875000013656063, -3.393966926194107447 ) ) ;
#25895=LINE ( 'NONE', #21076, #54206 ) ;
#25905=CARTESIAN_POINT ( 'NONE',  ( -52.10840900171896806, -125.1875000013656063, 3.393966926194110556 ) ) ;
#25906=CARTESIAN_POINT ( 'NONE',  ( -52.10840900171896806, -143.1875000013656063, 3.393966926194110556 ) ) ;
#25934=ADVANCED_FACE ( 'NONE', ( #23982 ), #33322, .F. ) ;
#25936=VERTEX_POINT ( 'NONE', #55169 ) ;
#25948=CARTESIAN_POINT ( 'NONE',  ( -55.39835681537999790, -142.8750000000000284, 4.984105922594378235 ) ) ;
#25957=CARTESIAN_POINT ( 'NONE',  ( -50.40829686548195099, -141.2500000013656063, -1.485763867205728284 ) ) ;
#25959=CARTESIAN_POINT ( 'NONE',  ( -59.98410592259440222, -135.2500000027312126, -0.3983568153799752487 ) ) ;
#25973=CARTESIAN_POINT ( 'NONE',  ( -50.70258187064364108, -130.1250000013656347, 2.196230717870141014 ) ) ;
#25979=ORIENTED_EDGE ( 'NONE', *, *, #57550, .T. ) ;
#25988=CARTESIAN_POINT ( 'NONE',  ( -55.35523342533222291, -137.3125000013656063, 4.444560631937231499 ) ) ;
#25996=EDGE_LOOP ( 'NONE', ( #12018, #14058, #10217, #1571 ) ) ;
#25999=CARTESIAN_POINT ( 'NONE',  ( -56.48576386720575471, -134.0000000013656063, -4.591703134518078322 ) ) ;
#26035=CARTESIAN_POINT ( 'NONE',  ( -54.64476657466781973, -125.0625000013655921, -4.444560631937228834 ) ) ;
#26042=VERTEX_POINT ( 'NONE', #26854 ) ;
#26043=CARTESIAN_POINT ( 'NONE',  ( -59.29741812935640155, -153.8750000013655779, -2.196230717870135685 ) ) ;
#26045=CARTESIAN_POINT ( 'NONE',  ( -59.81910112700025905, -147.3125000027312410, -2.462841084822630311 ) ) ;
#26063=CARTESIAN_POINT ( 'NONE',  ( -55.35523342533222291, -150.3125000013656063, 4.444560631937231499 ) ) ;
#26109=CARTESIAN_POINT ( 'NONE',  ( -57.19623071787017210, -135.6250000013655779, 4.297418129356382899 ) ) ;
#26116=CARTESIAN_POINT ( 'NONE',  ( -51.79594014233510535, -135.0000000000000000, -3.114416876829539937 ) ) ;
#26117=ORIENTED_EDGE ( 'NONE', *, *, #51226, .T. ) ;
#26150=CARTESIAN_POINT ( 'NONE',  ( -50.55543936806279248, -138.3125000013656063, 0.3552334253322060320 ) ) ;
#26168=CARTESIAN_POINT ( 'NONE',  ( -56.48576386720575471, -136.0000000013656063, -4.591703134518078322 ) ) ;
#26177=CARTESIAN_POINT ( 'NONE',  ( -49.85088928181150436, -135.6875000027311842, -1.666127454062680480 ) ) ;
#26181=CARTESIAN_POINT ( 'NONE',  ( -51.60603307380591787, -148.1875000013656063, -2.891590998281053704 ) ) ;
#26188=CARTESIAN_POINT ( 'NONE',  ( -58.24261429053147765, -140.2500000000000000, -3.805975901505573855 ) ) ;
#26192=CARTESIAN_POINT ( 'NONE',  ( -58.80597590150559739, -128.0000000000000284, 3.242614290531460330 ) ) ;
#26199=CARTESIAN_POINT ( 'NONE',  ( -59.59170313451811296, -152.5000000013655779, 1.485763867205729394 ) ) ;
#26216=PLANE ( 'NONE',  #11464 ) ;
#26223=CARTESIAN_POINT ( 'NONE',  ( -57.89159099828107458, -153.9375000013656063, -3.393966926194107447 ) ) ;
#26224=CARTESIAN_POINT ( 'NONE',  ( -59.44456063193725015, -144.5625000013656063, -0.3552334253322034230 ) ) ;
#26227=CARTESIAN_POINT ( 'NONE',  ( -59.81910112700027327, -137.1875000000000000, -2.462841084822392279 ) ) ;
#26240=LINE ( 'NONE', #30423, #22197 ) ;
#26258=CARTESIAN_POINT ( 'NONE',  ( -51.19402409849444524, -143.5000000000000284, -3.242614290531456334 ) ) ;
#26269=CARTESIAN_POINT ( 'NONE',  ( -57.89159099828107458, -141.9375000013656063, -3.393966926194107447 ) ) ;
#26271=CARTESIAN_POINT ( 'NONE',  ( -59.81910112700025905, -136.3125000027312126, -2.462841084822630311 ) ) ;
#26284=CARTESIAN_POINT ( 'NONE',  ( -50.70258187064364108, -127.1250000013656205, 2.196230717870141014 ) ) ;
#26297=CARTESIAN_POINT ( 'NONE',  ( -56.48576386720575471, -133.7500000013656063, -4.591703134518078322 ) ) ;
#26298=EDGE_CURVE ( 'NONE', #59631, #2425, #47954, .T. ) ;
#26306=CYLINDRICAL_SURFACE ( 'NONE', #46281, 5.000000000000000000 ) ;
#26309=CARTESIAN_POINT ( 'NONE',  ( -59.44456063193725015, -130.8125000013656063, -0.3552334253322034230 ) ) ;
#26325=( BOUNDED_CURVE ( )  B_SPLINE_CURVE ( 2, ( #11593, #27032, #16108, #32160, #1977, #11908, #60821, #55362, #12864 ),
 .UNSPECIFIED., .F., .F. ) 
 B_SPLINE_CURVE_WITH_KNOTS ( ( 3, 2, 2, 2, 3 ),
 ( 0.05833333333333338283, 0.06250000000000005551, 0.06666666666666672125, 0.07083333333333338699, 0.07500000000000005274 ),
 .UNSPECIFIED. ) 
 CURVE ( )  GEOMETRIC_REPRESENTATION_ITEM ( )  RATIONAL_B_SPLINE_CURVE ( ( 0.9999999999999991118, 0.9238795325112876267, 1.000000000000000000, 0.9238795325112867385, 1.000000000000000000, 0.9238795325112867385, 1.000000000000000000, 0.9238795325112857393, 1.000000000000001110 ) ) 
 REPRESENTATION_ITEM ( '' )  );
#26344=CARTESIAN_POINT ( 'NONE',  ( -57.46284108482265651, -153.9375000000000284, 4.819101127000239515 ) ) ;
#26354=CARTESIAN_POINT ( 'NONE',  ( -51.19402409849444524, -148.6250000027312126, -3.242614290531456334 ) ) ;
#26357=EDGE_CURVE ( 'NONE', #43968, #19989, #15940, .T. ) ;
#26368=( BOUNDED_CURVE ( )  B_SPLINE_CURVE ( 2, ( #20399, #50621, #40960, #470, #5285, #20071, #34874, #5601, #25218 ),
 .UNSPECIFIED., .F., .F. ) 
 B_SPLINE_CURVE_WITH_KNOTS ( ( 3, 2, 2, 2, 3 ),
 ( 0.1250000000000001110, 0.1291666666666667906, 0.1333333333333334425, 0.1375000000000001221, 0.1416666666666667740 ),
 .UNSPECIFIED. ) 
 CURVE ( )  GEOMETRIC_REPRESENTATION_ITEM ( )  RATIONAL_B_SPLINE_CURVE ( ( 0.9999999999999980016, 0.9238795325112887369, 1.000000000000000000, 0.9238795325112867385, 1.000000000000000000, 0.9238795325112867385, 1.000000000000000000, 0.9238795325112847401, 1.000000000000001998 ) ) 
 REPRESENTATION_ITEM ( '' )  );
#26378=CARTESIAN_POINT ( 'NONE',  ( -54.64476657466781973, -148.8125000013656063, -4.444560631937228834 ) ) ;
#26423=CARTESIAN_POINT ( 'NONE',  ( -51.60603307380591787, -137.1875000013656063, -2.891590998281053704 ) ) ;
#26445=DIRECTION ( 'NONE',  ( -0.6485228581062915110, 0.000000000000000000, -0.7611951803011149931 ) ) ;
#26446=VERTEX_POINT ( 'NONE', #6450 ) ;
#26471=CARTESIAN_POINT ( 'NONE',  ( -57.19623071787017210, -141.6250000013656063, 4.297418129356382899 ) ) ;
#26480=ORIENTED_EDGE ( 'NONE', *, *, #17333, .F. ) ;
#26491=CARTESIAN_POINT ( 'NONE',  ( -52.10840900171896806, -135.4375000013656063, 3.393966926194110556 ) ) ;
#26496=CARTESIAN_POINT ( 'NONE',  ( -53.33387254593703375, -138.8125000000000000, 5.149110718188541824 ) ) ;
#26498=VECTOR ( 'NONE', #60644, 1000.000000000000227 ) ;
#26504=CARTESIAN_POINT ( 'NONE',  ( -52.80376928212989185, -148.1250000013656063, -4.297418129356379346 ) ) ;
#26521=CARTESIAN_POINT ( 'NONE',  ( -56.48576386720575471, -148.7500000013655779, -4.591703134518078322 ) ) ;
#26522=CARTESIAN_POINT ( 'NONE',  ( -55.39835681537999790, -150.0000000027312126, 4.984105922594378235 ) ) ;
#26525=ORIENTED_EDGE ( 'NONE', *, *, #48349, .F. ) ;
#26546=CARTESIAN_POINT ( 'NONE',  ( -50.55543936806279248, -152.3125000013656063, 0.3552334253322060320 ) ) ;
#26547=CARTESIAN_POINT ( 'NONE',  ( -52.80376928212989185, -142.8750000013656063, -4.297418129356378458 ) ) ;
#26586=CARTESIAN_POINT ( 'NONE',  ( -60.14911071818854538, -140.0625000000000000, 1.666127454062681368 ) ) ;
#26590=ORIENTED_EDGE ( 'NONE', *, *, #15430, .T. ) ;
#26593=CARTESIAN_POINT ( 'NONE',  ( -57.46284108482265651, -137.0625000027312126, 4.819101127000238627 ) ) ;
#26594=EDGE_LOOP ( 'NONE', ( #40194, #1073, #17499 ) ) ;
#26596=CARTESIAN_POINT ( 'NONE',  ( -59.44456063193725015, -143.8125000013656063, -0.3552334253322034230 ) ) ;
#26599=CARTESIAN_POINT ( 'NONE',  ( -53.33387254593733928, -131.9375000027312126, 5.149110718188519620 ) ) ;
#26610=CARTESIAN_POINT ( 'NONE',  ( -59.29741812935640155, -128.6250000013656063, -2.196230717870135685 ) ) ;
#26622=CARTESIAN_POINT ( 'NONE',  ( -59.59170313451811296, -134.5000000013656063, 1.485763867205729394 ) ) ;
#26633=CARTESIAN_POINT ( 'NONE',  ( -58.39396692619412477, -129.6875000013656063, 2.891590998281057701 ) ) ;
#26657=CARTESIAN_POINT ( 'NONE',  ( -51.75738570946856498, -150.8750000027312126, 3.805975901505576964 ) ) ;
#26658=CARTESIAN_POINT ( 'NONE',  ( -62.00000000000001421, -135.0000000000000284, -4.041451884327373456 ) ) ;
#26662=CARTESIAN_POINT ( 'NONE',  ( -52.80376928212989185, -136.8750000013656063, -4.297418129356378458 ) ) ;
#26667=CARTESIAN_POINT ( 'NONE',  ( -50.01589407740564042, -152.6250000000000284, 0.3983568153799778022 ) ) ;
#26679=CARTESIAN_POINT ( 'NONE',  ( -50.01589407740564042, -144.7500000027312126, 0.3983568153799778022 ) ) ;
#26701=CARTESIAN_POINT ( 'NONE',  ( -52.80376928212989185, -144.8750000013655779, -4.297418129356379346 ) ) ;
#26704=DIRECTION ( 'NONE',  ( 0.000000000000000000, 0.000000000000000000, 1.000000000000000000 ) ) ;
#26729=AXIS2_PLACEMENT_3D ( 'NONE', #35828, #30988, #11051 ) ;
#26736=CARTESIAN_POINT ( 'NONE',  ( -55.00000000000001421, -135.0000000000000284, 8.082903768654762899 ) ) ;
#26747=CARTESIAN_POINT ( 'NONE',  ( -51.60603307380591787, -135.1875000013656063, -2.891590998281053704 ) ) ;
#26754=ORIENTED_EDGE ( 'NONE', *, *, #45704, .T. ) ;
#26788=CARTESIAN_POINT ( 'NONE',  ( -59.59170313451811296, -141.7500000013656063, 1.485763867205729394 ) ) ;
#26814=CARTESIAN_POINT ( 'NONE',  ( -59.98410592259440222, -139.1250000000000284, -0.3983568153799752487 ) ) ;
#26822=CARTESIAN_POINT ( 'NONE',  ( -50.70258187064364108, -145.3750000013656347, 2.196230717870141014 ) ) ;
#26831=DIRECTION ( 'NONE',  ( -1.000000000000000000, 0.000000000000000000, -0.000000000000000000 ) ) ;
#26839=CARTESIAN_POINT ( 'NONE',  ( -60.14911071818854538, -126.0625000000000284, 1.666127454062681368 ) ) ;
#26847=CARTESIAN_POINT ( 'NONE',  ( -52.80376928212989185, -148.8750000013655779, -4.297418129356379346 ) ) ;
#26854=CARTESIAN_POINT ( 'NONE',  ( -51.75738570946856498, -137.7500000000000000, 3.805975901505576964 ) ) ;
#26866=ORIENTED_EDGE ( 'NONE', *, *, #21949, .F. ) ;
#26871=CARTESIAN_POINT ( 'NONE',  ( -50.55543936806279248, -151.3125000013656063, 0.3552334253322060320 ) ) ;
#26908=CARTESIAN_POINT ( 'NONE',  ( -53.33387254593733928, -135.8125000000000000, 5.149110718188519620 ) ) ;
#26919=CARTESIAN_POINT ( 'NONE',  ( -52.10840900171896806, -141.4375000013656063, 3.393966926194110556 ) ) ;
#26922=CARTESIAN_POINT ( 'NONE',  ( -49.85088928181150436, -131.6875000027312126, -1.666127454062680702 ) ) ;
#26932=CARTESIAN_POINT ( 'NONE',  ( -58.80597590150559739, -154.0000000000000284, 3.242614290531460330 ) ) ;
#26947=CARTESIAN_POINT ( 'NONE',  ( -56.48576386720575471, -132.7500000013656063, -4.591703134518078322 ) ) ;
#26956=CARTESIAN_POINT ( 'NONE',  ( -52.10840900171896806, -126.4375000013656063, 3.393966926194110556 ) ) ;
#26962=CARTESIAN_POINT ( 'NONE',  ( -58.24261429053147765, -135.2500000000000284, -3.805975901505573855 ) ) ;
#26980=CARTESIAN_POINT ( 'NONE',  ( -59.59170313451810586, -140.5000000013655779, 1.485763867205729394 ) ) ;
#26985=CARTESIAN_POINT ( 'NONE',  ( -58.80597590150559739, -150.0000000000000284, 3.242614290531460330 ) ) ;
#26994=CARTESIAN_POINT ( 'NONE',  ( -58.24261429053147765, -144.3750000027312126, -3.805975901505573855 ) ) ;
#27001=CARTESIAN_POINT ( 'NONE',  ( -51.60603307380591787, -138.9375000013656063, -2.891590998281053704 ) ) ;
#27017=CARTESIAN_POINT ( 'NONE',  ( -52.10840900171896806, -147.1875000013656063, 3.393966926194110556 ) ) ;
#27032=CARTESIAN_POINT ( 'NONE',  ( -59.81910112700025905, -152.3125000027312126, -2.462841084822604110 ) ) ;
#27060=CARTESIAN_POINT ( 'NONE',  ( -59.44456063193725015, -136.8125000013656063, -0.3552334253322034230 ) ) ;
#27076=CARTESIAN_POINT ( 'NONE',  ( -50.01589407740564042, -148.7500000027312126, 0.3983568153799778022 ) ) ;
#27086=EDGE_CURVE ( 'NONE', #55783, #28080, #40128, .T. ) ;
#27104=CARTESIAN_POINT ( 'NONE',  ( -54.64476657466781973, -140.0625000013656063, -4.444560631937228834 ) ) ;
#27129=CARTESIAN_POINT ( 'NONE',  ( -59.81910112700027327, -139.1874999999999716, -2.462841084822392279 ) ) ;
#27136=CARTESIAN_POINT ( 'NONE',  ( -50.40829686548195099, -148.2500000013656063, -1.485763867205728284 ) ) ;
#27156=CARTESIAN_POINT ( 'NONE',  ( -52.10840900171896806, -148.1875000013656063, 3.393966926194110556 ) ) ;
#27181=CARTESIAN_POINT ( 'NONE',  ( -55.35523342533222291, -152.5625000013656063, 4.444560631937231499 ) ) ;
#27192=CARTESIAN_POINT ( 'NONE',  ( -51.75738570946856498, -152.7500000000000284, 3.805975901505576964 ) ) ;
#27197=CARTESIAN_POINT ( 'NONE',  ( -56.66612745406274598, -152.3125000000000284, -5.149110718188520508 ) ) ;
#27218=CARTESIAN_POINT ( 'NONE',  ( -52.53715891517739323, -136.4375000000000000, -4.819101127000233298 ) ) ;
#27225=CARTESIAN_POINT ( 'NONE',  ( -55.00000000000002132, -155.0000000000000284, 1.734723475976807094E-15 ) ) ;
#27226=CARTESIAN_POINT ( 'NONE',  ( -57.19623071787016499, -143.6250000013655779, 4.297418129356382899 ) ) ;
#27228=CARTESIAN_POINT ( 'NONE',  ( -57.46284108482265651, -130.0625000027311842, 4.819101127000239515 ) ) ;
#27241=CARTESIAN_POINT ( 'NONE',  ( -56.48576386720575471, -125.7500000013656347, -4.591703134518078322 ) ) ;
#27252=CARTESIAN_POINT ( 'NONE',  ( -52.80376928212989185, -133.8750000013656063, -4.297418129356379346 ) ) ;
#27256=( BOUNDED_CURVE ( )  B_SPLINE_CURVE ( 2, ( #31578, #53868, #44210, #54186, #31252, #41215, #60548, #19456, #51212 ),
 .UNSPECIFIED., .F., .F. ) 
 B_SPLINE_CURVE_WITH_KNOTS ( ( 3, 2, 2, 2, 3 ),
 ( 0.1750000000000001554, 0.1791666666666668351, 0.1833333333333334869, 0.1875000000000001665, 0.1916666666666668462 ),
 .UNSPECIFIED. ) 
 CURVE ( )  GEOMETRIC_REPRESENTATION_ITEM ( )  RATIONAL_B_SPLINE_CURVE ( ( 0.9999999999999970024, 0.9238795325112897361, 1.000000000000000000, 0.9238795325112867385, 1.000000000000000000, 0.9238795325112867385, 1.000000000000000000, 0.9238795325112837409, 1.000000000000003109 ) ) 
 REPRESENTATION_ITEM ( '' )  );
#27264=CARTESIAN_POINT ( 'NONE',  ( -57.89159099828107458, -126.9375000013656063, -3.393966926194107447 ) ) ;
#27289=DIRECTION ( 'NONE',  ( -0.8660254037844387076, 0.000000000000000000, 0.4999999999999998890 ) ) ;
#27293=CARTESIAN_POINT ( 'NONE',  ( -50.70258187064364108, -139.1250000013656063, 2.196230717870141014 ) ) ;
#27298=CARTESIAN_POINT ( 'NONE',  ( -54.60164318462004474, -149.3750000000000284, -4.984105922594373794 ) ) ;
#27301=( NAMED_UNIT ( * ) PLANE_ANGLE_UNIT ( ) SI_UNIT ( $, .RADIAN. ) );
#27306=CARTESIAN_POINT ( 'NONE',  ( -50.40829686548195099, -153.2500000013656063, -1.485763867205728284 ) ) ;
#27307=CARTESIAN_POINT ( 'NONE',  ( -58.80597590150559739, -142.1250000027312126, 3.242614290531460330 ) ) ;
#27308=( BOUNDED_CURVE ( )  B_SPLINE_CURVE ( 2, ( #10692, #30302, #50248, #24534, #1389 ),
 .UNSPECIFIED., .F., .F. ) 
 B_SPLINE_CURVE_WITH_KNOTS ( ( 3, 2, 3 ),
 ( 0.000000000000000000, 0.004166666666666670078, 0.008333333333333340157 ),
 .UNSPECIFIED. ) 
 CURVE ( )  GEOMETRIC_REPRESENTATION_ITEM ( )  RATIONAL_B_SPLINE_CURVE ( ( 1.000000000000000000, 0.9238795325112867385, 1.000000000000000000, 0.9238795325112866275, 1.000000000000000222 ) ) 
 REPRESENTATION_ITEM ( '' )  );
#27315=CARTESIAN_POINT ( 'NONE',  ( -52.10840900171896806, -136.1875000013656063, 3.393966926194110556 ) ) ;
#27329=CARTESIAN_POINT ( 'NONE',  ( -51.60603307380591787, -145.9375000013656063, -2.891590998281053704 ) ) ;
#27333=CARTESIAN_POINT ( 'NONE',  ( -56.66612745406288099, -141.4375000027311842, -5.149110718188529390 ) ) ;
#27366=CARTESIAN_POINT ( 'NONE',  ( -53.51423613279429503, -129.5000000013656347, 4.591703134518082763 ) ) ;
#27373=VERTEX_POINT ( 'NONE', #7642 ) ;
#27394=CYLINDRICAL_SURFACE ( 'NONE', #9852, 5.000000000000000000 ) ;
#27396=CARTESIAN_POINT ( 'NONE',  ( -54.60164318462004474, -138.3750000000000284, -4.984105922594373794 ) ) ;
#27407=LINE ( 'NONE', #52503, #5877 ) ;
#27411=CARTESIAN_POINT ( 'NONE',  ( -58.39396692619412477, -137.6875000013656063, 2.891590998281057701 ) ) ;
#27418=EDGE_LOOP ( 'NONE', ( #16663, #60086, #15392, #3731 ) ) ;
#27429=CARTESIAN_POINT ( 'NONE',  ( -55.52884467124510337, -135.0324864422690894, -4.515220955086300059 ) ) ;
#27441=CARTESIAN_POINT ( 'NONE',  ( -53.51423613279429503, -142.5000000013656347, 4.591703134518082763 ) ) ;
#27448=FACE_OUTER_BOUND ( 'NONE', #15333, .T. ) ;
#27453=CARTESIAN_POINT ( 'NONE',  ( -56.66612745406270335, -126.3125000000000284, -5.149110718188516067 ) ) ;
#27464=CARTESIAN_POINT ( 'NONE',  ( -50.55543936806279248, -147.0625000013656063, 0.3552334253322060320 ) ) ;
#27465=CARTESIAN_POINT ( 'NONE',  ( -58.24261429053147765, -150.3750000027312126, -3.805975901505573855 ) ) ;
#27476=CARTESIAN_POINT ( 'NONE',  ( -58.24261429053147765, -140.3750000027312126, -3.805975901505573855 ) ) ;
#27488=CARTESIAN_POINT ( 'NONE',  ( -50.70258187064364108, -150.3750000013656063, 2.196230717870141014 ) ) ;
#27500=CARTESIAN_POINT ( 'NONE',  ( -60.14911071818854538, -153.0625000000000284, 1.666127454062681146 ) ) ;
#27525=DIRECTION ( 'NONE',  ( 0.000000000000000000, 1.000000000000000000, 0.000000000000000000 ) ) ;
#27528=CARTESIAN_POINT ( 'NONE',  ( -51.19402409849444524, -137.5000000000000284, -3.242614290531456334 ) ) ;
#27530=ORIENTED_EDGE ( 'NONE', *, *, #62972, .F. ) ;
#27537=CARTESIAN_POINT ( 'NONE',  ( -55.35523342533222291, -137.5625000013656063, 4.444560631937231499 ) ) ;
#27539=CARTESIAN_POINT ( 'NONE',  ( -55.39835681537999790, -131.0000000027312126, 4.984105922594378235 ) ) ;
#27562=CARTESIAN_POINT ( 'NONE',  ( -59.29741812935640155, -134.6250000013656347, -2.196230717870135685 ) ) ;
#27572=CARTESIAN_POINT ( 'NONE',  ( -50.40829686548195099, -128.2500000013656063, -1.485763867205728284 ) ) ;
#27602=CARTESIAN_POINT ( 'NONE',  ( -55.35523342533222291, -138.3125000013656063, 4.444560631937231499 ) ) ;
#27608=CARTESIAN_POINT ( 'NONE',  ( -59.98410592259440222, -148.1250000000000284, -0.3983568153799752487 ) ) ;
#27617=VERTEX_POINT ( 'NONE', #10786 ) ;
#27619=CARTESIAN_POINT ( 'NONE',  ( -50.55543936806279248, -151.3125000013656063, 0.3552334253322060320 ) ) ;
#27620=CARTESIAN_POINT ( 'NONE',  ( -57.46284108482265651, -144.0625000027312126, 4.819101127000239515 ) ) ;
#27629=CARTESIAN_POINT ( 'NONE',  ( -59.29741812935640155, -138.6250000013655779, -2.196230717870135685 ) ) ;
#27645=CARTESIAN_POINT ( 'NONE',  ( -53.51423613279429503, -146.2500000013656063, 4.591703134518082763 ) ) ;
#27648=CARTESIAN_POINT ( 'NONE',  ( -49.85088928181150436, -141.6875000027311842, -1.666127454062680480 ) ) ;
#27688=CARTESIAN_POINT ( 'NONE',  ( -50.40829686548195099, -131.2500000013656347, -1.485763867205728284 ) ) ;
#27729=CARTESIAN_POINT ( 'NONE',  ( -59.44456063193725015, -135.8125000013656063, -0.3552334253322034230 ) ) ;
#27750=FACE_OUTER_BOUND ( 'NONE', #45875, .T. ) ;
#27759=CARTESIAN_POINT ( 'NONE',  ( -57.19623071787017210, -142.6250000013655779, 4.297418129356382899 ) ) ;
#27769=VECTOR ( 'NONE', #59769, 1000.000000000000000 ) ;
#27779=CARTESIAN_POINT ( 'NONE',  ( -53.51423613279429503, -148.2500000013656063, 4.591703134518082763 ) ) ;
#27804=CARTESIAN_POINT ( 'NONE',  ( -55.35523342533222291, -148.5625000013656063, 4.444560631937231499 ) ) ;
#27841=CARTESIAN_POINT ( 'NONE',  ( -53.33387254593733928, -136.8125000000000284, 5.149110718188519620 ) ) ;
#27850=CARTESIAN_POINT ( 'NONE',  ( -57.89159099828107458, -138.9375000013656063, -3.393966926194107447 ) ) ;
#27852=CARTESIAN_POINT ( 'NONE',  ( -57.46284108482265651, -129.0625000027312126, 4.819101127000239515 ) ) ;
#27866=CARTESIAN_POINT ( 'NONE',  ( -59.44456063193725015, -126.5625000013655921, -0.3552334253322034230 ) ) ;
#27875=ADVANCED_FACE ( 'NONE', ( #31037 ), #26216, .T. ) ;
#27878=CARTESIAN_POINT ( 'NONE',  ( -52.80376928212989185, -129.8750000013656063, -4.297418129356379346 ) ) ;
#27888=CARTESIAN_POINT ( 'NONE',  ( -52.10840900171896806, -128.4375000013656063, 3.393966926194110556 ) ) ;
#27913=VERTEX_POINT ( 'NONE', #46159 ) ;
#27920=CARTESIAN_POINT ( 'NONE',  ( -53.33387254593733928, -149.8124999999999716, 5.149110718188519620 ) ) ;
#27921=EDGE_CURVE ( 'NONE', #21128, #27373, #33598, .T. ) ;
#27929=ORIENTED_EDGE ( 'NONE', *, *, #53609, .T. ) ;
#27930=CARTESIAN_POINT ( 'NONE',  ( -57.89159099828107458, -151.9375000013656063, -3.393966926194107447 ) ) ;
#27931=CARTESIAN_POINT ( 'NONE',  ( -49.85088928181150436, -140.6875000027312410, -1.666127454062680702 ) ) ;
#27938=CARTESIAN_POINT ( 'NONE',  ( -58.39396692619412477, -135.4375000013656063, 2.891590998281057701 ) ) ;
#27954=CARTESIAN_POINT ( 'NONE',  ( -59.44456063193725015, -144.5625000013656063, -0.3552334253322034230 ) ) ;
#27956=EDGE_CURVE ( 'NONE', #11458, #44963, #53503, .T. ) ;
#27999=CARTESIAN_POINT ( 'NONE',  ( -52.10840900171896806, -129.4375000013656063, 3.393966926194110556 ) ) ;
#28007=CARTESIAN_POINT ( 'NONE',  ( -55.39835681537999790, -153.0000000027312410, 4.984105922594378235 ) ) ;
#28044=CARTESIAN_POINT ( 'NONE',  ( -53.51423613279429503, -134.5000000013656063, 4.591703134518082763 ) ) ;
#28045=DIRECTION ( 'NONE',  ( 0.000000000000000000, 1.000000000000000000, 0.000000000000000000 ) ) ;
#28051=EDGE_CURVE ( 'NONE', #34010, #27913, #57844, .T. ) ;
#28058=( BOUNDED_CURVE ( )  B_SPLINE_CURVE ( 2, ( #9747, #10071, #29045, #764, #63485, #48670, #5900, #1090, #44160 ),
 .UNSPECIFIED., .F., .F. ) 
 B_SPLINE_CURVE_WITH_KNOTS ( ( 3, 2, 2, 2, 3 ),
 ( 0.008333333333333340157, 0.01250000000000001110, 0.01666666666666668031, 0.02083333333333334952, 0.02500000000000002220 ),
 .UNSPECIFIED. ) 
 CURVE ( )  GEOMETRIC_REPRESENTATION_ITEM ( )  RATIONAL_B_SPLINE_CURVE ( ( 0.9999999999999998890, 0.9238795325112868495, 1.000000000000000000, 0.9238795325112867385, 1.000000000000000000, 0.9238795325112867385, 1.000000000000000000, 0.9238795325112864054, 1.000000000000000444 ) ) 
 REPRESENTATION_ITEM ( '' )  );
#28068=DIRECTION ( 'NONE',  ( 0.000000000000000000, 1.000000000000000000, 0.000000000000000000 ) ) ;
#28077=CARTESIAN_POINT ( 'NONE',  ( -59.59170313451811296, -144.7500000013656063, 1.485763867205729394 ) ) ;
#28080=VERTEX_POINT ( 'NONE', #8814 ) ;
#28094=CARTESIAN_POINT ( 'NONE',  ( -51.60603307380591787, -144.9375000013656063, -2.891590998281053704 ) ) ;
#28116=ORIENTED_EDGE ( 'NONE', *, *, #22896, .F. ) ;
#28120=CARTESIAN_POINT ( 'NONE',  ( -59.59170313451811296, -148.7500000013655779, 1.485763867205729394 ) ) ;
#28126=CARTESIAN_POINT ( 'NONE',  ( -55.39835681537999790, -136.0000000027312126, 4.984105922594378235 ) ) ;
#28158=CARTESIAN_POINT ( 'NONE',  ( -52.53715891517739323, -138.4375000000000000, -4.819101127000233298 ) ) ;
#28166=CARTESIAN_POINT ( 'NONE',  ( -53.51423613279429503, -138.5000000013656063, 4.591703134518083651 ) ) ;
#28168=CARTESIAN_POINT ( 'NONE',  ( -60.14911071818854538, -128.1875000027312410, 1.666127454062681368 ) ) ;
#28172=CARTESIAN_POINT ( 'NONE',  ( -53.33387254593728954, -150.9375000027311842, 5.149110718188522284 ) ) ;
#28179=CARTESIAN_POINT ( 'NONE',  ( -50.70258187064364108, -125.1250000013656205, 2.196230717870141014 ) ) ;
#28191=CARTESIAN_POINT ( 'NONE',  ( -51.60603307380591787, -129.9375000013656063, -2.891590998281053704 ) ) ;
#28198=CARTESIAN_POINT ( 'NONE',  ( -55.39835672516371545, -134.9999999999999716, 4.984105929804953483 ) ) ;
#28199=ORIENTED_EDGE ( 'NONE', *, *, #57550, .F. ) ;
#28208=DIRECTION ( 'NONE',  ( 0.000000000000000000, 1.000000000000000000, 0.000000000000000000 ) ) ;
#28223=CARTESIAN_POINT ( 'NONE',  ( -54.64476657466781973, -150.0625000013656063, -4.444560631937228834 ) ) ;
#28227=CARTESIAN_POINT ( 'NONE',  ( -57.89159099828107458, -136.6875000013656063, -3.393966926194107447 ) ) ;
#28233=CARTESIAN_POINT ( 'NONE',  ( -50.18089887299979068, -149.6875000000000284, 2.462841084822635640 ) ) ;
#28244=CARTESIAN_POINT ( 'NONE',  ( -54.64476657466781973, -150.0625000013656063, -4.444560631937228834 ) ) ;
#28245=CARTESIAN_POINT ( 'NONE',  ( -57.46284108482265651, -143.0625000027312126, 4.819101127000239515 ) ) ;
#28253=CARTESIAN_POINT ( 'NONE',  ( -58.24261429053147765, -139.3750000027312126, -3.805975901505573855 ) ) ;
#28254=CARTESIAN_POINT ( 'NONE',  ( -54.64476657466781973, -135.8125000013656063, -4.444560631937228834 ) ) ;
#28269=CARTESIAN_POINT ( 'NONE',  ( -57.89159099828107458, -141.6875000013656063, -3.393966926194107447 ) ) ;
#28273=CARTESIAN_POINT ( 'NONE',  ( -54.60164318462004474, -144.3750000000000284, -4.984105922594373794 ) ) ;
#28303=VERTEX_POINT ( 'NONE', #10068 ) ;
#28307=CARTESIAN_POINT ( 'NONE',  ( -56.66612745406278151, -149.4375000027312410, -5.149110718188523173 ) ) ;
#28310=CARTESIAN_POINT ( 'NONE',  ( -50.70258187064364108, -130.3750000013656631, 2.196230717870141014 ) ) ;
#28320=ORIENTED_EDGE ( 'NONE', *, *, #36538, .T. ) ;
#28327=( BOUNDED_CURVE ( )  B_SPLINE_CURVE ( 2, ( #47721, #62847, #34184, #18761, #48037, #38386, #24223, #19070, #62541 ),
 .UNSPECIFIED., .F., .F. ) 
 B_SPLINE_CURVE_WITH_KNOTS ( ( 3, 2, 2, 2, 3 ),
 ( 0.4250000000000003220, 0.4291666666666669738, 0.4333333333333336812, 0.4375000000000003886, 0.4416666666666670404 ),
 .UNSPECIFIED. ) 
 CURVE ( )  GEOMETRIC_REPRESENTATION_ITEM ( )  RATIONAL_B_SPLINE_CURVE ( ( 0.9999999999999938938, 0.9238795325112928447, 1.000000000000000000, 0.9238795325112867385, 1.000000000000000000, 0.9238795325112867385, 1.000000000000000000, 0.9238795325112796331, 1.000000000000007105 ) ) 
 REPRESENTATION_ITEM ( '' )  );
#28331=CARTESIAN_POINT ( 'NONE',  ( -55.00000000000002132, -155.0000000000000284, 1.734723475976807094E-15 ) ) ;
#28341=CARTESIAN_POINT ( 'NONE',  ( -57.19623071787017210, -152.3750000013656063, 4.297418129356382899 ) ) ;
#28354=CARTESIAN_POINT ( 'NONE',  ( -59.44456063193725015, -137.8125000013656063, -0.3552334253322034230 ) ) ;
#28375=CARTESIAN_POINT ( 'NONE',  ( -59.81910112700026616, -144.3125000027311842, -2.462841084822481541 ) ) ;
#28387=CARTESIAN_POINT ( 'NONE',  ( -57.19623071787017210, -144.6250000013656063, 4.297418129356382899 ) ) ;
#28407=CARTESIAN_POINT ( 'NONE',  ( -59.44456063193725015, -143.5625000013656063, -0.3552334253322034230 ) ) ;
#28424=DIRECTION ( 'NONE',  ( -0.6485228581062915110, 0.000000000000000000, -0.7611951803011149931 ) ) ;
#28437=CARTESIAN_POINT ( 'NONE',  ( -59.29741812935640155, -149.8750000013655779, -2.196230717870135685 ) ) ;
#28475=CARTESIAN_POINT ( 'NONE',  ( -55.39835681537999790, -132.8750000000000284, 4.984105922594378235 ) ) ;
#28482=CARTESIAN_POINT ( 'NONE',  ( -58.39396692619412477, -138.6875000013656347, 2.891590998281057701 ) ) ;
#28484=CARTESIAN_POINT ( 'NONE',  ( -58.24261429053147765, -127.3750000027312268, -3.805975901505573855 ) ) ;
#28508=CARTESIAN_POINT ( 'NONE',  ( -53.51423613279429503, -130.2500000013656063, 4.591703134518082763 ) ) ;
#28509=CARTESIAN_POINT ( 'NONE',  ( -50.70258187064364108, -147.1250000013656063, 2.196230717870141014 ) ) ;
#28519=UNCERTAINTY_MEASURE_WITH_UNIT (LENGTH_MEASURE( 1.000000000000000082E-05 ), #41093, 'distance_accuracy_value', 'NONE');
#28540=CARTESIAN_POINT ( 'NONE',  ( -50.70258187064364108, -149.3750000013656347, 2.196230717870141014 ) ) ;
#28544=CARTESIAN_POINT ( 'NONE',  ( -57.19623071787016499, -135.3750000013656063, 4.297418129356382899 ) ) ;
#28550=CARTESIAN_POINT ( 'NONE',  ( -57.46284108482265651, -144.9375000000000000, 4.819101127000239515 ) ) ;
#28558=CARTESIAN_POINT ( 'NONE',  ( -50.55543936806279248, -150.3125000013656063, 0.3552334253322060320 ) ) ;
#28559=CARTESIAN_POINT ( 'NONE',  ( -58.80597590150559739, -137.1250000027312410, 3.242614290531460330 ) ) ;
#28561=DIRECTION ( 'NONE',  ( 0.000000000000000000, 0.000000000000000000, -1.000000000000000000 ) ) ;
#28566=CARTESIAN_POINT ( 'NONE',  ( -51.75738570946856498, -139.8750000027312126, 3.805975901505576964 ) ) ;
#28567=CARTESIAN_POINT ( 'NONE',  ( -58.39396692619412477, -131.4375000013656063, 2.891590998281057701 ) ) ;
#28583=CARTESIAN_POINT ( 'NONE',  ( -50.40829686548195099, -141.0000000013656063, -1.485763867205728284 ) ) ;
#28587=DIRECTION ( 'NONE',  ( 0.6592143633790508161, -0.4999999999999791833, -0.5616372700549471242 ) ) ;
#28625=CARTESIAN_POINT ( 'NONE',  ( -57.19623071787017210, -128.6250000013656347, 4.297418129356382899 ) ) ;
#28628=LINE ( 'NONE', #28937, #18287 ) ;
#28633=CARTESIAN_POINT ( 'NONE',  ( -55.39835681537999790, -151.8750000000000284, 4.984105922594378235 ) ) ;
#28634=CARTESIAN_POINT ( 'NONE',  ( -51.19402409849444524, -152.6250000027312126, -3.242614290531456334 ) ) ;
#28637=VECTOR ( 'NONE', #56429, 1000.000000000000000 ) ;
#28652=CARTESIAN_POINT ( 'NONE',  ( -58.80597590150559739, -154.1250000027312126, 3.242614290531460330 ) ) ;
#28654=CARTESIAN_POINT ( 'NONE',  ( -57.19623071787017210, -154.3750000013656063, 4.297418129356382899 ) ) ;
#28668=CARTESIAN_POINT ( 'NONE',  ( -50.40829686548195099, -134.2500000013656063, -1.485763867205728284 ) ) ;
#28674=CARTESIAN_POINT ( 'NONE',  ( -58.24261429053147765, -140.2500000000000000, -3.805975901505573855 ) ) ;
#28675=CARTESIAN_POINT ( 'NONE',  ( -57.61805966450963012, -135.0000000000000000, -3.717333593771256606 ) ) ;
#28684=CARTESIAN_POINT ( 'NONE',  ( -55.00000000000001421, -155.0000000000000284, 8.082903768654762899 ) ) ;
#28688=CARTESIAN_POINT ( 'NONE',  ( -58.24261429053147765, -147.3750000027312126, -3.805975901505573855 ) ) ;
#28698=CARTESIAN_POINT ( 'NONE',  ( -54.64476657466781973, -142.0625000013656063, -4.444560631937228834 ) ) ;
#28712=VERTEX_POINT ( 'NONE', #28973 ) ;
#28715=CARTESIAN_POINT ( 'NONE',  ( -56.48576386720575471, -145.7500000013655779, -4.591703134518078322 ) ) ;
#28718=STYLED_ITEM ( 'NONE', ( #1933 ), #60912 ) ;
#28739=CARTESIAN_POINT ( 'NONE',  ( -52.10840900171896806, -148.4375000013656063, 3.393966926194110556 ) ) ;
#28766=ADVANCED_FACE ( 'NONE', ( #29280 ), #26306, .F. ) ;
#28784=PRODUCT_DEFINITION_CONTEXT ( 'detailed design', #5591, 'design' ) ;
#28786=CARTESIAN_POINT ( 'NONE',  ( -57.46284108482265651, -131.9375000000000000, 4.819101127000239515 ) ) ;
#28795=CARTESIAN_POINT ( 'NONE',  ( -50.18089887299979068, -125.8125000027312268, 2.462841084822635640 ) ) ;
#28798=( BOUNDED_CURVE ( )  B_SPLINE_CURVE ( 2, ( #62225, #18143, #37771, #16647, #47726, #51063, #46233, #16967, #60725 ),
 .UNSPECIFIED., .F., .F. ) 
 B_SPLINE_CURVE_WITH_KNOTS ( ( 3, 2, 2, 2, 3 ),
 ( 0.5083333333333337478, 0.5125000000000003997, 0.5166666666666671626, 0.5208333333333338144, 0.5250000000000004663 ),
 .UNSPECIFIED. ) 
 CURVE ( )  GEOMETRIC_REPRESENTATION_ITEM ( )  RATIONAL_B_SPLINE_CURVE ( ( 0.9999999999999918954, 0.9238795325112948431, 1.000000000000000000, 0.9238795325112867385, 1.000000000000000000, 0.9238795325112867385, 1.000000000000000000, 0.9238795325112786339, 1.000000000000008216 ) ) 
 REPRESENTATION_ITEM ( '' )  );
#28816=MANIFOLD_SOLID_BREP ( 'Cavity1', #5842 ) ;
#28819=CARTESIAN_POINT ( 'NONE',  ( -58.39396692619412477, -130.4375000013656063, 2.891590998281057701 ) ) ;
#28820=CARTESIAN_POINT ( 'NONE',  ( -56.48576386720575471, -147.7500000013656063, -4.591703134518078322 ) ) ;
#28853=CARTESIAN_POINT ( 'NONE',  ( -54.64476657466781973, -153.0625000013656063, -4.444560631937228834 ) ) ;
#28861=ORIENTED_EDGE ( 'NONE', *, *, #42941, .T. ) ;
#28863=CARTESIAN_POINT ( 'NONE',  ( -53.33387254593733928, -146.8125000000000284, 5.149110718188519620 ) ) ;
#28866=ORIENTED_EDGE ( 'NONE', *, *, #45252, .F. ) ;
#28870=CARTESIAN_POINT ( 'NONE',  ( -59.98410592259440222, -135.2500000027312126, -0.3983568153799752487 ) ) ;
#28872=CARTESIAN_POINT ( 'NONE',  ( -59.44456063193725015, -150.8125000013656063, -0.3552334253322034230 ) ) ;
#28873=CARTESIAN_POINT ( 'NONE',  ( -52.53715891517739323, -140.5625000027311842, -4.819101127000233298 ) ) ;
#28882=CARTESIAN_POINT ( 'NONE',  ( -52.10840900171896806, -131.1875000013656063, 3.393966926194110556 ) ) ;
#28897=CARTESIAN_POINT ( 'NONE',  ( -59.29741812935640155, -141.6250000013656063, -2.196230717870135685 ) ) ;
#28917=CARTESIAN_POINT ( 'NONE',  ( -51.75738570946856498, -155.0000000000000284, 3.805975901505577408 ) ) ;
#28928=CARTESIAN_POINT ( 'NONE',  ( -50.70258187064364108, -152.1250000013656063, 2.196230717870141014 ) ) ;
#28934=CARTESIAN_POINT ( 'NONE',  ( -51.60603307380591787, -129.1875000013656063, -2.891590998281053704 ) ) ;
#28937=CARTESIAN_POINT ( 'NONE',  ( -51.75738570946856498, -155.0000000000000284, 3.805975901505577408 ) ) ;
#28940=CARTESIAN_POINT ( 'NONE',  ( -58.24261429053147765, -155.0000000000000284, -3.805975901505573411 ) ) ;
#28944=CARTESIAN_POINT ( 'NONE',  ( -51.19402409849444524, -150.6250000027312126, -3.242614290531456334 ) ) ;
#28951=CARTESIAN_POINT ( 'NONE',  ( -52.53715891517739323, -150.5625000027311842, -4.819101127000233298 ) ) ;
#28963=CARTESIAN_POINT ( 'NONE',  ( -50.55543936806279248, -152.0625000013656063, 0.3552334253322060320 ) ) ;
#28973=CARTESIAN_POINT ( 'NONE',  ( -51.75738570946856498, -152.7500000000000284, 3.805975901505576964 ) ) ;
#28979=CARTESIAN_POINT ( 'NONE',  ( -52.80376928212989185, -133.1250000013656063, -4.297418129356379346 ) ) ;
#29005=CARTESIAN_POINT ( 'NONE',  ( -51.60603307380591787, -138.1875000013656347, -2.891590998281053704 ) ) ;
#29009=CARTESIAN_POINT ( 'NONE',  ( -59.81910112700027327, -148.3125000027311557, -2.462841084822540605 ) ) ;
#29024=CARTESIAN_POINT ( 'NONE',  ( -52.80376928212989185, -145.8750000013655779, -4.297418129356379346 ) ) ;
#29045=CARTESIAN_POINT ( 'NONE',  ( -50.01589407740564042, -154.6250000000000284, 0.3983568153799778022 ) ) ;
#29049=CARTESIAN_POINT ( 'NONE',  ( -59.29741812935640155, -148.8750000013655779, -2.196230717870135685 ) ) ;
#29084=CARTESIAN_POINT ( 'NONE',  ( -59.98410592259440222, -135.1250000000000284, -0.3983568153799752487 ) ) ;
#29096=CARTESIAN_POINT ( 'NONE',  ( -51.19402409849444524, -128.6250000027312126, -3.242614290531456334 ) ) ;
#29098=CARTESIAN_POINT ( 'NONE',  ( -50.78616202067674834, -135.0000000000000568, 2.038383678880063332 ) ) ;
#29122=CARTESIAN_POINT ( 'NONE',  ( -57.19623071787017210, -129.3750000013656347, 4.297418129356382899 ) ) ;
#29123=CARTESIAN_POINT ( 'NONE',  ( -55.35523342533222291, -147.3125000013656063, 4.444560631937231499 ) ) ;
#29157=CARTESIAN_POINT ( 'NONE',  ( -55.35523342533222291, -151.5625000013656063, 4.444560631937231499 ) ) ;
#29162=CARTESIAN_POINT ( 'NONE',  ( -52.10840900171896806, -136.1875000013656063, 3.393966926194110556 ) ) ;
#29167=ORIENTED_EDGE ( 'NONE', *, *, #56136, .F. ) ;
#29168=CARTESIAN_POINT ( 'NONE',  ( -59.98410592259440222, -147.1250000000000284, -0.3983568153799752487 ) ) ;
#29177=CARTESIAN_POINT ( 'NONE',  ( -50.70258187064364108, -145.3750000013656063, 2.196230717870141014 ) ) ;
#29178=CARTESIAN_POINT ( 'NONE',  ( -59.98410592259440222, -139.2500000027312126, -0.3983568153799752487 ) ) ;
#29184=EDGE_LOOP ( 'NONE', ( #45717, #54656, #48636, #12410 ) ) ;
#29187=CARTESIAN_POINT ( 'NONE',  ( -50.18089887299979068, -153.6875000000000284, 2.462841084822613436 ) ) ;
#29188=CARTESIAN_POINT ( 'NONE',  ( -50.70258187064364108, -132.1250000013656347, 2.196230717870141014 ) ) ;
#29204=CARTESIAN_POINT ( 'NONE',  ( -59.59170313451811296, -141.5000000013656063, 1.485763867205729394 ) ) ;
#29222=VERTEX_POINT ( 'NONE', #28198 ) ;
#29244=CARTESIAN_POINT ( 'NONE',  ( -57.89159099828107458, -128.9375000013656063, -3.393966926194107447 ) ) ;
#29255=CARTESIAN_POINT ( 'NONE',  ( -55.39835681537999790, -149.0000000027312126, 4.984105922594378235 ) ) ;
#29280=FACE_OUTER_BOUND ( 'NONE', #51562, .T. ) ;
#29306=CARTESIAN_POINT ( 'NONE',  ( -51.75738570946856498, -136.7500000000000284, 3.805975901505576964 ) ) ;
#29312=CARTESIAN_POINT ( 'NONE',  ( -50.40829686548195099, -140.2500000013656063, -1.485763867205728284 ) ) ;
#29316=EDGE_LOOP ( 'NONE', ( #10993, #10112, #14300, #11626 ) ) ;
#29331=CARTESIAN_POINT ( 'NONE',  ( -57.89159099828107458, -145.6875000013656063, -3.393966926194107447 ) ) ;
#29357=CARTESIAN_POINT ( 'NONE',  ( -50.40829686548195099, -142.2500000013656063, -1.485763867205728284 ) ) ;
#29396=CARTESIAN_POINT ( 'NONE',  ( -58.24261429053147765, -133.2500000000000284, -3.805975901505573855 ) ) ;
#29406=CARTESIAN_POINT ( 'NONE',  ( -52.53715891517739323, -126.5625000027312268, -4.819101127000233298 ) ) ;
#29431=CARTESIAN_POINT ( 'NONE',  ( -55.35523342533222291, -125.3125000013655921, 4.444560631937231499 ) ) ;
#29433=CARTESIAN_POINT ( 'NONE',  ( -55.35523342533222291, -146.3125000013656063, 4.444560631937231499 ) ) ;
#29445=CARTESIAN_POINT ( 'NONE',  ( -50.70258187064364108, -125.3750000013656205, 2.196230717870141014 ) ) ;
#29468=CARTESIAN_POINT ( 'NONE',  ( -54.64476657466781973, -151.0625000013656063, -4.444560631937228834 ) ) ;
#29479=CARTESIAN_POINT ( 'NONE',  ( -58.24261429053147765, -144.2500000000000284, -3.805975901505573855 ) ) ;
#29486=CARTESIAN_POINT ( 'NONE',  ( -59.44456063193725015, -145.8125000013656063, -0.3552334253322034230 ) ) ;
#29487=CARTESIAN_POINT ( 'NONE',  ( -49.85088928181150436, -138.6875000027312126, -1.666127454062680702 ) ) ;
#29498=ORIENTED_EDGE ( 'NONE', *, *, #22562, .T. ) ;
#29503=CARTESIAN_POINT ( 'NONE',  ( -52.10840900171896806, -134.1875000013656063, 3.393966926194110556 ) ) ;
#29518=CARTESIAN_POINT ( 'NONE',  ( -59.29741812935640155, -142.6250000013655779, -2.196230717870135685 ) ) ;
#29531=LINE ( 'NONE', #44984, #4045 ) ;
#29542=( BOUNDED_CURVE ( )  B_SPLINE_CURVE ( 2, ( #21561, #60169, #30554, #16730, #41158, #36346, #30230, #20609, #30882 ),
 .UNSPECIFIED., .F., .F. ) 
 B_SPLINE_CURVE_WITH_KNOTS ( ( 3, 2, 2, 2, 3 ),
 ( 0.5583333333333337922, 0.5625000000000004441, 0.5666666666666670960, 0.5708333333333338588, 0.5750000000000005107 ),
 .UNSPECIFIED. ) 
 CURVE ( )  GEOMETRIC_REPRESENTATION_ITEM ( )  RATIONAL_B_SPLINE_CURVE ( ( 0.9999999999999918954, 0.9238795325112948431, 1.000000000000000000, 0.9238795325112867385, 1.000000000000000000, 0.9238795325112867385, 1.000000000000000000, 0.9238795325112766355, 1.000000000000010214 ) ) 
 REPRESENTATION_ITEM ( '' )  );
#29556=CARTESIAN_POINT ( 'NONE',  ( -54.64476657466781973, -153.8125000013656347, -4.444560631937228834 ) ) ;
#29566=CARTESIAN_POINT ( 'NONE',  ( -59.44456063193725015, -128.8125000013656063, -0.3552334253322034230 ) ) ;
#29576=CARTESIAN_POINT ( 'NONE',  ( -58.80597590150559739, -149.1250000027312126, 3.242614290531460330 ) ) ;
#29595=CARTESIAN_POINT ( 'NONE',  ( -50.55543936806279248, -153.0625000013656063, 0.3552334253322060320 ) ) ;
#29620=CARTESIAN_POINT ( 'NONE',  ( -59.70202243701069023, -135.0000000000000853, 1.323094887694161281 ) ) ;
#29624=CARTESIAN_POINT ( 'NONE',  ( -51.75738570946856498, -155.0000000000000284, 3.805975901505577408 ) ) ;
#29644=CARTESIAN_POINT ( 'NONE',  ( -53.51423613279429503, -140.5000000013656347, 4.591703134518082763 ) ) ;
#29654=EDGE_LOOP ( 'NONE', ( #34968, #9857, #49736, #61282 ) ) ;
#29660=CARTESIAN_POINT ( 'NONE',  ( -51.75738570946856498, -136.8750000027312126, 3.805975901505576964 ) ) ;
#29663=CARTESIAN_POINT ( 'NONE',  ( -50.70258187064364108, -140.1250000013655779, 2.196230717870141014 ) ) ;
#29687=CARTESIAN_POINT ( 'NONE',  ( -58.39396692619412477, -143.6875000013656063, 2.891590998281057701 ) ) ;
#29693=LINE ( 'NONE', #53827, #49259 ) ;
#29696=ORIENTED_EDGE ( 'NONE', *, *, #13810, .F. ) ;
#29717=VERTEX_POINT ( 'NONE', #61611 ) ;
#29724=CARTESIAN_POINT ( 'NONE',  ( -60.14911071818854538, -131.0625000000000284, 1.666127454062681368 ) ) ;
#29734=CARTESIAN_POINT ( 'NONE',  ( -59.44456063193725015, -153.5625000013656063, -0.3552334253322034230 ) ) ;
#29739=CARTESIAN_POINT ( 'NONE',  ( -51.75738570946856498, -155.0000000000000284, 3.805975901505577408 ) ) ;
#29758=CARTESIAN_POINT ( 'NONE',  ( -54.64476657466781973, -125.8125000013655921, -4.444560631937228834 ) ) ;
#29759=CARTESIAN_POINT ( 'NONE',  ( -50.55543936806279248, -148.0625000013656063, 0.3552334253322060320 ) ) ;
#29790=CARTESIAN_POINT ( 'NONE',  ( -58.39396692619412477, -147.6875000013656063, 2.891590998281057701 ) ) ;
#29801=CARTESIAN_POINT ( 'NONE',  ( -55.39835681537999790, -144.8750000000000284, 4.984105922594378235 ) ) ;
#29811=CARTESIAN_POINT ( 'NONE',  ( -57.19623071787016499, -147.6250000013655779, 4.297418129356382899 ) ) ;
#29814=CARTESIAN_POINT ( 'NONE',  ( -60.14911071818854538, -137.1875000027312126, 1.666127454062681368 ) ) ;
#29822=( BOUNDED_CURVE ( )  B_SPLINE_CURVE ( 2, ( #55055, #10979, #60208, #6170, #25787, #1364, #16451, #37332, #8389 ),
 .UNSPECIFIED., .F., .F. ) 
 B_SPLINE_CURVE_WITH_KNOTS ( ( 3, 2, 2, 2, 3 ),
 ( 0.4250000000000003220, 0.4291666666666669738, 0.4333333333333336812, 0.4375000000000003886, 0.4416666666666670404 ),
 .UNSPECIFIED. ) 
 CURVE ( )  GEOMETRIC_REPRESENTATION_ITEM ( )  RATIONAL_B_SPLINE_CURVE ( ( 0.9999999999999938938, 0.9238795325112928447, 1.000000000000000000, 0.9238795325112867385, 1.000000000000000000, 0.9238795325112867385, 1.000000000000000000, 0.9238795325112796331, 1.000000000000007105 ) ) 
 REPRESENTATION_ITEM ( '' )  );
#29827=CARTESIAN_POINT ( 'NONE',  ( -54.64476657466781973, -131.8125000013656063, -4.444560631937228834 ) ) ;
#29830=CARTESIAN_POINT ( 'NONE',  ( -49.85088928181150436, -146.6875000027312126, -1.666127454062680480 ) ) ;
#29843=CARTESIAN_POINT ( 'NONE',  ( -59.29741812935640155, -138.6250000013655779, -2.196230717870135685 ) ) ;
#29855=CARTESIAN_POINT ( 'NONE',  ( -55.39835681537999790, -153.0000000027312410, 4.984105922594378235 ) ) ;
#29876=CARTESIAN_POINT ( 'NONE',  ( -50.70258187064364108, -149.1250000013656063, 2.196230717870141014 ) ) ;
#29884=CARTESIAN_POINT ( 'NONE',  ( -57.19623071787017210, -125.6250000013656205, 4.297418129356382899 ) ) ;
#29894=CARTESIAN_POINT ( 'NONE',  ( -56.66612745406270335, -152.4375000027311842, -5.149110718188516067 ) ) ;
#29899=EDGE_CURVE ( 'NONE', #16288, #3805, #8610, .T. ) ;
#29909=ORIENTED_EDGE ( 'NONE', *, *, #8580, .T. ) ;
#29914=VECTOR ( 'NONE', #4364, 1000.000000000000000 ) ;
#29916=EDGE_CURVE ( 'NONE', #35585, #1423, #34904, .T. ) ;
#29918=CARTESIAN_POINT ( 'NONE',  ( -58.39396692619412477, -148.4375000013656063, 2.891590998281057701 ) ) ;
#29941=CARTESIAN_POINT ( 'NONE',  ( -58.09382797660032338, -135.0000000000000284, -3.377790754402798967 ) ) ;
#29942=ORIENTED_EDGE ( 'NONE', *, *, #50397, .T. ) ;
#29963=CARTESIAN_POINT ( 'NONE',  ( -52.80376928212989185, -138.1250000013656063, -4.297418129356379346 ) ) ;
#29973=CARTESIAN_POINT ( 'NONE',  ( -58.24261429053147765, -140.2500000000000000, -3.805975901505573855 ) ) ;
#29982=CARTESIAN_POINT ( 'NONE',  ( -59.29741812935640155, -141.6250000013656063, -2.196230717870135685 ) ) ;
#30008=CARTESIAN_POINT ( 'NONE',  ( -52.10840900171896806, -145.4375000013656063, 3.393966926194110556 ) ) ;
#30024=CARTESIAN_POINT ( 'NONE',  ( -51.75738570946856498, -138.8750000027312126, 3.805975901505576964 ) ) ;
#30048=CARTESIAN_POINT ( 'NONE',  ( -53.33387254593733928, -127.8125000000000142, 5.149110718188519620 ) ) ;
#30056=CARTESIAN_POINT ( 'NONE',  ( -51.60603307380591787, -151.9375000013656063, -2.891590998281053704 ) ) ;
#30078=CARTESIAN_POINT ( 'NONE',  ( -51.60603307380591787, -125.9375000013656063, -2.891590998281053704 ) ) ;
#30079=CARTESIAN_POINT ( 'NONE',  ( -54.64476657466781973, -143.8125000013656063, -4.444560631937228834 ) ) ;
#30111=ORIENTED_EDGE ( 'NONE', *, *, #31183, .F. ) ;
#30120=ORIENTED_EDGE ( 'NONE', *, *, #33369, .F. ) ;
#30121=CARTESIAN_POINT ( 'NONE',  ( -49.85088928181150436, -140.5625000000000284, -1.666127454062680702 ) ) ;
#30130=CARTESIAN_POINT ( 'NONE',  ( -58.39396692619412477, -145.6875000013656063, 2.891590998281057701 ) ) ;
#30132=CARTESIAN_POINT ( 'NONE',  ( -50.18089887299979068, -135.8125000027312126, 2.462841084822635640 ) ) ;
#30144=CARTESIAN_POINT ( 'NONE',  ( -51.60603307380591787, -127.9375000013656063, -2.891590998281053704 ) ) ;
#30148=CARTESIAN_POINT ( 'NONE',  ( -51.75738570946856498, -136.7500000000000284, 3.805975901505576964 ) ) ;
#30159=CARTESIAN_POINT ( 'NONE',  ( -54.64476657466781973, -135.8125000013656063, -4.444560631937228834 ) ) ;
#30167=CARTESIAN_POINT ( 'NONE',  ( -50.70258187064364108, -130.3750000013656631, 2.196230717870141014 ) ) ;
#30192=CARTESIAN_POINT ( 'NONE',  ( -58.39396692619412477, -150.4375000013656063, 2.891590998281057701 ) ) ;
#30198=DIRECTION ( 'NONE',  ( -0.000000000000000000, -1.000000000000000000, 0.000000000000000000 ) ) ;
#30199=CARTESIAN_POINT ( 'NONE',  ( -58.80597590150559739, -155.0000000000000284, 3.242614290531460330 ) ) ;
#30213=CARTESIAN_POINT ( 'NONE',  ( -52.53715891517739323, -146.5625000027311842, -4.819101127000233298 ) ) ;
#30216=EDGE_CURVE ( 'NONE', #18086, #11538, #24138, .T. ) ;
#30230=CARTESIAN_POINT ( 'NONE',  ( -55.39835681537999790, -137.8750000000000284, 4.984105922594378235 ) ) ;
#30231=CARTESIAN_POINT ( 'NONE',  ( -52.10840900171896806, -148.1875000013656063, 3.393966926194110556 ) ) ;
#30237=DIRECTION ( 'NONE',  ( -0.4999999999999998335, 0.000000000000000000, 0.8660254037844388186 ) ) ;
#30250=DIRECTION ( 'NONE',  ( -0.6485228581062915110, 0.000000000000000000, -0.7611951803011149931 ) ) ;
#30271=DIRECTION ( 'NONE',  ( 0.000000000000000000, 1.000000000000000000, 0.000000000000000000 ) ) ;
#30273=ORIENTED_EDGE ( 'NONE', *, *, #25652, .F. ) ;
#30282=CARTESIAN_POINT ( 'NONE',  ( -53.51423613279429503, -137.5000000013656063, 4.591703134518082763 ) ) ;
#30288=EDGE_CURVE ( 'NONE', #25936, #18086, #18985, .T. ) ;
#30290=CARTESIAN_POINT ( 'NONE',  ( -52.46430154831001857, -135.0000000000000284, -3.678960875299264188 ) ) ;
#30301=CARTESIAN_POINT ( 'NONE',  ( -52.10840900171896806, -141.1875000013656063, 3.393966926194110556 ) ) ;
#30302=CARTESIAN_POINT ( 'NONE',  ( -57.46284108482265651, -154.9375000000000000, 4.819101127000238627 ) ) ;
#30326=CARTESIAN_POINT ( 'NONE',  ( -59.29741812935640155, -144.8750000013655779, -2.196230717870135685 ) ) ;
#30343=AXIS2_PLACEMENT_3D ( 'NONE', #20589, #54357, #40195 ) ;
#30353=EDGE_CURVE ( 'NONE', #19989, #42565, #3896, .T. ) ;
#30371=CARTESIAN_POINT ( 'NONE',  ( -51.75738570946856498, -130.7500000000000284, 3.805975901505576964 ) ) ;
#30378=CARTESIAN_POINT ( 'NONE',  ( -59.59170313451811296, -153.5000000013656063, 1.485763867205729394 ) ) ;
#30381=CARTESIAN_POINT ( 'NONE',  ( -55.39835681537999790, -147.0000000027312126, 4.984105922594378235 ) ) ;
#30404=CARTESIAN_POINT ( 'NONE',  ( -57.89159099828107458, -126.6875000013656063, -3.393966926194107447 ) ) ;
#30405=CARTESIAN_POINT ( 'NONE',  ( -59.44456063193725015, -141.5625000013656063, -0.3552334253322034230 ) ) ;
#30423=CARTESIAN_POINT ( 'NONE',  ( -51.75738570946856498, -155.0000000000000284, 3.805975901505577408 ) ) ;
#30437=( BOUNDED_CURVE ( )  B_SPLINE_CURVE ( 2, ( #14856, #19691, #53161, #4900, #13918, #54099, #53782, #33232, #5221 ),
 .UNSPECIFIED., .F., .F. ) 
 B_SPLINE_CURVE_WITH_KNOTS ( ( 3, 2, 2, 2, 3 ),
 ( 0.1416666666666667740, 0.1458333333333334814, 0.1500000000000001332, 0.1541666666666668406, 0.1583333333333334925 ),
 .UNSPECIFIED. ) 
 CURVE ( )  GEOMETRIC_REPRESENTATION_ITEM ( )  RATIONAL_B_SPLINE_CURVE ( ( 0.9999999999999980016, 0.9238795325112887369, 1.000000000000000000, 0.9238795325112867385, 1.000000000000000000, 0.9238795325112867385, 1.000000000000000000, 0.9238795325112837409, 1.000000000000003109 ) ) 
 REPRESENTATION_ITEM ( '' )  );
#30444=CARTESIAN_POINT ( 'NONE',  ( -53.33387254593733928, -142.8125000000000568, 5.149110718188519620 ) ) ;
#30454=CARTESIAN_POINT ( 'NONE',  ( -51.60603307380591787, -147.1875000013656063, -2.891590998281053704 ) ) ;
#30456=CARTESIAN_POINT ( 'NONE',  ( -58.80597590150559739, -133.1250000027312126, 3.242614290531460330 ) ) ;
#30468=CARTESIAN_POINT ( 'NONE',  ( -53.51423613279429503, -128.2500000013656063, 4.591703134518082763 ) ) ;
#30485=CARTESIAN_POINT ( 'NONE',  ( -55.35523342533222291, -139.3125000013656063, 4.444560631937231499 ) ) ;
#30486=VECTOR ( 'NONE', #28587, 1000.000000000000114 ) ;
#30496=CARTESIAN_POINT ( 'NONE',  ( -50.40829686548195099, -133.2500000013656347, -1.485763867205728284 ) ) ;
#30504=CARTESIAN_POINT ( 'NONE',  ( -51.19402409849444524, -151.5000000000000284, -3.242614290531456334 ) ) ;
#30506=ORIENTED_EDGE ( 'NONE', *, *, #30353, .T. ) ;
#30519=CARTESIAN_POINT ( 'NONE',  ( -59.44456063193725015, -150.5625000013656063, -0.3552334253322034230 ) ) ;
#30526=CARTESIAN_POINT ( 'NONE',  ( -51.75738570946856498, -151.7500000000000284, 3.805975901505576964 ) ) ;
#30530=CARTESIAN_POINT ( 'NONE',  ( -56.66612745406293783, -136.4375000027312126, -5.149110718188535607 ) ) ;
#30538=CARTESIAN_POINT ( 'NONE',  ( -51.75738570946856498, -147.8750000027312126, 3.805975901505576964 ) ) ;
#30554=CARTESIAN_POINT ( 'NONE',  ( -59.98410592259440222, -138.1250000000000284, -0.3983568153799752487 ) ) ;
#30555=CARTESIAN_POINT ( 'NONE',  ( -59.59170313451811296, -149.5000000013655779, 1.485763867205729394 ) ) ;
#30560=CARTESIAN_POINT ( 'NONE',  ( -55.00000000000002132, -155.0000000000000284, 1.734723475976807094E-15 ) ) ;
#30583=CARTESIAN_POINT ( 'NONE',  ( -56.75196168792112417, -135.0000000000000853, -4.145498605701915196 ) ) ;
#30606=CARTESIAN_POINT ( 'NONE',  ( -50.70258187064364108, -135.3750000013656063, 2.196230717870141014 ) ) ;
#30625=CARTESIAN_POINT ( 'NONE',  ( -57.89159099828107458, -141.6875000013656063, -3.393966926194107447 ) ) ;
#30650=EDGE_CURVE ( 'NONE', #21128, #10962, #41526, .T. ) ;
#30653=CARTESIAN_POINT ( 'NONE',  ( -52.10840900171896806, -142.4375000013656063, 3.393966926194110556 ) ) ;
#30681=( BOUNDED_CURVE ( )  B_SPLINE_CURVE ( 2, ( #44618, #43974, #34986, #11167, #19857 ),
 .UNSPECIFIED., .F., .F. ) 
 B_SPLINE_CURVE_WITH_KNOTS ( ( 3, 2, 3 ),
 ( 0.6583333333333329929, 0.6624999999999996447, 0.6666666666666662966 ),
 .UNSPECIFIED. ) 
 CURVE ( )  GEOMETRIC_REPRESENTATION_ITEM ( )  RATIONAL_B_SPLINE_CURVE ( ( 1.000000000000005995, 0.9238795325112806323, 1.000000000000000000, 0.9238795325112928447, 0.9999999999999938938 ) ) 
 REPRESENTATION_ITEM ( '' )  );
#30693=ORIENTED_EDGE ( 'NONE', *, *, #16593, .F. ) ;
#30698=CARTESIAN_POINT ( 'NONE',  ( -52.53715891517739323, -128.4375000000000284, -4.819101127000233298 ) ) ;
#30704=CARTESIAN_POINT ( 'NONE',  ( -55.35523342533222291, -151.3125000013656063, 4.444560631937231499 ) ) ;
#30731=CARTESIAN_POINT ( 'NONE',  ( -57.89159099828107458, -125.6875000013656063, -3.393966926194107447 ) ) ;
#30732=CARTESIAN_POINT ( 'NONE',  ( -59.44456063193725015, -143.5625000013656063, -0.3552334253322034230 ) ) ;
#30743=ORIENTED_EDGE ( 'NONE', *, *, #29899, .T. ) ;
#30763=ORIENTED_EDGE ( 'NONE', *, *, #19972, .T. ) ;
#30771=CARTESIAN_POINT ( 'NONE',  ( -56.66612745406270335, -143.3125000000000284, -5.149110718188516067 ) ) ;
#30773=LINE ( 'NONE', #24996, #57036 ) ;
#30775=( BOUNDED_CURVE ( )  B_SPLINE_CURVE ( 2, ( #55174, #21074, #55498, #10781, #31032, #60643, #11093, #50982, #15287 ),
 .UNSPECIFIED., .F., .F. ) 
 B_SPLINE_CURVE_WITH_KNOTS ( ( 3, 2, 2, 2, 3 ),
 ( 0.2583333333333335813, 0.2625000000000002331, 0.2666666666666668850, 0.2708333333333335369, 0.2750000000000002442 ),
 .UNSPECIFIED. ) 
 CURVE ( )  GEOMETRIC_REPRESENTATION_ITEM ( )  RATIONAL_B_SPLINE_CURVE ( ( 0.9999999999999958922, 0.9238795325112908463, 1.000000000000000000, 0.9238795325112867385, 1.000000000000000000, 0.9238795325112867385, 1.000000000000000000, 0.9238795325112826307, 1.000000000000003997 ) ) 
 REPRESENTATION_ITEM ( '' )  );
#30782=CARTESIAN_POINT ( 'NONE',  ( -56.48576386720575471, -143.0000000013655779, -4.591703134518078322 ) ) ;
#30784=CARTESIAN_POINT ( 'NONE',  ( -54.60164318462004474, -134.5000000027312126, -4.984105922594373794 ) ) ;
#30797=CARTESIAN_POINT ( 'NONE',  ( -54.64476657466781973, -127.8125000013655921, -4.444560631937228834 ) ) ;
#30811=CARTESIAN_POINT ( 'NONE',  ( -57.19623071787017210, -136.3750000013656063, 4.297418129356382899 ) ) ;
#30822=CARTESIAN_POINT ( 'NONE',  ( -59.44456063193725015, -133.8125000013656063, -0.3552334253322034230 ) ) ;
#30827=ADVANCED_FACE ( 'NONE', ( #2955 ), #2431, .F. ) ;
#30828=FACE_OUTER_BOUND ( 'NONE', #22618, .T. ) ;
#30854=VECTOR ( 'NONE', #28045, 1000.000000000000000 ) ;
#30855=CARTESIAN_POINT ( 'NONE',  ( -50.18089887299979068, -151.6875000000000284, 2.462841084822635640 ) ) ;
#30865=CARTESIAN_POINT ( 'NONE',  ( -55.39835681537999790, -148.0000000027312126, 4.984105922594378235 ) ) ;
#30882=CARTESIAN_POINT ( 'NONE',  ( -51.75738570946856498, -137.7500000000000000, 3.805975901505576964 ) ) ;
#30883=CARTESIAN_POINT ( 'NONE',  ( -50.40829686548195099, -150.0000000013655779, -1.485763867205728284 ) ) ;
#30927=CARTESIAN_POINT ( 'NONE',  ( -50.55543936806279248, -136.3125000013656063, 0.3552334253322060320 ) ) ;
#30933=CARTESIAN_POINT ( 'NONE',  ( -56.09268833151246980, -135.0000000000000853, -4.332774804594910378 ) ) ;
#30934=EDGE_LOOP ( 'NONE', ( #4402, #23742, #2671, #63278 ) ) ;
#30971=CARTESIAN_POINT ( 'NONE',  ( -50.55543936806279248, -141.3125000013656063, 0.3552334253322060320 ) ) ;
#30988=DIRECTION ( 'NONE',  ( 0.000000000000000000, 1.000000000000000000, 0.000000000000000000 ) ) ;
#30989=CARTESIAN_POINT ( 'NONE',  ( -50.55543936806279248, -136.3125000013656063, 0.3552334253322060320 ) ) ;
#31001=CARTESIAN_POINT ( 'NONE',  ( -57.89159099828107458, -146.9375000013656063, -3.393966926194107447 ) ) ;
#31010=CARTESIAN_POINT ( 'NONE',  ( -59.81910112700025905, -128.1875000000000568, -2.462841084822630311 ) ) ;
#31018=CARTESIAN_POINT ( 'NONE',  ( -59.98410592259440222, -124.2500000027311984, -0.3983568153799752487 ) ) ;
#31032=CARTESIAN_POINT ( 'NONE',  ( -58.80597590150559739, -147.0000000000000284, 3.242614290531460330 ) ) ;
#31037=FACE_OUTER_BOUND ( 'NONE', #62487, .T. ) ;
#31044=CARTESIAN_POINT ( 'NONE',  ( -59.59170313451811296, -151.7500000013655779, 1.485763867205729394 ) ) ;
#31045=CARTESIAN_POINT ( 'NONE',  ( -52.80376928212989185, -141.8750000013655779, -4.297418129356378458 ) ) ;
#31068=ORIENTED_EDGE ( 'NONE', *, *, #48349, .T. ) ;
#31086=CARTESIAN_POINT ( 'NONE',  ( -53.33387254593733928, -139.8125000000000000, 5.149110718188519620 ) ) ;
#31097=CARTESIAN_POINT ( 'NONE',  ( -50.55543936806279248, -144.3125000013656063, 0.3552334253322060320 ) ) ;
#31099=CARTESIAN_POINT ( 'NONE',  ( -51.19402409849444524, -134.6250000027312126, -3.242614290531456334 ) ) ;
#31111=CARTESIAN_POINT ( 'NONE',  ( -55.35523342533222291, -127.3125000013655921, 4.444560631937231499 ) ) ;
#31113=CARTESIAN_POINT ( 'NONE',  ( -58.24261429053147765, -142.3750000027312126, -3.805975901505573855 ) ) ;
#31125=CARTESIAN_POINT ( 'NONE',  ( -54.64476657466781973, -137.8125000013656063, -4.444560631937228834 ) ) ;
#31134=CARTESIAN_POINT ( 'NONE',  ( -56.48576386720575471, -131.0000000013656063, -4.591703134518078322 ) ) ;
#31139=CARTESIAN_POINT ( 'NONE',  ( -55.00000000000002132, -155.0000000000000284, 1.734723475976807094E-15 ) ) ;
#31143=CARTESIAN_POINT ( 'NONE',  ( -56.66612745406273888, -151.3125000000000000, -5.149110718188520508 ) ) ;
#31167=CARTESIAN_POINT ( 'NONE',  ( -52.53715891517739323, -154.4375000000000284, -4.819101127000233298 ) ) ;
#31179=CARTESIAN_POINT ( 'NONE',  ( -57.46284108482265651, -145.0625000027312126, 4.819101127000239515 ) ) ;
#31183=EDGE_CURVE ( 'NONE', #59424, #7528, #30775, .T. ) ;
#31191=ORIENTED_EDGE ( 'NONE', *, *, #44158, .T. ) ;
#31198=CARTESIAN_POINT ( 'NONE',  ( -50.70258187064364108, -149.1250000013656063, 2.196230717870141014 ) ) ;
#31226=FACE_OUTER_BOUND ( 'NONE', #47303, .T. ) ;
#31240=CARTESIAN_POINT ( 'NONE',  ( -50.70258187064364108, -136.3750000013656063, 2.196230717870141014 ) ) ;
#31245=CARTESIAN_POINT ( 'NONE',  ( -53.23292615868056288, -134.9999999999999432, -4.104181387521468771 ) ) ;
#31252=CARTESIAN_POINT ( 'NONE',  ( -51.19402409849444524, -149.5000000000000284, -3.242614290531456334 ) ) ;
#31280=CARTESIAN_POINT ( 'NONE',  ( -51.60603307380591787, -138.1875000013656347, -2.891590998281053704 ) ) ;
#31299=CARTESIAN_POINT ( 'NONE',  ( -57.89159099828107458, -136.9375000013655779, -3.393966926194107447 ) ) ;
#31312=CARTESIAN_POINT ( 'NONE',  ( -57.89159099828107458, -148.9375000013656063, -3.393966926194107447 ) ) ;
#31320=CARTESIAN_POINT ( 'NONE',  ( -58.24261429053147765, -149.3750000027312126, -3.805975901505573855 ) ) ;
#31325=CARTESIAN_POINT ( 'NONE',  ( -50.01589407740564042, -125.6250000000000142, 0.3983568153799778022 ) ) ;
#31332=CARTESIAN_POINT ( 'NONE',  ( -57.19623071787017210, -148.3750000013656063, 4.297418129356382899 ) ) ;
#31339=CARTESIAN_POINT ( 'NONE',  ( -54.60164318462004474, -152.5000000027312410, -4.984105922594373794 ) ) ;
#31348=EDGE_LOOP ( 'NONE', ( #404, #38128, #30763, #28320, #50633, #1815 ) ) ;
#31354=CARTESIAN_POINT ( 'NONE',  ( -50.40829686548195099, -152.2500000013656347, -1.485763867205728284 ) ) ;
#31355=CARTESIAN_POINT ( 'NONE',  ( -53.51423613279429503, -143.2500000013656063, 4.591703134518083651 ) ) ;
#31358=CARTESIAN_POINT ( 'NONE',  ( -60.14911071818854538, -137.0625000000000284, 1.666127454062681146 ) ) ;
#31367=CARTESIAN_POINT ( 'NONE',  ( -57.46284108482265651, -135.9375000000000284, 4.819101127000238627 ) ) ;
#31379=ORIENTED_EDGE ( 'NONE', *, *, #54341, .T. ) ;
#31394=CARTESIAN_POINT ( 'NONE',  ( -50.18089887299979068, -140.6875000000000284, 2.462841084822635640 ) ) ;
#31404=CARTESIAN_POINT ( 'NONE',  ( -57.89159099828107458, -142.9375000013656063, -3.393966926194107447 ) ) ;
#31406=CARTESIAN_POINT ( 'NONE',  ( -50.18089887299979068, -128.8125000027312126, 2.462841084822635640 ) ) ;
#31418=CARTESIAN_POINT ( 'NONE',  ( -59.59170313451811296, -129.5000000013656347, 1.485763867205729394 ) ) ;
#31433=CARTESIAN_POINT ( 'NONE',  ( -57.89159099828107458, -133.6875000013656063, -3.393966926194107447 ) ) ;
#31443=CARTESIAN_POINT ( 'NONE',  ( -51.60603307380591787, -127.1875000013656063, -2.891590998281053704 ) ) ;
#31471=CARTESIAN_POINT ( 'NONE',  ( -50.40829686548195099, -138.0000000013656063, -1.485763867205728284 ) ) ;
#31476=CARTESIAN_POINT ( 'NONE',  ( -58.80597590150559739, -153.0000000000000284, 3.242614290531460330 ) ) ;
#31486=CARTESIAN_POINT ( 'NONE',  ( -57.46284108482265651, -147.0625000027312126, 4.819101127000239515 ) ) ;
#31509=CARTESIAN_POINT ( 'NONE',  ( -59.44456063193725015, -145.5625000013656063, -0.3552334253322034230 ) ) ;
#31533=DIRECTION ( 'NONE',  ( -0.000000000000000000, -1.000000000000000000, 0.000000000000000000 ) ) ;
#31554=LINE ( 'NONE', #26736, #40500 ) ;
#31557=ORIENTED_EDGE ( 'NONE', *, *, #25652, .T. ) ;
#31566=CARTESIAN_POINT ( 'NONE',  ( -52.80376928212989185, -136.1250000013656063, -4.297418129356379346 ) ) ;
#31572=VERTEX_POINT ( 'NONE', #56766 ) ;
#31578=CARTESIAN_POINT ( 'NONE',  ( -51.75738570946856498, -149.7500000000000284, 3.805975901505576964 ) ) ;
#31587=VECTOR ( 'NONE', #33554, 1000.000000000000000 ) ;
#31609=CARTESIAN_POINT ( 'NONE',  ( -56.48576386720575471, -142.0000000013656063, -4.591703134518078322 ) ) ;
#31624=DIRECTION ( 'NONE',  ( 0.000000000000000000, 1.000000000000000000, 0.000000000000000000 ) ) ;
#31627=FACE_OUTER_BOUND ( 'NONE', #58438, .T. ) ;
#31628=EDGE_CURVE ( 'NONE', #51345, #52848, #28327, .T. ) ;
#31629=CARTESIAN_POINT ( 'NONE',  ( -54.64476657466781973, -135.0625000013656063, -4.444560631937228834 ) ) ;
#31643=CARTESIAN_POINT ( 'NONE',  ( -50.55543936806279248, -148.3125000013656063, 0.3552334253322060320 ) ) ;
#31661=CARTESIAN_POINT ( 'NONE',  ( -50.55543936806279248, -150.0625000013656063, 0.3552334253322060320 ) ) ;
#31685=CARTESIAN_POINT ( 'NONE',  ( -50.70258187064364108, -152.3750000013656063, 2.196230717870141014 ) ) ;
#31689=CARTESIAN_POINT ( 'NONE',  ( -51.19402409849444524, -153.6250000027312126, -3.242614290531456334 ) ) ;
#31725=CARTESIAN_POINT ( 'NONE',  ( -49.85088928181150436, -137.5625000000000284, -1.666127454062680702 ) ) ;
#31730=ORIENTED_EDGE ( 'NONE', *, *, #62817, .F. ) ;
#31736=CARTESIAN_POINT ( 'NONE',  ( -55.35523342533222291, -143.5625000013656063, 4.444560631937231499 ) ) ;
#31738=CARTESIAN_POINT ( 'NONE',  ( -54.60164318462004474, -132.5000000027312126, -4.984105922594373794 ) ) ;
#31749=CARTESIAN_POINT ( 'NONE',  ( -58.39396692619412477, -126.4375000013656063, 2.891590998281057701 ) ) ;
#31761=CARTESIAN_POINT ( 'NONE',  ( -55.35523342533222291, -133.3125000013656063, 4.444560631937231499 ) ) ;
#31771=CARTESIAN_POINT ( 'NONE',  ( -57.19623071787017210, -126.6250000013656489, 4.297418129356382899 ) ) ;
#31774=AXIS2_PLACEMENT_3D ( 'NONE', #35334, #6079, #9919 ) ;
#31793=CARTESIAN_POINT ( 'NONE',  ( -52.10840900171896806, -153.4375000013656063, 3.393966926194110556 ) ) ;
#31797=CARTESIAN_POINT ( 'NONE',  ( -59.29741812935640155, -138.6250000013656063, -2.196230717870135685 ) ) ;
#31802=CARTESIAN_POINT ( 'NONE',  ( -58.80597590150559739, -149.0000000000000284, 3.242614290531460330 ) ) ;
#31812=CARTESIAN_POINT ( 'NONE',  ( -51.60603307380591787, -154.1875000013656063, -2.891590998281053704 ) ) ;
#31813=CARTESIAN_POINT ( 'NONE',  ( -51.19402409849444524, -143.6250000027312126, -3.242614290531456334 ) ) ;
#31816=EDGE_CURVE ( 'NONE', #44367, #31572, #37358, .T. ) ;
#31825=CARTESIAN_POINT ( 'NONE',  ( -54.64476657466781973, -139.8125000013656063, -4.444560631937228834 ) ) ;
#31838=CARTESIAN_POINT ( 'NONE',  ( -57.19623071787017210, -147.3750000013656063, 4.297418129356382899 ) ) ;
#31843=CARTESIAN_POINT ( 'NONE',  ( -54.60164318462004474, -141.5000000027312126, -4.984105922594373794 ) ) ;
#31881=CARTESIAN_POINT ( 'NONE',  ( -55.35523342533222291, -133.5625000013656063, 4.444560631937231499 ) ) ;
#31891=CARTESIAN_POINT ( 'NONE',  ( -53.33387254593733928, -153.9375000027312126, 5.149110718188519620 ) ) ;
#31927=CARTESIAN_POINT ( 'NONE',  ( -59.29741812935640155, -138.8750000013655779, -2.196230717870135685 ) ) ;
#31944=CARTESIAN_POINT ( 'NONE',  ( -50.55543936806279248, -135.3125000013656063, 0.3552334253322060320 ) ) ;
#31955=CARTESIAN_POINT ( 'NONE',  ( -59.29741812935640155, -148.8750000013655779, -2.196230717870135685 ) ) ;
#31968=CARTESIAN_POINT ( 'NONE',  ( -51.19402409849444524, -125.5000000000000284, -3.242614290531456334 ) ) ;
#31976=CARTESIAN_POINT ( 'NONE',  ( -54.64476657466781973, -148.8125000013656063, -4.444560631937228834 ) ) ;
#32001=CARTESIAN_POINT ( 'NONE',  ( -54.64476657466781973, -153.0625000013656063, -4.444560631937228834 ) ) ;
#32005=CARTESIAN_POINT ( 'NONE',  ( -49.85088928181150436, -153.6875000027311842, -1.666127454062680480 ) ) ;
#32017=CARTESIAN_POINT ( 'NONE',  ( -51.19402409849444524, -152.5000000000000284, -3.242614290531456334 ) ) ;
#32032=ORIENTED_EDGE ( 'NONE', *, *, #40525, .T. ) ;
#32036=CARTESIAN_POINT ( 'NONE',  ( -58.24261429053147765, -139.2500000000000000, -3.805975901505573855 ) ) ;
#32045=CARTESIAN_POINT ( 'NONE',  ( -59.29741812935640155, -140.8750000013656063, -2.196230717870135685 ) ) ;
#32047=CARTESIAN_POINT ( 'NONE',  ( -50.18089887299979068, -130.8125000027312410, 2.462841084822635640 ) ) ;
#32059=CARTESIAN_POINT ( 'NONE',  ( -50.40829686548195099, -125.0000000013656205, -1.485763867205728284 ) ) ;
#32071=CARTESIAN_POINT ( 'NONE',  ( -50.70258187064364108, -135.1250000013656063, 2.196230717870141014 ) ) ;
#32079=VERTEX_POINT ( 'NONE', #2979 ) ;
#32081=CARTESIAN_POINT ( 'NONE',  ( -52.80376928212989185, -129.1250000013655779, -4.297418129356379346 ) ) ;
#32109=CARTESIAN_POINT ( 'NONE',  ( -57.19623071787016499, -138.3750000013656063, 4.297418129356382899 ) ) ;
#32114=CARTESIAN_POINT ( 'NONE',  ( -51.19402409849444524, -150.5000000000000284, -3.242614290531456334 ) ) ;
#32118=( LENGTH_UNIT ( ) NAMED_UNIT ( * ) SI_UNIT ( .MILLI., .METRE. ) );
#32123=CARTESIAN_POINT ( 'NONE',  ( -50.70258187064364108, -153.3750000013656063, 2.196230717870141014 ) ) ;
#32124=CARTESIAN_POINT ( 'NONE',  ( -55.39835681537999790, -143.0000000027312126, 4.984105922594378235 ) ) ;
#32130=CARTESIAN_POINT ( 'NONE',  ( -58.24261429053147765, -153.2500000000000284, -3.805975901505573855 ) ) ;
#32131=CARTESIAN_POINT ( 'NONE',  ( -54.64476657466781973, -138.8125000013656063, -4.444560631937228834 ) ) ;
#32146=CARTESIAN_POINT ( 'NONE',  ( -55.00000000000002132, -155.0000000000000284, 1.734723475976807094E-15 ) ) ;
#32147=CARTESIAN_POINT ( 'NONE',  ( -55.35523342533222291, -147.3125000013656063, 4.444560631937231499 ) ) ;
#32160=CARTESIAN_POINT ( 'NONE',  ( -60.14911071818854538, -152.1875000027312126, 1.666127454062681146 ) ) ;
#32191=CARTESIAN_POINT ( 'NONE',  ( -58.39396692619412477, -130.6875000013656063, 2.891590998281057701 ) ) ;
#32199=VERTEX_POINT ( 'NONE', #37373 ) ;
#32200=CARTESIAN_POINT ( 'NONE',  ( -51.75738570946856498, -153.8750000027312126, 3.805975901505576964 ) ) ;
#32235=CARTESIAN_POINT ( 'NONE',  ( -51.60603307380591787, -139.1875000013656347, -2.891590998281053704 ) ) ;
#32270=CARTESIAN_POINT ( 'NONE',  ( -58.39396692619412477, -144.6875000013656063, 2.891590998281057701 ) ) ;
#32274=ORIENTED_EDGE ( 'NONE', *, *, #16862, .T. ) ;
#32282=CARTESIAN_POINT ( 'NONE',  ( -59.98410592259440222, -127.1250000000000142, -0.3983568153799752487 ) ) ;
#32291=CARTESIAN_POINT ( 'NONE',  ( -52.10840900171896806, -147.1875000013656063, 3.393966926194110556 ) ) ;
#32294=ORIENTED_EDGE ( 'NONE', *, *, #44808, .F. ) ;
#32310=ORIENTED_EDGE ( 'NONE', *, *, #63072, .F. ) ;
#32314=CARTESIAN_POINT ( 'NONE',  ( -59.59170313451811296, -150.7500000013655495, 1.485763867205729394 ) ) ;
#32359=CARTESIAN_POINT ( 'NONE',  ( -54.60164318462004474, -138.3750000000000284, -4.984105922594373794 ) ) ;
#32364=CARTESIAN_POINT ( 'NONE',  ( -58.24261429053147765, -141.3750000027312126, -3.805975901505573855 ) ) ;
#32367=CARTESIAN_POINT ( 'NONE',  ( -55.35523342533222291, -138.5625000013656063, 4.444560631937231499 ) ) ;
#32369=CARTESIAN_POINT ( 'NONE',  ( -51.19402409849444524, -129.6250000027312126, -3.242614290531456334 ) ) ;
#32375=CARTESIAN_POINT ( 'NONE',  ( -58.80597590150559739, -151.1250000027312126, 3.242614290531460330 ) ) ;
#32383=CARTESIAN_POINT ( 'NONE',  ( -57.19623071787017210, -126.3750000013656489, 4.297418129356382899 ) ) ;
#32394=CARTESIAN_POINT ( 'NONE',  ( -50.40829686548195099, -135.0000000013656347, -1.485763867205728284 ) ) ;
#32404=CARTESIAN_POINT ( 'NONE',  ( -55.35523342533222291, -128.5625000013656063, 4.444560631937231499 ) ) ;
#32418=CARTESIAN_POINT ( 'NONE',  ( -48.00000000000002132, -155.0000000000000284, 4.041451884327384114 ) ) ;
#32428=CARTESIAN_POINT ( 'NONE',  ( -55.35523342533222291, -153.5625000013656063, 4.444560631937231499 ) ) ;
#32432=CARTESIAN_POINT ( 'NONE',  ( -54.64476657466781973, -138.8125000013656063, -4.444560631937228834 ) ) ;
#32437=CARTESIAN_POINT ( 'NONE',  ( -54.60164318462004474, -148.3750000000000284, -4.984105922594373794 ) ) ;
#32445=CARTESIAN_POINT ( 'NONE',  ( -59.44456063193725015, -152.8125000013656063, -0.3552334253322034230 ) ) ;
#32446=CARTESIAN_POINT ( 'NONE',  ( -59.98410592259440222, -144.2500000027312126, -0.3983568153799752487 ) ) ;
#32453=CARTESIAN_POINT ( 'NONE',  ( -59.29741812935640155, -135.6250000013655779, -2.196230717870135685 ) ) ;
#32470=CARTESIAN_POINT ( 'NONE',  ( -57.89159099828107458, -146.6875000013656063, -3.393966926194107447 ) ) ;
#32510=CARTESIAN_POINT ( 'NONE',  ( -50.55543936806279248, -131.3125000013656063, 0.3552334253322060320 ) ) ;
#32519=CARTESIAN_POINT ( 'NONE',  ( -59.81910112700025905, -153.3125000027312126, -2.462841084822630311 ) ) ;
#32523=ADVANCED_FACE ( 'NONE', ( #23533, #43133 ), #62773, .F. ) ;
#32525=VERTEX_POINT ( 'NONE', #48588 ) ;
#32538=CARTESIAN_POINT ( 'NONE',  ( -55.39835681537999790, -144.8750000000000284, 4.984105922594378235 ) ) ;
#32540=CARTESIAN_POINT ( 'NONE',  ( -50.18089887299976937, -138.6875000000000000, 2.462841084822337656 ) ) ;
#32558=CARTESIAN_POINT ( 'NONE',  ( -52.80376928212989185, -135.1250000013656063, -4.297418129356379346 ) ) ;
#32590=CARTESIAN_POINT ( 'NONE',  ( -59.59170313451811296, -143.7500000013656063, 1.485763867205729394 ) ) ;
#32600=CARTESIAN_POINT ( 'NONE',  ( -50.01589407740564042, -126.6250000000000142, 0.3983568153799778022 ) ) ;
#32603=ADVANCED_FACE ( 'NONE', ( #34756 ), #60172, .F. ) ;
#32609=CARTESIAN_POINT ( 'NONE',  ( -56.48576386720575471, -149.7500000013656063, -4.591703134518078322 ) ) ;
#32634=CARTESIAN_POINT ( 'NONE',  ( -57.19623071787017210, -149.6250000013655779, 4.297418129356382899 ) ) ;
#32656=CARTESIAN_POINT ( 'NONE',  ( -55.00000000000002132, -155.0000000000000284, 1.734723475976807094E-15 ) ) ;
#32672=CARTESIAN_POINT ( 'NONE',  ( -58.80597590150559739, -138.0000000000000284, 3.242614290531460330 ) ) ;
#32684=CARTESIAN_POINT ( 'NONE',  ( -52.10840900171896806, -138.4375000013656063, 3.393966926194110556 ) ) ;
#32686=CARTESIAN_POINT ( 'NONE',  ( -60.14911071818854538, -131.1875000027312126, 1.666127454062681368 ) ) ;
#32699=EDGE_CURVE ( 'NONE', #41738, #35585, #21014, .T. ) ;
#32712=CARTESIAN_POINT ( 'NONE',  ( -54.64476657466781973, -131.8125000013656063, -4.444560631937228834 ) ) ;
#32721=( BOUNDED_CURVE ( )  B_SPLINE_CURVE ( 2, ( #62543, #22983, #51931, #16332, #57083, #47723, #47416, #7872, #27476 ),
 .UNSPECIFIED., .F., .F. ) 
 B_SPLINE_CURVE_WITH_KNOTS ( ( 3, 2, 2, 2, 3 ),
 ( 0.4416666666666670404, 0.4458333333333337478, 0.4500000000000003997, 0.4541666666666671071, 0.4583333333333337589 ),
 .UNSPECIFIED. ) 
 CURVE ( )  GEOMETRIC_REPRESENTATION_ITEM ( )  RATIONAL_B_SPLINE_CURVE ( ( 0.9999999999999928946, 0.9238795325112938439, 1.000000000000000000, 0.9238795325112867385, 1.000000000000000000, 0.9238795325112867385, 1.000000000000000000, 0.9238795325112786339, 1.000000000000008216 ) ) 
 REPRESENTATION_ITEM ( '' )  );
#32722=CARTESIAN_POINT ( 'NONE',  ( -51.60603307380591787, -128.1875000013656063, -2.891590998281053704 ) ) ;
#32744=EDGE_LOOP ( 'NONE', ( #15353, #47838, #26590, #1216 ) ) ;
#32748=PRODUCT_DEFINITION ( 'UNKNOWN', '', #16439, #28784 ) ;
#32750=CARTESIAN_POINT ( 'NONE',  ( -50.40829686548195099, -137.0000000013655779, -1.485763867205728284 ) ) ;
#32755=ORIENTED_EDGE ( 'NONE', *, *, #19406, .F. ) ;
#32756=CARTESIAN_POINT ( 'NONE',  ( -50.01589407740564042, -150.6250000000000284, 0.3983568153799778022 ) ) ;
#32765=CARTESIAN_POINT ( 'NONE',  ( -57.19623071787016499, -151.6250000013655779, 4.297418129356382899 ) ) ;
#32766=CARTESIAN_POINT ( 'NONE',  ( -51.75738570946856498, -140.8750000027312126, 3.805975901505576964 ) ) ;
#32773=CARTESIAN_POINT ( 'NONE',  ( -52.80376928212989185, -136.8750000013656063, -4.297418129356379346 ) ) ;
#32775=EDGE_CURVE ( 'NONE', #11538, #36394, #21239, .T. ) ;
#32781=ORIENTED_EDGE ( 'NONE', *, *, #50397, .F. ) ;
#32792=CARTESIAN_POINT ( 'NONE',  ( -52.10840900171896806, -144.1875000013656063, 3.393966926194110556 ) ) ;
#32802=CARTESIAN_POINT ( 'NONE',  ( -51.75738570946856498, -148.8750000027312126, 3.805975901505576964 ) ) ;
#32834=CARTESIAN_POINT ( 'NONE',  ( -58.39396692619412477, -129.6875000013656063, 2.891590998281057701 ) ) ;
#32842=CARTESIAN_POINT ( 'NONE',  ( -51.19402409849444524, -153.6250000027312126, -3.242614290531456334 ) ) ;
#32874=CARTESIAN_POINT ( 'NONE',  ( -53.33387254593719717, -144.9375000027312410, 5.149110718188530278 ) ) ;
#32878=CARTESIAN_POINT ( 'NONE',  ( -50.40829686548195099, -135.2500000013656347, -1.485763867205728284 ) ) ;
#32880=CARTESIAN_POINT ( 'NONE',  ( -54.60164318462004474, -145.3750000000000284, -4.984105922594373794 ) ) ;
#32912=CARTESIAN_POINT ( 'NONE',  ( -59.44456063193725015, -141.8125000013656063, -0.3552334253322034230 ) ) ;
#32916=CARTESIAN_POINT ( 'NONE',  ( -57.46284108482265651, -148.0625000027312126, 4.819101127000238627 ) ) ;
#32923=VECTOR ( 'NONE', #20465, 1000.000000000000000 ) ;
#32930=CARTESIAN_POINT ( 'NONE',  ( -52.10840900171896806, -145.1875000013656063, 3.393966926194110556 ) ) ;
#32954=CARTESIAN_POINT ( 'NONE',  ( -50.40829686548195099, -149.2500000013655779, -1.485763867205728284 ) ) ;
#32960=CARTESIAN_POINT ( 'NONE',  ( -58.24261429053147765, -136.3750000027312126, -3.805975901505573855 ) ) ;
#32965=MECHANICAL_DESIGN_GEOMETRIC_PRESENTATION_REPRESENTATION('',(#34979),#20618);
#32978=ORIENTED_EDGE ( 'NONE', *, *, #14581, .T. ) ;
#32988=EDGE_CURVE ( 'NONE', #49453, #46511, #30773, .T. ) ;
#32994=CARTESIAN_POINT ( 'NONE',  ( -57.46284108482265651, -138.9375000000000000, 4.819101127000239515 ) ) ;
#32996=VERTEX_POINT ( 'NONE', #5698 ) ;
#33001=ORIENTED_EDGE ( 'NONE', *, *, #14600, .T. ) ;
#33002=CARTESIAN_POINT ( 'NONE',  ( -54.64476657466781973, -139.0625000013656063, -4.444560631937228834 ) ) ;
#33004=CARTESIAN_POINT ( 'NONE',  ( -55.39835681537999790, -127.0000000027312126, 4.984105922594378235 ) ) ;
#33018=CARTESIAN_POINT ( 'NONE',  ( -55.35523342533222291, -125.3125000013655921, 4.444560631937231499 ) ) ;
#33030=CARTESIAN_POINT ( 'NONE',  ( -54.64476657466781973, -129.8125000013656063, -4.444560631937228834 ) ) ;
#33041=CARTESIAN_POINT ( 'NONE',  ( -51.60603307380591787, -125.1875000013656063, -2.891590998281053704 ) ) ;
#33057=CARTESIAN_POINT ( 'NONE',  ( -58.24261429053147765, -144.3750000027312126, -3.805975901505573855 ) ) ;
#33066=CARTESIAN_POINT ( 'NONE',  ( -56.48576386720575471, -154.0000000013655779, -4.591703134518078322 ) ) ;
#33076=CARTESIAN_POINT ( 'NONE',  ( -53.33387254593733928, -147.8125000000000000, 5.149110718188519620 ) ) ;
#33084=CARTESIAN_POINT ( 'NONE',  ( -50.55543936806279248, -152.3125000013656063, 0.3552334253322060320 ) ) ;
#33085=CARTESIAN_POINT ( 'NONE',  ( -56.66612745406270335, -142.4375000027312126, -5.149110718188516067 ) ) ;
#33092=CARTESIAN_POINT ( 'NONE',  ( -59.44456063193725015, -137.5625000013656063, -0.3552334253322034230 ) ) ;
#33108=CARTESIAN_POINT ( 'NONE',  ( -52.10840900171896806, -143.1875000013656063, 3.393966926194110556 ) ) ;
#33146=EDGE_LOOP ( 'NONE', ( #21976, #19934, #23966, #6930 ) ) ;
#33147=CARTESIAN_POINT ( 'NONE',  ( -56.48576386720575471, -153.7500000013656063, -4.591703134518078322 ) ) ;
#33155=CARTESIAN_POINT ( 'NONE',  ( -59.29741812935640155, -132.8750000013656063, -2.196230717870135685 ) ) ;
#33164=CARTESIAN_POINT ( 'NONE',  ( -58.80597590150559739, -154.1250000027312126, 3.242614290531460330 ) ) ;
#33181=CARTESIAN_POINT ( 'NONE',  ( -53.33387254593719717, -144.8125000000000000, 5.149110718188530278 ) ) ;
#33196=CARTESIAN_POINT ( 'NONE',  ( -50.70258187064364108, -134.3750000013656347, 2.196230717870141014 ) ) ;
#33224=CARTESIAN_POINT ( 'NONE',  ( -56.48576386720575471, -145.0000000013656063, -4.591703134518078322 ) ) ;
#33232=CARTESIAN_POINT ( 'NONE',  ( -56.66612745406278151, -150.3125000000000284, -5.149110718188523173 ) ) ;
#33242=CARTESIAN_POINT ( 'NONE',  ( -50.40829686548195099, -145.0000000013656063, -1.485763867205728284 ) ) ;
#33256=CARTESIAN_POINT ( 'NONE',  ( -51.75738570946856498, -139.7500000000000000, 3.805975901505576964 ) ) ;
#33268=CARTESIAN_POINT ( 'NONE',  ( -54.64476657466781973, -146.0625000013656063, -4.444560631937228834 ) ) ;
#33274=CARTESIAN_POINT ( 'NONE',  ( -58.80597590150559739, -148.0000000000000284, 3.242614290531460330 ) ) ;
#33278=VERTEX_POINT ( 'NONE', #24205 ) ;
#33299=FACE_OUTER_BOUND ( 'NONE', #58063, .T. ) ;
#33303=CARTESIAN_POINT ( 'NONE',  ( -59.81910112700025905, -135.1875000000000284, -2.462841084822630311 ) ) ;
#33310=CARTESIAN_POINT ( 'NONE',  ( -51.60603307380591787, -140.1875000013656063, -2.891590998281053704 ) ) ;
#33312=CARTESIAN_POINT ( 'NONE',  ( -50.01589407740564042, -124.7500000027311984, 0.3983568153799778022 ) ) ;
#33322=CYLINDRICAL_SURFACE ( 'NONE', #3128, 5.000000000000000000 ) ;
#33338=CARTESIAN_POINT ( 'NONE',  ( -59.44456063193725015, -131.5625000013656063, -0.3552334253322034230 ) ) ;
#33340=CARTESIAN_POINT ( 'NONE',  ( -59.59170313451810586, -145.5000000013656063, 1.485763867205729394 ) ) ;
#33343=ADVANCED_FACE ( 'NONE', ( #44128 ), #408, .F. ) ;
#33351=CARTESIAN_POINT ( 'NONE',  ( -58.39396692619412477, -125.6875000013656063, 2.891590998281057701 ) ) ;
#33357=CARTESIAN_POINT ( 'NONE',  ( -58.24261429053147765, -155.0000000000000284, -3.805975901505573411 ) ) ;
#33369=EDGE_CURVE ( 'NONE', #2645, #10962, #38646, .T. ) ;
#33372=CARTESIAN_POINT ( 'NONE',  ( -59.59170313451811296, -151.7500000013655779, 1.485763867205729394 ) ) ;
#33381=CARTESIAN_POINT ( 'NONE',  ( -49.85088928181150436, -147.5625000000000000, -1.666127454062680702 ) ) ;
#33384=ORIENTED_EDGE ( 'NONE', *, *, #44158, .F. ) ;
#33390=CARTESIAN_POINT ( 'NONE',  ( -58.39396692619412477, -150.6875000013656063, 2.891590998281057701 ) ) ;
#33391=CARTESIAN_POINT ( 'NONE',  ( -53.33387254593733928, -137.9375000027311842, 5.149110718188519620 ) ) ;
#33401=CARTESIAN_POINT ( 'NONE',  ( -57.89159099828107458, -131.6875000013656063, -3.393966926194107447 ) ) ;
#33416=CARTESIAN_POINT ( 'NONE',  ( -57.89159099828107458, -140.6875000013656063, -3.393966926194107447 ) ) ;
#33456=CARTESIAN_POINT ( 'NONE',  ( -59.44456063193725015, -132.8125000013656063, -0.3552334253322034230 ) ) ;
#33464=CARTESIAN_POINT ( 'NONE',  ( -49.85088928181150436, -150.6875000027312126, -1.666127454062680702 ) ) ;
#33471=CARTESIAN_POINT ( 'NONE',  ( -55.00000000000001421, -155.0000000000000284, -8.082903768654752241 ) ) ;
#33474=DIRECTION ( 'NONE',  ( -0.6485228581062915110, 0.000000000000000000, -0.7611951803011149931 ) ) ;
#33489=CARTESIAN_POINT ( 'NONE',  ( -50.40829686548195099, -153.0000000013656063, -1.485763867205728284 ) ) ;
#33504=CARTESIAN_POINT ( 'NONE',  ( -59.98410592259440222, -145.2500000027312126, -0.3983568153799752487 ) ) ;
#33508=CARTESIAN_POINT ( 'NONE',  ( -56.48576386720575471, -137.0000000013655779, -4.591703134518078322 ) ) ;
#33515=CARTESIAN_POINT ( 'NONE',  ( -58.64957059093959657, -135.0000000000000853, -2.842749532660685752 ) ) ;
#33520=CARTESIAN_POINT ( 'NONE',  ( -51.75738570946856498, -155.0000000000000284, 3.805975901505577408 ) ) ;
#33538=CARTESIAN_POINT ( 'NONE',  ( -50.70258187064364108, -141.3750000013656063, 2.196230717870141014 ) ) ;
#33547=CARTESIAN_POINT ( 'NONE',  ( -60.14911071818854538, -143.1875000027312410, 1.666127454062681146 ) ) ;
#33553=CARTESIAN_POINT ( 'NONE',  ( -55.35523342533222291, -145.3125000013656063, 4.444560631937231499 ) ) ;
#33554=DIRECTION ( 'NONE',  ( 0.000000000000000000, 1.000000000000000000, 0.000000000000000000 ) ) ;
#33565=CARTESIAN_POINT ( 'NONE',  ( -54.60164318462004474, -142.5000000027312126, -4.984105922594373794 ) ) ;
#33579=CARTESIAN_POINT ( 'NONE',  ( -54.64476657466781973, -147.0625000013656063, -4.444560631937228834 ) ) ;
#33598=( BOUNDED_CURVE ( )  B_SPLINE_CURVE ( 2, ( #56130, #48359, #3995, #22990, #3686, #39020, #52255, #48667, #42900 ),
 .UNSPECIFIED., .F., .F. ) 
 B_SPLINE_CURVE_WITH_KNOTS ( ( 3, 2, 2, 2, 3 ),
 ( 0.4583333333333337589, 0.4625000000000004663, 0.4666666666666671182, 0.4708333333333337700, 0.4750000000000004219 ),
 .UNSPECIFIED. ) 
 CURVE ( )  GEOMETRIC_REPRESENTATION_ITEM ( )  RATIONAL_B_SPLINE_CURVE ( ( 0.9999999999999918954, 0.9238795325112948431, 1.000000000000000000, 0.9238795325112867385, 1.000000000000000000, 0.9238795325112867385, 1.000000000000000000, 0.9238795325112786339, 1.000000000000008216 ) ) 
 REPRESENTATION_ITEM ( '' )  );
#33615=DIRECTION ( 'NONE',  ( -0.6485228581062915110, 0.000000000000000000, -0.7611951803011149931 ) ) ;
#33619=CARTESIAN_POINT ( 'NONE',  ( -52.53715891517739323, -135.4375000000000284, -4.819101127000233298 ) ) ;
#33628=CARTESIAN_POINT ( 'NONE',  ( -58.24261429053147765, -125.3750000027312126, -3.805975901505573855 ) ) ;
#33630=CARTESIAN_POINT ( 'NONE',  ( -51.86629881543737497, -135.0000000000000000, 3.632629519372841287 ) ) ;
#33653=CARTESIAN_POINT ( 'NONE',  ( -59.29741812935640155, -131.6250000013655779, -2.196230717870135685 ) ) ;
#33654=CARTESIAN_POINT ( 'NONE',  ( -53.51423613279429503, -147.2500000013656063, 4.591703134518083651 ) ) ;
#33663=CARTESIAN_POINT ( 'NONE',  ( -56.48576386720575471, -125.0000000013656205, -4.591703134518078322 ) ) ;
#33676=CARTESIAN_POINT ( 'NONE',  ( -51.75738570946856498, -144.8750000027312126, 3.805975901505576964 ) ) ;
#33684=CARTESIAN_POINT ( 'NONE',  ( -54.64476657466781973, -152.0625000013656063, -4.444560631937228834 ) ) ;
#33695=CARTESIAN_POINT ( 'NONE',  ( -55.39835681537999790, -146.8750000000000284, 4.984105922594378235 ) ) ;
#33702=CARTESIAN_POINT ( 'NONE',  ( -60.14911071818854538, -135.1875000027312126, 1.666127454062681146 ) ) ;
#33704=CARTESIAN_POINT ( 'NONE',  ( -50.40829686548195099, -152.2500000013656063, -1.485763867205728284 ) ) ;
#33705=CARTESIAN_POINT ( 'NONE',  ( -58.80597590150559739, -138.1250000027312410, 3.242614290531460330 ) ) ;
#33714=CARTESIAN_POINT ( 'NONE',  ( -55.35523342533222291, -131.3125000013656063, 4.444560631937231499 ) ) ;
#33729=CARTESIAN_POINT ( 'NONE',  ( -51.60603307380591787, -139.9375000013656063, -2.891590998281053704 ) ) ;
#33741=CARTESIAN_POINT ( 'NONE',  ( -53.33387254593725402, -148.8125000000000000, 5.149110718188524949 ) ) ;
#33742=CARTESIAN_POINT ( 'NONE',  ( -55.00000000000001421, -155.0000000000000284, -8.082903768654752241 ) ) ;
#33761=ORIENTED_EDGE ( 'NONE', *, *, #52869, .T. ) ;
#33762=CARTESIAN_POINT ( 'NONE',  ( -50.70258187064364108, -154.1250000013656063, 2.196230717870141014 ) ) ;
#33770=CARTESIAN_POINT ( 'NONE',  ( -53.51423613279429503, -125.5000000013656205, 4.591703134518082763 ) ) ;
#33782=CARTESIAN_POINT ( 'NONE',  ( -52.53715891517739323, -152.5625000027312126, -4.819101127000233298 ) ) ;
#33796=DIRECTION ( 'NONE',  ( 0.000000000000000000, 0.000000000000000000, -1.000000000000000000 ) ) ;
#33800=CARTESIAN_POINT ( 'NONE',  ( -59.59170313451811296, -153.5000000013656063, 1.485763867205729394 ) ) ;
#33806=ORIENTED_EDGE ( 'NONE', *, *, #14941, .T. ) ;
#33815=CARTESIAN_POINT ( 'NONE',  ( -50.55543936806279248, -136.3125000013656063, 0.3552334253322060320 ) ) ;
#33822=CARTESIAN_POINT ( 'NONE',  ( -53.33387254593710480, -139.8125000000000284, 5.149110718188539160 ) ) ;
#33842=CARTESIAN_POINT ( 'NONE',  ( -62.00000000000001421, -135.0000000000000284, -4.041451884327373456 ) ) ;
#33846=CARTESIAN_POINT ( 'NONE',  ( -53.51423613279429503, -138.5000000013656347, 4.591703134518082763 ) ) ;
#33851=CARTESIAN_POINT ( 'NONE',  ( -58.80597590150559739, -148.1250000027312126, 3.242614290531460330 ) ) ;
#33865=CARTESIAN_POINT ( 'NONE',  ( -52.80376928212989185, -143.8750000013655779, -4.297418129356379346 ) ) ;
#33876=CARTESIAN_POINT ( 'NONE',  ( -52.53715891517739323, -142.5625000027311557, -4.819101127000233298 ) ) ;
#33889=CARTESIAN_POINT ( 'NONE',  ( -51.60603307380591787, -148.1875000013656063, -2.891590998281053704 ) ) ;
#33910=FACE_OUTER_BOUND ( 'NONE', #60038, .T. ) ;
#33924=EDGE_CURVE ( 'NONE', #32996, #27913, #28628, .T. ) ;
#33929=CARTESIAN_POINT ( 'NONE',  ( -56.66612745406270335, -132.3125000000000284, -5.149110718188516067 ) ) ;
#33939=CARTESIAN_POINT ( 'NONE',  ( -57.46284108482265651, -126.0625000027312268, 4.819101127000239515 ) ) ;
#33964=CARTESIAN_POINT ( 'NONE',  ( -51.60603307380591787, -128.9375000013656063, -2.891590998281053704 ) ) ;
#33966=CARTESIAN_POINT ( 'NONE',  ( -51.60603307380591787, -144.9375000013656063, -2.891590998281053704 ) ) ;
#33998=CARTESIAN_POINT ( 'NONE',  ( -51.60603307380591787, -153.1875000013656063, -2.891590998281053704 ) ) ;
#34008=CARTESIAN_POINT ( 'NONE',  ( -52.53715891517739323, -144.4375000000000284, -4.819101127000233298 ) ) ;
#34010=VERTEX_POINT ( 'NONE', #10914 ) ;
#34015=CARTESIAN_POINT ( 'NONE',  ( -56.48576386720575471, -146.0000000013656347, -4.591703134518078322 ) ) ;
#34016=CARTESIAN_POINT ( 'NONE',  ( -58.80597590150559739, -140.1250000027312126, 3.242614290531460330 ) ) ;
#34027=CARTESIAN_POINT ( 'NONE',  ( -56.48576386720575471, -132.7500000013656063, -4.591703134518078322 ) ) ;
#34030=CARTESIAN_POINT ( 'NONE',  ( -50.01589407740564042, -146.7500000027312126, 0.3983568153799778022 ) ) ;
#34042=CARTESIAN_POINT ( 'NONE',  ( -50.55543936806279248, -142.0625000013656063, 0.3552334253322060320 ) ) ;
#34046=CARTESIAN_POINT ( 'NONE',  ( -52.53715891517739323, -144.4375000000000000, -4.819101127000233298 ) ) ;
#34074=CARTESIAN_POINT ( 'NONE',  ( -57.89159099828107458, -151.6875000013656063, -3.393966926194107447 ) ) ;
#34080=DIRECTION ( 'NONE',  ( 0.6485228581062915110, 0.000000000000000000, 0.7611951803011149931 ) ) ;
#34081=CARTESIAN_POINT ( 'NONE',  ( -52.10840900171896806, -125.4375000013656063, 3.393966926194110556 ) ) ;
#34088=CARTESIAN_POINT ( 'NONE',  ( -59.81910112700026616, -152.1875000000000568, -2.462841084822585014 ) ) ;
#34090=CARTESIAN_POINT ( 'NONE',  ( -59.81910112700025905, -149.3125000027312126, -2.462841084822630311 ) ) ;
#34108=CARTESIAN_POINT ( 'NONE',  ( -56.48576386720575471, -153.7500000013656063, -4.591703134518078322 ) ) ;
#34123=CYLINDRICAL_SURFACE ( 'NONE', #16483, 5.000000000000000000 ) ;
#34127=EDGE_CURVE ( 'NONE', #59631, #16288, #52197, .T. ) ;
#34140=CARTESIAN_POINT ( 'NONE',  ( -51.75738570946856498, -153.8750000027312126, 3.805975901505576964 ) ) ;
#34145=CARTESIAN_POINT ( 'NONE',  ( -50.01589407740564042, -136.6250000000000284, 0.3983568153799778022 ) ) ;
#34153=CARTESIAN_POINT ( 'NONE',  ( -59.29741812935640155, -138.8750000013655779, -2.196230717870135685 ) ) ;
#34158=CARTESIAN_POINT ( 'NONE',  ( -60.14911071818854538, -148.1875000027312126, 1.666127454062681146 ) ) ;
#34171=CARTESIAN_POINT ( 'NONE',  ( -56.48576386720575471, -144.7500000013656063, -4.591703134518078322 ) ) ;
#34174=ORIENTED_EDGE ( 'NONE', *, *, #35304, .F. ) ;
#34184=CARTESIAN_POINT ( 'NONE',  ( -59.98410592259440222, -142.1250000000000284, -0.3983568153799752487 ) ) ;
#34187=( BOUNDED_CURVE ( )  B_SPLINE_CURVE ( 2, ( #60702, #41686, #16310, #6982, #36243, #26593, #35931, #55559, #11473 ),
 .UNSPECIFIED., .F., .F. ) 
 B_SPLINE_CURVE_WITH_KNOTS ( ( 3, 2, 2, 2, 3 ),
 ( 0.5583333333333337922, 0.5625000000000004441, 0.5666666666666670960, 0.5708333333333338588, 0.5750000000000005107 ),
 .UNSPECIFIED. ) 
 CURVE ( )  GEOMETRIC_REPRESENTATION_ITEM ( )  RATIONAL_B_SPLINE_CURVE ( ( 0.9999999999999918954, 0.9238795325112948431, 1.000000000000000000, 0.9238795325112867385, 1.000000000000000000, 0.9238795325112867385, 1.000000000000000000, 0.9238795325112766355, 1.000000000000010214 ) ) 
 REPRESENTATION_ITEM ( '' )  );
#34197=CARTESIAN_POINT ( 'NONE',  ( -53.51423613279429503, -143.5000000013656347, 4.591703134518082763 ) ) ;
#34224=VERTEX_POINT ( 'NONE', #12506 ) ;
#34232=CARTESIAN_POINT ( 'NONE',  ( -57.46284108482265651, -133.9375000000000000, 4.819101127000239515 ) ) ;
#34242=CARTESIAN_POINT ( 'NONE',  ( -56.66612745406270335, -127.4375000027312126, -5.149110718188516067 ) ) ;
#34270=CARTESIAN_POINT ( 'NONE',  ( -59.29741812935640155, -128.6250000013656063, -2.196230717870135685 ) ) ;
#34271=CARTESIAN_POINT ( 'NONE',  ( -54.64476657466781973, -146.8125000013656063, -4.444560631937228834 ) ) ;
#34283=CARTESIAN_POINT ( 'NONE',  ( -59.59170313451811296, -125.7500000013656347, 1.485763867205729394 ) ) ;
#34300=CARTESIAN_POINT ( 'NONE',  ( -58.24261429053147765, -148.3750000027312126, -3.805975901505573855 ) ) ;
#34306=CARTESIAN_POINT ( 'NONE',  ( -55.35523342533222291, -152.5625000013656063, 4.444560631937231499 ) ) ;
#34315=CARTESIAN_POINT ( 'NONE',  ( -54.60164318462004474, -144.3750000000000284, -4.984105922594373794 ) ) ;
#34318=( BOUNDED_CURVE ( )  B_SPLINE_CURVE ( 2, ( #12669, #34088, #14154, #53398, #7849, #24134, #28633, #42249, #56745 ),
 .UNSPECIFIED., .F., .F. ) 
 B_SPLINE_CURVE_WITH_KNOTS ( ( 3, 2, 2, 2, 3 ),
 ( 0.09166666666666674346, 0.09583333333333342308, 0.1000000000000000888, 0.1041666666666667546, 0.1083333333333334203 ),
 .UNSPECIFIED. ) 
 CURVE ( )  GEOMETRIC_REPRESENTATION_ITEM ( )  RATIONAL_B_SPLINE_CURVE ( ( 0.9999999999999984457, 0.9238795325112882928, 1.000000000000000000, 0.9238795325112867385, 1.000000000000000000, 0.9238795325112867385, 1.000000000000000000, 0.9238795325112851842, 1.000000000000001554 ) ) 
 REPRESENTATION_ITEM ( '' )  );
#34324=CARTESIAN_POINT ( 'NONE',  ( -55.35523342533222291, -146.5625000013656063, 4.444560631937231499 ) ) ;
#34325=CARTESIAN_POINT ( 'NONE',  ( -55.39835681537999790, -140.0000000027312126, 4.984105922594378235 ) ) ;
#34332=VECTOR ( 'NONE', #25060, 1000.000000000000000 ) ;
#34338=CARTESIAN_POINT ( 'NONE',  ( -55.35523342533222291, -134.3125000013656063, 4.444560631937231499 ) ) ;
#34351=CARTESIAN_POINT ( 'NONE',  ( -50.70258187064364108, -140.1250000013655779, 2.196230717870141014 ) ) ;
#34374=AXIS2_PLACEMENT_3D ( 'NONE', #15432, #54663, #6103 ) ;
#34383=CARTESIAN_POINT ( 'NONE',  ( -50.40829686548195099, -154.0000000013656063, -1.485763867205728284 ) ) ;
#34391=CARTESIAN_POINT ( 'NONE',  ( -56.48576386720575471, -126.0000000013656063, -4.591703134518078322 ) ) ;
#34399=CARTESIAN_POINT ( 'NONE',  ( -59.81910112700025905, -151.3125000027312126, -2.462841084822630311 ) ) ;
#34412=CARTESIAN_POINT ( 'NONE',  ( -55.39835681537999790, -154.0000000027312410, 4.984105922594378235 ) ) ;
#34417=CARTESIAN_POINT ( 'NONE',  ( -52.10840900171896806, -153.1875000013656063, 3.393966926194110556 ) ) ;
#34419=DIRECTION ( 'NONE',  ( -0.6485228581062915110, 0.000000000000000000, -0.7611951803011149931 ) ) ;
#34440=CARTESIAN_POINT ( 'NONE',  ( -59.04365660845520836, -135.0000000000000284, 2.932170451817831758 ) ) ;
#34462=CARTESIAN_POINT ( 'NONE',  ( -50.55543936806279248, -139.3125000013656063, 0.3552334253322060320 ) ) ;
#34478=CARTESIAN_POINT ( 'NONE',  ( -51.60603307380591787, -140.9375000013656063, -2.891590998281053704 ) ) ;
#34504=CARTESIAN_POINT ( 'NONE',  ( -50.70258187064364108, -143.3750000013656063, 2.196230717870141014 ) ) ;
#34507=LINE ( 'NONE', #45451, #11064 ) ;
#34537=ORIENTED_EDGE ( 'NONE', *, *, #21754, .T. ) ;
#34545=CARTESIAN_POINT ( 'NONE',  ( -54.60164318462004474, -134.3750000000000284, -4.984105922594373794 ) ) ;
#34558=CARTESIAN_POINT ( 'NONE',  ( -51.60603307380591787, -153.9375000013656063, -2.891590998281053704 ) ) ;
#34560=CARTESIAN_POINT ( 'NONE',  ( -51.14619162160809651, -135.0000000000000284, 2.724453935955323480 ) ) ;
#34583=CARTESIAN_POINT ( 'NONE',  ( -58.39396692619412477, -124.4375000013656063, 2.891590998281057701 ) ) ;
#34584=CARTESIAN_POINT ( 'NONE',  ( -57.89159099828107458, -147.6875000013656063, -3.393966926194107447 ) ) ;
#34623=CARTESIAN_POINT ( 'NONE',  ( -59.59170313451811296, -149.7500000013656063, 1.485763867205729394 ) ) ;
#34634=CARTESIAN_POINT ( 'NONE',  ( -58.80597590150559739, -144.0000000000000284, 3.242614290531460330 ) ) ;
#34645=CARTESIAN_POINT ( 'NONE',  ( -59.44456063193725015, -146.8125000013656063, -0.3552334253322034230 ) ) ;
#34647=CARTESIAN_POINT ( 'NONE',  ( -57.46284108482265651, -138.0625000027311842, 4.819101127000239515 ) ) ;
#34664=CARTESIAN_POINT ( 'NONE',  ( -54.64476657466781973, -132.8125000013656063, -4.444560631937228834 ) ) ;
#34679=CARTESIAN_POINT ( 'NONE',  ( -59.59170313451811296, -136.5000000013656347, 1.485763867205729394 ) ) ;
#34689=CYLINDRICAL_SURFACE ( 'NONE', #31774, 5.000000000000000000 ) ;
#34708=EDGE_LOOP ( 'NONE', ( #28199, #36532, #29942, #39613 ) ) ;
#34712=ORIENTED_EDGE ( 'NONE', *, *, #8713, .F. ) ;
#34713=CARTESIAN_POINT ( 'NONE',  ( -52.10840900171896806, -149.1875000013656063, 3.393966926194110556 ) ) ;
#34720=CARTESIAN_POINT ( 'NONE',  ( -57.89159099828107458, -127.9375000013656063, -3.393966926194107447 ) ) ;
#34727=CARTESIAN_POINT ( 'NONE',  ( -60.14911071818854538, -150.0625000000000000, 1.666127454062681146 ) ) ;
#34732=CARTESIAN_POINT ( 'NONE',  ( -60.14911071818854538, -151.1875000027312126, 1.666127454062681368 ) ) ;
#34754=CARTESIAN_POINT ( 'NONE',  ( -59.29741812935640155, -149.6250000013655779, -2.196230717870135685 ) ) ;
#34756=FACE_OUTER_BOUND ( 'NONE', #19943, .T. ) ;
#34776=DIRECTION ( 'NONE',  ( 1.000000000000000000, 0.000000000000000000, -0.000000000000000000 ) ) ;
#34787=B_SPLINE_CURVE_WITH_KNOTS ( 'NONE', 3,
 ( #24930, #14950, #14319, #53562, #43890, #63538, #9185, #18825, #58071, #59019, #29098, #38444, #34560, #14003, #14631, #33630, #48413, #54191, #48724, #19780, #53249, #52934, #44215, #53873, #63222 ),
 .UNSPECIFIED., .F., .F.,
 ( 4, 2, 2, 2, 2, 1, 2, 2, 2, 2, 2, 2, 4 ),
 ( 1.525486860402933621E-14, 0.001159901942158824556, 0.001739852913230607954, 0.002319803884302391352, 0.002899754855374174316, 0.003479705826445958147, 0.004059656797517741111, 0.004639607768589523208, 0.005799509710733074391, 0.006959411652876625574, 0.007539362623948399865, 0.008119313595020176758, 0.009279215537163704522 ),
 .UNSPECIFIED. ) ;
#34803=CARTESIAN_POINT ( 'NONE',  ( -59.59170313451811296, -139.7500000013656347, 1.485763867205729394 ) ) ;
#34808=ORIENTED_EDGE ( 'NONE', *, *, #31816, .T. ) ;
#34822=CARTESIAN_POINT ( 'NONE',  ( -59.44456063193725015, -140.5625000013656063, -0.3552334253322034230 ) ) ;
#34838=PRODUCT_DEFINITION_SHAPE ( 'NONE', 'NONE',  #32748 ) ;
#34850=CARTESIAN_POINT ( 'NONE',  ( -59.59170313451811296, -145.7500000013655779, 1.485763867205729394 ) ) ;
#34856=DIRECTION ( 'NONE',  ( 0.000000000000000000, 1.000000000000000000, 0.000000000000000000 ) ) ;
#34870=CARTESIAN_POINT ( 'NONE',  ( -50.18089887299977647, -145.8125000027311842, 2.462841084822515292 ) ) ;
#34874=CARTESIAN_POINT ( 'NONE',  ( -55.39835681537999790, -150.8750000000000284, 4.984105922594378235 ) ) ;
#34889=CARTESIAN_POINT ( 'NONE',  ( -50.18089887299979068, -128.6875000000000284, 2.462841084822635640 ) ) ;
#34897=CARTESIAN_POINT ( 'NONE',  ( -59.44456063193725015, -151.5625000013656063, -0.3552334253322034230 ) ) ;
#34904=( BOUNDED_CURVE ( )  B_SPLINE_CURVE ( 2, ( #43847, #63493, #48995, #47744, #33274, #3700, #23315, #62563, #8829 ),
 .UNSPECIFIED., .F., .T. ) 
 B_SPLINE_CURVE_WITH_KNOTS ( ( 3, 2, 2, 2, 3 ),
 ( 0.2250000000000001998, 0.2291666666666668517, 0.2333333333333335313, 0.2375000000000001832, 0.2416666666666668628 ),
 .UNSPECIFIED. ) 
 CURVE ( )  GEOMETRIC_REPRESENTATION_ITEM ( )  RATIONAL_B_SPLINE_CURVE ( ( 0.9999999999999964473, 0.9238795325112902912, 1.000000000000000000, 0.9238795325112867385, 1.000000000000000000, 0.9238795325112867385, 1.000000000000000000, 0.9238795325112831858, 1.000000000000003553 ) ) 
 REPRESENTATION_ITEM ( '' )  );
#34911=CARTESIAN_POINT ( 'NONE',  ( -55.00000000000001421, -135.0000000000000284, 8.082903768654762899 ) ) ;
#34922=CARTESIAN_POINT ( 'NONE',  ( -54.64476657466781973, -154.0625000013656347, -4.444560631937228834 ) ) ;
#34923=CARTESIAN_POINT ( 'NONE',  ( -51.60603307380591787, -143.9375000013656063, -2.891590998281053704 ) ) ;
#34957=CARTESIAN_POINT ( 'NONE',  ( -58.39396692619412477, -146.6875000013656063, 2.891590998281057701 ) ) ;
#34968=ORIENTED_EDGE ( 'NONE', *, *, #20327, .T. ) ;
#34969=CARTESIAN_POINT ( 'NONE',  ( -50.01589407740564042, -140.6250000000000284, 0.3983568153799778022 ) ) ;
#34978=CARTESIAN_POINT ( 'NONE',  ( -50.70258187064364108, -147.3750000013656063, 2.196230717870141014 ) ) ;
#34979=STYLED_ITEM('',(#63698),#28816);
#34981=CARTESIAN_POINT ( 'NONE',  ( -56.66612745406270335, -133.4375000027312126, -5.149110718188516067 ) ) ;
#34986=CARTESIAN_POINT ( 'NONE',  ( -59.98410592259440222, -135.1250000000000284, -0.3983568153799752487 ) ) ;
#34993=CARTESIAN_POINT ( 'NONE',  ( -59.29741812935640155, -130.6250000013656347, -2.196230717870135685 ) ) ;
#35004=CARTESIAN_POINT ( 'NONE',  ( -54.60164318462004474, -143.5000000027312126, -4.984105922594373794 ) ) ;
#35009=CARTESIAN_POINT ( 'NONE',  ( -52.10840900171896806, -137.1875000013656063, 3.393966926194110556 ) ) ;
#35019=CARTESIAN_POINT ( 'NONE',  ( -53.51423613279429503, -130.5000000013656063, 4.591703134518082763 ) ) ;
#35025=EDGE_CURVE ( 'NONE', #24115, #17875, #9101, .T. ) ;
#35045=CARTESIAN_POINT ( 'NONE',  ( -56.48576386720575471, -150.7500000013655779, -4.591703134518078322 ) ) ;
#35052=CARTESIAN_POINT ( 'NONE',  ( -52.80376928212989185, -126.1250000013656205, -4.297418129356379346 ) ) ;
#35060=FACE_OUTER_BOUND ( 'NONE', #59074, .T. ) ;
#35062=CARTESIAN_POINT ( 'NONE',  ( -50.01589407740564042, -147.7500000027312126, 0.3983568153799778022 ) ) ;
#35078=CARTESIAN_POINT ( 'NONE',  ( -57.89159099828107458, -148.6875000013656063, -3.393966926194107447 ) ) ;
#35084=FACE_OUTER_BOUND ( 'NONE', #12585, .T. ) ;
#35087=ORIENTED_EDGE ( 'NONE', *, *, #43472, .T. ) ;
#35111=EDGE_CURVE ( 'NONE', #25453, #44367, #14789, .T. ) ;
#35130=CARTESIAN_POINT ( 'NONE',  ( -58.39396692619412477, -137.6875000013656063, 2.891590998281057701 ) ) ;
#35137=CYLINDRICAL_SURFACE ( 'NONE', #39929, 5.000000000000000000 ) ;
#35140=LINE ( 'NONE', #6189, #54790 ) ;
#35147=CARTESIAN_POINT ( 'NONE',  ( -52.80376928212989185, -140.8750000013656063, -4.297418129356379346 ) ) ;
#35173=CARTESIAN_POINT ( 'NONE',  ( -57.19623071787017210, -145.6250000013655779, 4.297418129356382899 ) ) ;
#35199=CARTESIAN_POINT ( 'NONE',  ( -51.19402409849444524, -135.6250000027312410, -3.242614290531456334 ) ) ;
#35205=ORIENTED_EDGE ( 'NONE', *, *, #16429, .T. ) ;
#35208=VERTEX_POINT ( 'NONE', #15833 ) ;
#35210=CARTESIAN_POINT ( 'NONE',  ( -55.39835681537999790, -129.8750000000000284, 4.984105922594378235 ) ) ;
#35217=CARTESIAN_POINT ( 'NONE',  ( -59.29741812935640155, -153.6250000013655779, -2.196230717870135685 ) ) ;
#35242=CARTESIAN_POINT ( 'NONE',  ( -50.55543936806279248, -126.0625000013655921, 0.3552334253322060320 ) ) ;
#35243=CARTESIAN_POINT ( 'NONE',  ( -57.89159099828107458, -143.6875000013656063, -3.393966926194107447 ) ) ;
#35269=AXIS2_PLACEMENT_3D ( 'NONE', #4134, #13147, #62048 ) ;
#35280=CARTESIAN_POINT ( 'NONE',  ( -50.18089887299979068, -141.6875000000000000, 2.462841084822635640 ) ) ;
#35291=CARTESIAN_POINT ( 'NONE',  ( -50.55543936806279248, -148.3125000013656063, 0.3552334253322060320 ) ) ;
#35293=CARTESIAN_POINT ( 'NONE',  ( -60.14911071818854538, -133.1875000027312126, 1.666127454062681368 ) ) ;
#35304=EDGE_CURVE ( 'NONE', #44139, #47814, #35140, .T. ) ;
#35307=CARTESIAN_POINT ( 'NONE',  ( -59.44456063193725015, -129.5625000013656063, -0.3552334253322034230 ) ) ;
#35321=CARTESIAN_POINT ( 'NONE',  ( -59.29741812935640155, -139.6250000013655779, -2.196230717870135685 ) ) ;
#35330=CARTESIAN_POINT ( 'NONE',  ( -51.60603307380591787, -132.1875000013656063, -2.891590998281053704 ) ) ;
#35334=CARTESIAN_POINT ( 'NONE',  ( -55.00000000000002132, -155.0000000000000284, 1.734723475976807094E-15 ) ) ;
#35343=( BOUNDED_CURVE ( )  B_SPLINE_CURVE ( 2, ( #54718, #44092, #19974, #35411, #20301, #40235, #49874, #4866, #59546 ),
 .UNSPECIFIED., .F., .F. ) 
 B_SPLINE_CURVE_WITH_KNOTS ( ( 3, 2, 2, 2, 3 ),
 ( 0.07500000000000005274, 0.07916666666666671848, 0.08333333333333339810, 0.08750000000000007772, 0.09166666666666674346 ),
 .UNSPECIFIED. ) 
 CURVE ( )  GEOMETRIC_REPRESENTATION_ITEM ( )  RATIONAL_B_SPLINE_CURVE ( ( 0.9999999999999990008, 0.9238795325112877377, 1.000000000000000000, 0.9238795325112867385, 1.000000000000000000, 0.9238795325112867385, 1.000000000000000000, 0.9238795325112851842, 1.000000000000001554 ) ) 
 REPRESENTATION_ITEM ( '' )  );
#35354=CARTESIAN_POINT ( 'NONE',  ( -54.64476657466781973, -150.8125000013656063, -4.444560631937228834 ) ) ;
#35359=CARTESIAN_POINT ( 'NONE',  ( -57.46284108482265651, -151.9375000000000284, 4.819101127000239515 ) ) ;
#35371=CARTESIAN_POINT ( 'NONE',  ( -58.80597590150559739, -146.1250000027312126, 3.242614290531460330 ) ) ;
#35392=CARTESIAN_POINT ( 'NONE',  ( -59.29741812935640155, -151.6250000013656063, -2.196230717870135685 ) ) ;
#35397=CARTESIAN_POINT ( 'NONE',  ( -55.00000000000002132, -155.0000000000000284, 1.734723475976807094E-15 ) ) ;
#35411=CARTESIAN_POINT ( 'NONE',  ( -49.85088928181150436, -151.6875000027311842, -1.666127454062680480 ) ) ;
#35436=CARTESIAN_POINT ( 'NONE',  ( -57.89159099828107458, -134.9375000013656063, -3.393966926194107447 ) ) ;
#35460=CARTESIAN_POINT ( 'NONE',  ( -59.59170313451811296, -142.5000000013656347, 1.485763867205729394 ) ) ;
#35488=CARTESIAN_POINT ( 'NONE',  ( -58.39396692619412477, -142.6875000013656063, 2.891590998281057701 ) ) ;
#35502=CARTESIAN_POINT ( 'NONE',  ( -52.53715891517739323, -138.5625000027311842, -4.819101127000233298 ) ) ;
#35521=CARTESIAN_POINT ( 'NONE',  ( -59.81910112700027327, -149.3125000027312126, -2.462841084822540605 ) ) ;
#35527=CARTESIAN_POINT ( 'NONE',  ( -49.85088928181150436, -128.5625000000000568, -1.666127454062680702 ) ) ;
#35535=CARTESIAN_POINT ( 'NONE',  ( -56.48576386720575471, -151.7500000013655779, -4.591703134518078322 ) ) ;
#35562=CARTESIAN_POINT ( 'NONE',  ( -56.48576386720575471, -125.7500000013656347, -4.591703134518078322 ) ) ;
#35563=CARTESIAN_POINT ( 'NONE',  ( -58.39396692619412477, -143.4375000013656063, 2.891590998281057701 ) ) ;
#35585=VERTEX_POINT ( 'NONE', #42483 ) ;
#35603=CARTESIAN_POINT ( 'NONE',  ( -59.98410592259440222, -142.1250000000000284, -0.3983568153799752487 ) ) ;
#35612=CARTESIAN_POINT ( 'NONE',  ( -52.10840900171896806, -142.4375000013656063, 3.393966926194110556 ) ) ;
#35614=CARTESIAN_POINT ( 'NONE',  ( -50.18089887299979068, -132.8125000027312126, 2.462841084822635640 ) ) ;
#35627=CARTESIAN_POINT ( 'NONE',  ( -57.19623071787017210, -129.3750000013656347, 4.297418129356382899 ) ) ;
#35640=CIRCLE ( 'NONE', #14039, 5.000000000000000000 ) ;
#35644=CARTESIAN_POINT ( 'NONE',  ( -58.39396692619412477, -139.4375000013656063, 2.891590998281057701 ) ) ;
#35654=CARTESIAN_POINT ( 'NONE',  ( -51.60603307380591787, -130.1875000013656063, -2.891590998281053704 ) ) ;
#35667=DIRECTION ( 'NONE',  ( -0.6485228581062915110, 0.000000000000000000, -0.7611951803011149931 ) ) ;
#35680=CARTESIAN_POINT ( 'NONE',  ( -50.40829686548195099, -149.0000000013656063, -1.485763867205728284 ) ) ;
#35688=CARTESIAN_POINT ( 'NONE',  ( -58.24261429053147765, -152.2500000000000284, -3.805975901505573855 ) ) ;
#35699=CARTESIAN_POINT ( 'NONE',  ( -52.53715891517739323, -147.5625000027312126, -4.819101127000233298 ) ) ;
#35715=CARTESIAN_POINT ( 'NONE',  ( -59.59170313451811296, -150.5000000013655779, 1.485763867205729394 ) ) ;
#35761=CARTESIAN_POINT ( 'NONE',  ( -57.89159099828107458, -133.9375000013656063, -3.393966926194107447 ) ) ;
#35807=CARTESIAN_POINT ( 'NONE',  ( -50.70258187064364108, -138.3750000013656063, 2.196230717870141014 ) ) ;
#35828=CARTESIAN_POINT ( 'NONE',  ( -55.00000000000002132, -155.0000000000000284, 1.734723475976807094E-15 ) ) ;
#35850=CARTESIAN_POINT ( 'NONE',  ( -51.19402409849444524, -128.5000000000000284, -3.242614290531456334 ) ) ;
#35858=CARTESIAN_POINT ( 'NONE',  ( -55.35523342533222291, -154.3125000013656347, 4.444560631937231499 ) ) ;
#35882=CARTESIAN_POINT ( 'NONE',  ( -56.48576386720575471, -152.0000000013655779, -4.591703134518078322 ) ) ;
#35883=CARTESIAN_POINT ( 'NONE',  ( -51.60603307380591787, -140.9375000013656063, -2.891590998281053704 ) ) ;
#35924=CARTESIAN_POINT ( 'NONE',  ( -49.85088928181150436, -142.5625000000000284, -1.666127454062680702 ) ) ;
#35931=CARTESIAN_POINT ( 'NONE',  ( -55.39835681537999790, -137.0000000027312126, 4.984105922594378235 ) ) ;
#35934=CARTESIAN_POINT ( 'NONE',  ( -50.70258187064364108, -143.3750000013656063, 2.196230717870141014 ) ) ;
#35936=CARTESIAN_POINT ( 'NONE',  ( -49.85088928181150436, -132.6875000027312410, -1.666127454062680702 ) ) ;
#35949=CARTESIAN_POINT ( 'NONE',  ( -50.40829686548195099, -130.0000000013656063, -1.485763867205728284 ) ) ;
#35964=CARTESIAN_POINT ( 'NONE',  ( -50.70258187064364108, -138.1250000013656063, 2.196230717870141014 ) ) ;
#35974=CARTESIAN_POINT ( 'NONE',  ( -51.60603307380591787, -131.1875000013656063, -2.891590998281053704 ) ) ;
#35978=CYLINDRICAL_SURFACE ( 'NONE', #12312, 5.000000000000000000 ) ;
#35986=DIRECTION ( 'NONE',  ( -0.8660254037844384856, 0.000000000000000000, 0.5000000000000001110 ) ) ;
#36001=CARTESIAN_POINT ( 'NONE',  ( -51.75738570946856498, -155.0000000000000284, 3.805975901505577408 ) ) ;
#36004=CARTESIAN_POINT ( 'NONE',  ( -58.39396692619412477, -124.6875000013656063, 2.891590998281057701 ) ) ;
#36012=CARTESIAN_POINT ( 'NONE',  ( -53.51423613279429503, -152.5000000013655779, 4.591703134518083651 ) ) ;
#36014=CARTESIAN_POINT ( 'NONE',  ( -52.53715891517739323, -148.5625000027312126, -4.819101127000233298 ) ) ;
#36033=CARTESIAN_POINT ( 'NONE',  ( -53.51423613279429503, -150.2500000013656063, 4.591703134518082763 ) ) ;
#36077=CARTESIAN_POINT ( 'NONE',  ( -59.29741812935640155, -134.8750000013656063, -2.196230717870135685 ) ) ;
#36082=CARTESIAN_POINT ( 'NONE',  ( -53.50367810914265476, -135.0000000000000000, -4.210172938645351692 ) ) ;
#36122=CARTESIAN_POINT ( 'NONE',  ( -52.10840900171896806, -140.4375000013656063, 3.393966926194110556 ) ) ;
#36143=CARTESIAN_POINT ( 'NONE',  ( -57.19623071787016499, -136.6250000013656063, 4.297418129356382899 ) ) ;
#36156=CARTESIAN_POINT ( 'NONE',  ( -57.19623071787017210, -146.6250000013656063, 4.297418129356382899 ) ) ;
#36167=CARTESIAN_POINT ( 'NONE',  ( -53.33387254593733928, -128.8125000000000568, 5.149110718188519620 ) ) ;
#36176=CARTESIAN_POINT ( 'NONE',  ( -50.55543936806279248, -148.0625000013656063, 0.3552334253322060320 ) ) ;
#36199=CARTESIAN_POINT ( 'NONE',  ( -59.59170313451811296, -152.7500000013655779, 1.485763867205729394 ) ) ;
#36200=CARTESIAN_POINT ( 'NONE',  ( -50.55543936806279248, -144.0625000013656063, 0.3552334253322060320 ) ) ;
#36203=CARTESIAN_POINT ( 'NONE',  ( -52.53715891517739323, -153.5625000027312126, -4.819101127000233298 ) ) ;
#36235=CARTESIAN_POINT ( 'NONE',  ( -58.80597590150559739, -141.0000000000000000, 3.242614290531460330 ) ) ;
#36243=CARTESIAN_POINT ( 'NONE',  ( -58.80597590150559739, -137.1250000027312410, 3.242614290531460330 ) ) ;
#36247=CARTESIAN_POINT ( 'NONE',  ( -54.64476657466781973, -141.0625000013656063, -4.444560631937228834 ) ) ;
#36249=CARTESIAN_POINT ( 'NONE',  ( -55.39835681537999790, -134.0000000027312126, 4.984105922594378235 ) ) ;
#36263=CARTESIAN_POINT ( 'NONE',  ( -57.19623071787017210, -130.3750000013656631, 4.297418129356382899 ) ) ;
#36266=CARTESIAN_POINT ( 'NONE',  ( -55.39835681537999790, -142.0000000027312126, 4.984105922594378235 ) ) ;
#36279=CARTESIAN_POINT ( 'NONE',  ( -52.80376928212989185, -134.8750000013656063, -4.297418129356379346 ) ) ;
#36289=CARTESIAN_POINT ( 'NONE',  ( -50.55543936806279248, -133.3125000013656063, 0.3552334253322060320 ) ) ;
#36312=ORIENTED_EDGE ( 'NONE', *, *, #60309, .F. ) ;
#36314=CARTESIAN_POINT ( 'NONE',  ( -53.51423613279429503, -139.2500000013656063, 4.591703134518083651 ) ) ;
#36319=CARTESIAN_POINT ( 'NONE',  ( -59.98410592259440222, -153.1250000000000284, -0.3983568153799752487 ) ) ;
#36326=CARTESIAN_POINT ( 'NONE',  ( -53.51423613279429503, -154.5000000013655779, 4.591703134518083651 ) ) ;
#36328=CARTESIAN_POINT ( 'NONE',  ( -51.19402409849444524, -145.6250000027312126, -3.242614290531456334 ) ) ;
#36337=CARTESIAN_POINT ( 'NONE',  ( -58.24261429053147765, -146.3750000027312126, -3.805975901505573855 ) ) ;
#36346=CARTESIAN_POINT ( 'NONE',  ( -57.46284108482265651, -137.9375000000000284, 4.819101127000238627 ) ) ;
#36347=CARTESIAN_POINT ( 'NONE',  ( -59.59170313451811296, -146.5000000013656347, 1.485763867205729394 ) ) ;
#36375=VECTOR ( 'NONE', #25244, 1000.000000000000000 ) ;
#36391=CARTESIAN_POINT ( 'NONE',  ( -55.35523342533222291, -134.5625000013656063, 4.444560631937231499 ) ) ;
#36394=VERTEX_POINT ( 'NONE', #57852 ) ;
#36434=CARTESIAN_POINT ( 'NONE',  ( -53.51423613279429503, -140.5000000013656347, 4.591703134518082763 ) ) ;
#36450=ADVANCED_FACE ( 'NONE', ( #62999 ), #47252, .F. ) ;
#36454=CARTESIAN_POINT ( 'NONE',  ( -52.10840900171896806, -136.4375000013656063, 3.393966926194110556 ) ) ;
#36460=CARTESIAN_POINT ( 'NONE',  ( -57.46284108482265651, -138.9375000000000000, 4.819101127000238627 ) ) ;
#36466=CARTESIAN_POINT ( 'NONE',  ( -57.89159099828107458, -145.9375000013656063, -3.393966926194107447 ) ) ;
#36480=CARTESIAN_POINT ( 'NONE',  ( -56.66612745406270335, -127.3125000000000284, -5.149110718188516067 ) ) ;
#36486=CARTESIAN_POINT ( 'NONE',  ( -50.40829686548195099, -151.0000000013656063, -1.485763867205728284 ) ) ;
#36509=CARTESIAN_POINT ( 'NONE',  ( -56.48576386720575471, -154.0000000013655779, -4.591703134518078322 ) ) ;
#36525=CARTESIAN_POINT ( 'NONE',  ( -54.60164318462004474, -152.3750000000000284, -4.984105922594373794 ) ) ;
#36532=ORIENTED_EDGE ( 'NONE', *, *, #48322, .T. ) ;
#36538=EDGE_CURVE ( 'NONE', #47814, #25936, #53008, .T. ) ;
#36548=CARTESIAN_POINT ( 'NONE',  ( -58.24261429053147765, -138.2500000000000000, -3.805975901505573855 ) ) ;
#36558=CARTESIAN_POINT ( 'NONE',  ( -53.51423613279429503, -142.5000000013656063, 4.591703134518083651 ) ) ;
#36560=CARTESIAN_POINT ( 'NONE',  ( -58.24261429053147765, -129.3750000027312126, -3.805975901505573855 ) ) ;
#36585=CARTESIAN_POINT ( 'NONE',  ( -59.44456063193725015, -133.5625000013656063, -0.3552334253322034230 ) ) ;
#36593=ORIENTED_EDGE ( 'NONE', *, *, #15239, .F. ) ;
#36596=CARTESIAN_POINT ( 'NONE',  ( -59.59170313451811296, -126.7500000013655921, 1.485763867205729394 ) ) ;
#36621=CARTESIAN_POINT ( 'NONE',  ( -59.59170313451811296, -153.7500000013656063, 1.485763867205729394 ) ) ;
#36626=CARTESIAN_POINT ( 'NONE',  ( -59.29741812935640155, -139.6250000013655779, -2.196230717870135685 ) ) ;
#36632=CARTESIAN_POINT ( 'NONE',  ( -53.33387254593733928, -152.8125000000000284, 5.149110718188519620 ) ) ;
#36642=CARTESIAN_POINT ( 'NONE',  ( -56.66612745406270335, -144.4375000027312410, -5.149110718188516067 ) ) ;
#36651=CARTESIAN_POINT ( 'NONE',  ( -50.55543936806279248, -141.0625000013656063, 0.3552334253322060320 ) ) ;
#36666=CARTESIAN_POINT ( 'NONE',  ( -56.48576386720575471, -144.7500000013656063, -4.591703134518078322 ) ) ;
#36683=EDGE_CURVE ( 'NONE', #49700, #28303, #53953, .T. ) ;
#36686=( BOUNDED_CURVE ( )  B_SPLINE_CURVE ( 2, ( #30024, #1743, #5919, #15882, #6871, #35502, #782, #40635, #20389 ),
 .UNSPECIFIED., .F., .F. ) 
 B_SPLINE_CURVE_WITH_KNOTS ( ( 3, 2, 2, 2, 3 ),
 ( 0.5083333333333337478, 0.5125000000000003997, 0.5166666666666671626, 0.5208333333333338144, 0.5250000000000004663 ),
 .UNSPECIFIED. ) 
 CURVE ( )  GEOMETRIC_REPRESENTATION_ITEM ( )  RATIONAL_B_SPLINE_CURVE ( ( 0.9999999999999918954, 0.9238795325112948431, 1.000000000000000000, 0.9238795325112867385, 1.000000000000000000, 0.9238795325112867385, 1.000000000000000000, 0.9238795325112786339, 1.000000000000008216 ) ) 
 REPRESENTATION_ITEM ( '' )  );
#36688=CARTESIAN_POINT ( 'NONE',  ( -55.00000000000002132, -155.0000000000000284, 1.734723475976807094E-15 ) ) ;
#36716=CARTESIAN_POINT ( 'NONE',  ( -55.35523342533222291, -136.5625000013656063, 4.444560631937231499 ) ) ;
#36731=CARTESIAN_POINT ( 'NONE',  ( -59.81910112700026616, -147.3125000027311842, -2.462841084822525506 ) ) ;
#36735=VECTOR ( 'NONE', #18128, 1000.000000000000000 ) ;
#36759=CARTESIAN_POINT ( 'NONE',  ( -59.59170313451811296, -139.7500000013656347, 1.485763867205729394 ) ) ;
#36777=CARTESIAN_POINT ( 'NONE',  ( -58.39396692619412477, -135.6875000013656063, 2.891590998281057701 ) ) ;
#36783=AXIS2_PLACEMENT_3D ( 'NONE', #62224, #17528, #37453 ) ;
#36789=CARTESIAN_POINT ( 'NONE',  ( -52.10840900171896806, -147.4375000013656063, 3.393966926194110556 ) ) ;
#36801=CARTESIAN_POINT ( 'NONE',  ( -51.19402409849444524, -126.5000000000000284, -3.242614290531456334 ) ) ;
#36806=( BOUNDED_CURVE ( )  B_SPLINE_CURVE ( 2, ( #29306, #48622, #34145, #19036, #59237, #24824, #48936, #24506, #9699 ),
 .UNSPECIFIED., .F., .F. ) 
 B_SPLINE_CURVE_WITH_KNOTS ( ( 3, 2, 2, 2, 3 ),
 ( 0.6083333333333329485, 0.6124999999999997113, 0.6166666666666663632, 0.6208333333333330151, 0.6249999999999996669 ),
 .UNSPECIFIED. ) 
 CURVE ( )  GEOMETRIC_REPRESENTATION_ITEM ( )  RATIONAL_B_SPLINE_CURVE ( ( 1.000000000000005995, 0.9238795325112806323, 1.000000000000000000, 0.9238795325112867385, 1.000000000000000000, 0.9238795325112867385, 1.000000000000000000, 0.9238795325112928447, 0.9999999999999938938 ) ) 
 REPRESENTATION_ITEM ( '' )  );
#36810=CARTESIAN_POINT ( 'NONE',  ( -51.60603307380591787, -150.9375000013656063, -2.891590998281053704 ) ) ;
#36811=CARTESIAN_POINT ( 'NONE',  ( -58.80597590150559739, -150.1250000027312126, 3.242614290531460330 ) ) ;
#36835=CARTESIAN_POINT ( 'NONE',  ( -52.80376928212989185, -152.1250000013656063, -4.297418129356379346 ) ) ;
#36872=CARTESIAN_POINT ( 'NONE',  ( -55.39835681537999790, -136.8750000000000284, 4.984105922594378235 ) ) ;
#36882=CARTESIAN_POINT ( 'NONE',  ( -50.55543936806279248, -143.3125000013656063, 0.3552334253322060320 ) ) ;
#36884=CARTESIAN_POINT ( 'NONE',  ( -59.81910112700025905, -131.3125000027312694, -2.462841084822630311 ) ) ;
#36909=CARTESIAN_POINT ( 'NONE',  ( -50.70258187064364108, -132.1250000013656347, 2.196230717870141014 ) ) ;
#36921=CARTESIAN_POINT ( 'NONE',  ( -57.89159099828107458, -129.9375000013656063, -3.393966926194107447 ) ) ;
#36935=VERTEX_POINT ( 'NONE', #46853 ) ;
#36937=CARTESIAN_POINT ( 'NONE',  ( -59.81910112700027327, -139.3125000027312126, -2.462841084822392279 ) ) ;
#36947=ORIENTED_EDGE ( 'NONE', *, *, #1296, .T. ) ;
#36949=CARTESIAN_POINT ( 'NONE',  ( -58.39396692619412477, -139.4375000013656063, 2.891590998281057701 ) ) ;
#36954=CARTESIAN_POINT ( 'NONE',  ( -49.85088928181150436, -148.5625000000000000, -1.666127454062680702 ) ) ;
#36963=CARTESIAN_POINT ( 'NONE',  ( -58.80597590150559739, -143.1250000027312126, 3.242614290531460330 ) ) ;
#36975=CARTESIAN_POINT ( 'NONE',  ( -56.48576386720575471, -137.7500000013656063, -4.591703134518078322 ) ) ;
#36991=CARTESIAN_POINT ( 'NONE',  ( -56.48576386720575471, -146.7500000013655495, -4.591703134518078322 ) ) ;
#37017=AXIS2_PLACEMENT_3D ( 'NONE', #769, #54472, #15554 ) ;
#37034=CARTESIAN_POINT ( 'NONE',  ( -52.10840900171896806, -130.4375000013656063, 3.393966926194110556 ) ) ;
#37079=EDGE_CURVE ( 'NONE', #58923, #36394, #24931, .T. ) ;
#37084=CARTESIAN_POINT ( 'NONE',  ( -53.51423613279429503, -139.5000000013656063, 4.591703134518082763 ) ) ;
#37116=CARTESIAN_POINT ( 'NONE',  ( -53.51423613279429503, -144.5000000013656063, 4.591703134518082763 ) ) ;
#37134=CARTESIAN_POINT ( 'NONE',  ( -55.35523342533222291, -147.3125000013656063, 4.444560631937231499 ) ) ;
#37135=CARTESIAN_POINT ( 'NONE',  ( -60.14911071818854538, -150.1875000027312126, 1.666127454062681146 ) ) ;
#37158=CARTESIAN_POINT ( 'NONE',  ( -59.29741812935640155, -152.8750000013656063, -2.196230717870135685 ) ) ;
#37194=CARTESIAN_POINT ( 'NONE',  ( -50.01589407740564042, -135.6250000000000284, 0.3983568153799778022 ) ) ;
#37203=CARTESIAN_POINT ( 'NONE',  ( -59.29741812935640155, -138.8750000013656063, -2.196230717870135685 ) ) ;
#37205=CARTESIAN_POINT ( 'NONE',  ( -54.60164318462004474, -131.5000000027312126, -4.984105922594373794 ) ) ;
#37210=CARTESIAN_POINT ( 'NONE',  ( -59.81910112700026616, -151.3125000027312410, -2.462841084822585014 ) ) ;
#37217=CARTESIAN_POINT ( 'NONE',  ( -59.59170313451811296, -126.5000000013656063, 1.485763867205729394 ) ) ;
#37228=CARTESIAN_POINT ( 'NONE',  ( -53.51423613279429503, -134.2500000013656063, 4.591703134518082763 ) ) ;
#37239=CARTESIAN_POINT ( 'NONE',  ( -54.64476657466781973, -126.0625000013655921, -4.444560631937228834 ) ) ;
#37263=CARTESIAN_POINT ( 'NONE',  ( -53.51423613279429503, -137.2500000013656063, 4.591703134518083651 ) ) ;
#37269=CARTESIAN_POINT ( 'NONE',  ( -55.39835681537999790, -149.8750000000000284, 4.984105922594378235 ) ) ;
#37278=CARTESIAN_POINT ( 'NONE',  ( -56.48576386720575471, -153.0000000013656063, -4.591703134518078322 ) ) ;
#37279=CARTESIAN_POINT ( 'NONE',  ( -49.85088928181150436, -141.6875000027312126, -1.666127454062680702 ) ) ;
#37286=CARTESIAN_POINT ( 'NONE',  ( -59.29741812935640155, -137.6250000013655779, -2.196230717870135685 ) ) ;
#37288=CYLINDRICAL_SURFACE ( 'NONE', #40455, 5.000000000000000000 ) ;
#37301=CARTESIAN_POINT ( 'NONE',  ( -59.59170313451811296, -145.5000000013656063, 1.485763867205729394 ) ) ;
#37326=LINE ( 'NONE', #56646, #46238 ) ;
#37332=CARTESIAN_POINT ( 'NONE',  ( -53.33387254593711901, -140.9375000027311842, 5.149110718188534719 ) ) ;
#37341=CARTESIAN_POINT ( 'NONE',  ( -55.35523342533222291, -130.5625000013656063, 4.444560631937231499 ) ) ;
#37346=EDGE_CURVE ( 'NONE', #13129, #25936, #5633, .T. ) ;
#37358=( BOUNDED_CURVE ( )  B_SPLINE_CURVE ( 2, ( #43205, #39322, #4297, #3679, #14253, #33876, #33565, #48976, #53495 ),
 .UNSPECIFIED., .F., .F. ) 
 B_SPLINE_CURVE_WITH_KNOTS ( ( 3, 2, 2, 2, 3 ),
 ( 0.3750000000000002776, 0.3791666666666669294, 0.3833333333333336368, 0.3875000000000003442, 0.3916666666666669960 ),
 .UNSPECIFIED. ) 
 CURVE ( )  GEOMETRIC_REPRESENTATION_ITEM ( )  RATIONAL_B_SPLINE_CURVE ( ( 0.9999999999999948930, 0.9238795325112918455, 1.000000000000000000, 0.9238795325112867385, 1.000000000000000000, 0.9238795325112867385, 1.000000000000000000, 0.9238795325112806323, 1.000000000000005995 ) ) 
 REPRESENTATION_ITEM ( '' )  );
#37361=CARTESIAN_POINT ( 'NONE',  ( -49.85088928181150436, -148.6875000027312126, -1.666127454062680480 ) ) ;
#37371=CARTESIAN_POINT ( 'NONE',  ( -58.24261429053147765, -138.2500000000000000, -3.805975901505573855 ) ) ;
#37373=CARTESIAN_POINT ( 'NONE',  ( -58.24261429053147765, -144.3750000027312126, -3.805975901505573855 ) ) ;
#37385=CARTESIAN_POINT ( 'NONE',  ( -50.70258187064364108, -136.3750000013656063, 2.196230717870141014 ) ) ;
#37409=EDGE_CURVE ( 'NONE', #39907, #40253, #933, .T. ) ;
#37410=CARTESIAN_POINT ( 'NONE',  ( -58.24261429053147765, -151.2500000000000284, -3.805975901505573855 ) ) ;
#37420=CARTESIAN_POINT ( 'NONE',  ( -52.80376928212989185, -145.1250000013655779, -4.297418129356379346 ) ) ;
#37432=EDGE_CURVE ( 'NONE', #54748, #11960, #42038, .T. ) ;
#37441=CARTESIAN_POINT ( 'NONE',  ( -50.70258187064364108, -150.1250000013656063, 2.196230717870141014 ) ) ;
#37453=DIRECTION ( 'NONE',  ( -0.6485228581062915110, 0.000000000000000000, -0.7611951803011149931 ) ) ;
#37465=CARTESIAN_POINT ( 'NONE',  ( -50.55543936806279248, -149.3125000013656063, 0.3552334253322060320 ) ) ;
#37498=EDGE_CURVE ( 'NONE', #6296, #49700, #7492, .T. ) ;
#37500=CARTESIAN_POINT ( 'NONE',  ( -58.24261429053147765, -137.2500000000000000, -3.805975901505573855 ) ) ;
#37509=CARTESIAN_POINT ( 'NONE',  ( -50.40829686548195099, -139.2500000013656063, -1.485763867205728284 ) ) ;
#37511=CARTESIAN_POINT ( 'NONE',  ( -49.85088928181150436, -129.6875000027312126, -1.666127454062680702 ) ) ;
#37535=CARTESIAN_POINT ( 'NONE',  ( -50.40829686548195099, -132.0000000013656063, -1.485763867205728284 ) ) ;
#37545=CARTESIAN_POINT ( 'NONE',  ( -56.48576386720575471, -129.0000000013656063, -4.591703134518078322 ) ) ;
#37552=CARTESIAN_POINT ( 'NONE',  ( -58.80597590150559739, -135.0000000000000284, 3.242614290531460330 ) ) ;
#37572=CARTESIAN_POINT ( 'NONE',  ( -52.10840900171896806, -137.1875000013656063, 3.393966926194110556 ) ) ;
#37577=CARTESIAN_POINT ( 'NONE',  ( -56.66612745406270335, -148.3125000000000000, -5.149110718188516067 ) ) ;
#37585=CARTESIAN_POINT ( 'NONE',  ( -53.51423613279429503, -150.5000000013655779, 4.591703134518083651 ) ) ;
#37586=CARTESIAN_POINT ( 'NONE',  ( -58.80597590150559739, -141.1250000027312126, 3.242614290531460330 ) ) ;
#37593=CARTESIAN_POINT ( 'NONE',  ( -52.10840900171896806, -137.1875000013656063, 3.393966926194110556 ) ) ;
#37611=CARTESIAN_POINT ( 'NONE',  ( -59.29741812935640155, -146.6250000013656063, -2.196230717870135685 ) ) ;
#37631=ORIENTED_EDGE ( 'NONE', *, *, #49591, .F. ) ;
#37653=CARTESIAN_POINT ( 'NONE',  ( -58.39396692619412477, -132.6875000013656063, 2.891590998281057701 ) ) ;
#37662=CARTESIAN_POINT ( 'NONE',  ( -60.14911071818854538, -153.1875000027312410, 1.666127454062681368 ) ) ;
#37669=CARTESIAN_POINT ( 'NONE',  ( -57.46284108482265651, -147.0625000027312126, 4.819101127000238627 ) ) ;
#37693=CARTESIAN_POINT ( 'NONE',  ( -57.46284108482265651, -145.0625000027312126, 4.819101127000238627 ) ) ;
#37697=CARTESIAN_POINT ( 'NONE',  ( -56.48576386720575471, -135.0000000013656347, -4.591703134518078322 ) ) ;
#37699=ADVANCED_FACE ( 'NONE', ( #53405 ), #4514, .F. ) ;
#37732=CARTESIAN_POINT ( 'NONE',  ( -58.39396692619412477, -142.6875000013656063, 2.891590998281057701 ) ) ;
#37745=CARTESIAN_POINT ( 'NONE',  ( -56.66612745406270335, -125.3125000000000142, -5.149110718188516067 ) ) ;
#37748=AXIS2_PLACEMENT_3D ( 'NONE', #36688, #47596, #18329 ) ;
#37754=CARTESIAN_POINT ( 'NONE',  ( -56.48576386720575471, -146.7500000013655495, -4.591703134518078322 ) ) ;
#37771=CARTESIAN_POINT ( 'NONE',  ( -50.01589407740564042, -139.6250000000000284, 0.3983568153799778022 ) ) ;
#37782=CARTESIAN_POINT ( 'NONE',  ( -59.59170313451811296, -147.7500000013655779, 1.485763867205729394 ) ) ;
#37814=VERTEX_POINT ( 'NONE', #16080 ) ;
#37820=CARTESIAN_POINT ( 'NONE',  ( -57.46284108482265651, -137.9375000000000284, 4.819101127000239515 ) ) ;
#37826=ORIENTED_EDGE ( 'NONE', *, *, #25646, .T. ) ;
#37828=CARTESIAN_POINT ( 'NONE',  ( -56.48576386720575471, -140.0000000013656063, -4.591703134518078322 ) ) ;
#37830=CARTESIAN_POINT ( 'NONE',  ( -58.80597590150559739, -129.1250000027312126, 3.242614290531460330 ) ) ;
#37846=CARTESIAN_POINT ( 'NONE',  ( -51.60603307380591787, -124.9375000013656063, -2.891590998281053704 ) ) ;
#37857=CARTESIAN_POINT ( 'NONE',  ( -50.40829686548195099, -128.0000000013656063, -1.485763867205728284 ) ) ;
#37892=FACE_OUTER_BOUND ( 'NONE', #42326, .T. ) ;
#37901=CARTESIAN_POINT ( 'NONE',  ( -57.46284108482265651, -147.9375000000000000, 4.819101127000239515 ) ) ;
#37909=CARTESIAN_POINT ( 'NONE',  ( -59.44456063193725015, -148.8125000013656063, -0.3552334253322034230 ) ) ;
#37910=CARTESIAN_POINT ( 'NONE',  ( -50.18089887299979068, -143.8125000027312126, 2.462841084822635640 ) ) ;
#37918=CARTESIAN_POINT ( 'NONE',  ( -50.70258187064364108, -135.1250000013656063, 2.196230717870141014 ) ) ;
#37934=CARTESIAN_POINT ( 'NONE',  ( -54.64476657466781973, -140.8125000013656063, -4.444560631937228834 ) ) ;
#37960=DIRECTION ( 'NONE',  ( 0.000000000000000000, 1.000000000000000000, 0.000000000000000000 ) ) ;
#37968=CARTESIAN_POINT ( 'NONE',  ( -51.60603307380591787, -151.9375000013656063, -2.891590998281053704 ) ) ;
#37973=CARTESIAN_POINT ( 'NONE',  ( -52.53715891517739323, -149.5625000027312126, -4.819101127000233298 ) ) ;
#37977=CARTESIAN_POINT ( 'NONE',  ( -55.35523342533222291, -132.5625000013656063, 4.444560631937231499 ) ) ;
#37984=CARTESIAN_POINT ( 'NONE',  ( -49.85088928181150436, -152.6875000027311842, -1.666127454062680702 ) ) ;
#37991=DIRECTION ( 'NONE',  ( 0.000000000000000000, 1.000000000000000000, 0.000000000000000000 ) ) ;
#38016=VECTOR ( 'NONE', #19348, 1000.000000000000227 ) ;
#38019=CARTESIAN_POINT ( 'NONE',  ( -52.10840900171896806, -134.4375000013656063, 3.393966926194110556 ) ) ;
#38020=FACE_OUTER_BOUND ( 'NONE', #27418, .T. ) ;
#38049=CARTESIAN_POINT ( 'NONE',  ( -57.19623071787017210, -141.6250000013656063, 4.297418129356382899 ) ) ;
#38058=ORIENTED_EDGE ( 'NONE', *, *, #35111, .F. ) ;
#38070=CARTESIAN_POINT ( 'NONE',  ( -59.29741812935640155, -146.6250000013656063, -2.196230717870135685 ) ) ;
#38078=ADVANCED_FACE ( 'NONE', ( #61746 ), #37288, .F. ) ;
#38097=CARTESIAN_POINT ( 'NONE',  ( -55.35523342533222291, -147.5625000013656063, 4.444560631937231499 ) ) ;
#38123=CARTESIAN_POINT ( 'NONE',  ( -51.75738570946856498, -135.7500000000000284, 3.805975901505576964 ) ) ;
#38128=ORIENTED_EDGE ( 'NONE', *, *, #23718, .T. ) ;
#38135=DIRECTION ( 'NONE',  ( 0.000000000000000000, 1.000000000000000000, 0.000000000000000000 ) ) ;
#38136=CARTESIAN_POINT ( 'NONE',  ( -59.81910112700025905, -134.1875000000000284, -2.462841084822630311 ) ) ;
#38138=ORIENTED_EDGE ( 'NONE', *, *, #23832, .F. ) ;
#38144=CARTESIAN_POINT ( 'NONE',  ( -50.70258187064364108, -138.3750000013656063, 2.196230717870141014 ) ) ;
#38146=CARTESIAN_POINT ( 'NONE',  ( -49.85088928181150436, -125.6875000027311984, -1.666127454062680702 ) ) ;
#38152=VECTOR ( 'NONE', #8564, 1000.000000000000000 ) ;
#38155=DIRECTION ( 'NONE',  ( 0.000000000000000000, 1.000000000000000000, 0.000000000000000000 ) ) ;
#38173=CARTESIAN_POINT ( 'NONE',  ( -57.89159099828107458, -129.6875000013656063, -3.393966926194107447 ) ) ;
#38181=ORIENTED_EDGE ( 'NONE', *, *, #40150, .F. ) ;
#38184=CARTESIAN_POINT ( 'NONE',  ( -59.59170313451811296, -124.7500000013655921, 1.485763867205729394 ) ) ;
#38205=CARTESIAN_POINT ( 'NONE',  ( -50.55543936806279248, -150.3125000013656063, 0.3552334253322060320 ) ) ;
#38210=CARTESIAN_POINT ( 'NONE',  ( -51.60603307380591787, -135.9375000013656063, -2.891590998281053704 ) ) ;
#38217=CARTESIAN_POINT ( 'NONE',  ( -50.18089887299979068, -143.6875000000000284, 2.462841084822635640 ) ) ;
#38220=EDGE_CURVE ( 'NONE', #57381, #39445, #18190, .T. ) ;
#38228=CARTESIAN_POINT ( 'NONE',  ( -58.39396692619412477, -148.6875000013656063, 2.891590998281057701 ) ) ;
#38229=CARTESIAN_POINT ( 'NONE',  ( -60.14911071818854538, -139.1875000027312126, 1.666127454062681368 ) ) ;
#38237=CARTESIAN_POINT ( 'NONE',  ( -50.01589407740564042, -139.7500000027312126, 0.3983568153799778022 ) ) ;
#38238=CARTESIAN_POINT ( 'NONE',  ( -54.64476657466781973, -136.8125000013656063, -4.444560631937228834 ) ) ;
#38244=EDGE_LOOP ( 'NONE', ( #41194, #7228, #16293, #28861 ) ) ;
#38251=CARTESIAN_POINT ( 'NONE',  ( -53.51423613279429503, -142.2500000013656063, 4.591703134518082763 ) ) ;
#38280=VERTEX_POINT ( 'NONE', #40122 ) ;
#38288=CARTESIAN_POINT ( 'NONE',  ( -57.19623071787017210, -129.6250000013655779, 4.297418129356382899 ) ) ;
#38301=VERTEX_POINT ( 'NONE', #10534 ) ;
#38305=CARTESIAN_POINT ( 'NONE',  ( -50.01589407740564042, -150.7500000027312410, 0.3983568153799778022 ) ) ;
#38313=CARTESIAN_POINT ( 'NONE',  ( -51.75738570946856498, -153.8750000027312126, 3.805975901505576964 ) ) ;
#38317=CARTESIAN_POINT ( 'NONE',  ( -50.40829686548195099, -152.0000000013655779, -1.485763867205728284 ) ) ;
#38330=CARTESIAN_POINT ( 'NONE',  ( -57.19623071787017210, -134.6250000013656347, 4.297418129356382899 ) ) ;
#38359=CARTESIAN_POINT ( 'NONE',  ( -53.51423613279429503, -141.5000000013656063, 4.591703134518082763 ) ) ;
#38367=DIRECTION ( 'NONE',  ( 0.000000000000000000, 0.000000000000000000, 1.000000000000000000 ) ) ;
#38375=CARTESIAN_POINT ( 'NONE',  ( -50.55543936806279248, -145.0625000013656063, 0.3552334253322060320 ) ) ;
#38378=( BOUNDED_CURVE ( )  B_SPLINE_CURVE ( 2, ( #27465, #61261, #2106, #37135, #36811, #1782, #26522, #55798, #57073 ),
 .UNSPECIFIED., .F., .T. ) 
 B_SPLINE_CURVE_WITH_KNOTS ( ( 3, 2, 2, 2, 3 ),
 ( 0.1250000000000001110, 0.1291666666666667906, 0.1333333333333334425, 0.1375000000000001221, 0.1416666666666667740 ),
 .UNSPECIFIED. ) 
 CURVE ( )  GEOMETRIC_REPRESENTATION_ITEM ( )  RATIONAL_B_SPLINE_CURVE ( ( 0.9999999999999980016, 0.9238795325112887369, 1.000000000000000000, 0.9238795325112867385, 1.000000000000000000, 0.9238795325112867385, 1.000000000000000000, 0.9238795325112847401, 1.000000000000001998 ) ) 
 REPRESENTATION_ITEM ( '' )  );
#38386=CARTESIAN_POINT ( 'NONE',  ( -57.46284108482265651, -141.9375000000000284, 4.819101127000238627 ) ) ;
#38394=CARTESIAN_POINT ( 'NONE',  ( -58.80597590150559739, -144.0000000000000284, 3.242614290531460330 ) ) ;
#38401=CARTESIAN_POINT ( 'NONE',  ( -50.40829686548195099, -148.2500000013656063, -1.485763867205728284 ) ) ;
#38406=CARTESIAN_POINT ( 'NONE',  ( -60.14911071818854538, -136.1875000027312126, 1.666127454062681146 ) ) ;
#38433=CARTESIAN_POINT ( 'NONE',  ( -59.81910112700025905, -132.1875000000000568, -2.462841084822630311 ) ) ;
#38442=CARTESIAN_POINT ( 'NONE',  ( -59.81910112700025905, -127.3125000027312552, -2.462841084822630311 ) ) ;
#38444=CARTESIAN_POINT ( 'NONE',  ( -50.95487605259684472, -135.0000000000000853, 2.386008429272880704 ) ) ;
#38450=DIRECTION ( 'NONE',  ( 0.5000000000000001110, 0.000000000000000000, -0.8660254037844387076 ) ) ;
#38467=CARTESIAN_POINT ( 'NONE',  ( -50.70258187064364108, -130.1250000013656347, 2.196230717870141014 ) ) ;
#38469=CARTESIAN_POINT ( 'NONE',  ( -56.48576386720575471, -145.7500000013656063, -4.591703134518078322 ) ) ;
#38486=CARTESIAN_POINT ( 'NONE',  ( -56.66612745406293783, -137.4375000027312126, -5.149110718188535607 ) ) ;
#38500=CARTESIAN_POINT ( 'NONE',  ( -53.51423613279429503, -150.5000000013655779, 4.591703134518082763 ) ) ;
#38509=CARTESIAN_POINT ( 'NONE',  ( -54.60164318462004474, -146.3750000000000284, -4.984105922594373794 ) ) ;
#38518=CARTESIAN_POINT ( 'NONE',  ( -57.19623071787016499, -150.6250000013656063, 4.297418129356382899 ) ) ;
#38519=CARTESIAN_POINT ( 'NONE',  ( -49.85088928181150436, -136.6875000027312126, -1.666127454062680702 ) ) ;
#38527=CARTESIAN_POINT ( 'NONE',  ( -52.53715891517739323, -153.4375000000000284, -4.819101127000233298 ) ) ;
#38528=CARTESIAN_POINT ( 'NONE',  ( -50.55543936806279248, -133.0625000013656063, 0.3552334253322060320 ) ) ;
#38542=CARTESIAN_POINT ( 'NONE',  ( -56.48576386720575471, -140.7500000013655779, -4.591703134518078322 ) ) ;
#38544=EDGE_CURVE ( 'NONE', #31572, #14198, #4641, .T. ) ;
#38556=CARTESIAN_POINT ( 'NONE',  ( -55.39835681537999790, -148.8750000000000284, 4.984105922594378235 ) ) ;
#38584=CARTESIAN_POINT ( 'NONE',  ( -59.59170313451811296, -127.7500000013655921, 1.485763867205729394 ) ) ;
#38593=CARTESIAN_POINT ( 'NONE',  ( -58.24261429053147765, -149.3750000027312126, -3.805975901505573855 ) ) ;
#38608=CARTESIAN_POINT ( 'NONE',  ( -62.00000000000001421, -135.0000000000000284, 4.041451884327384114 ) ) ;
#38612=CARTESIAN_POINT ( 'NONE',  ( -52.80376928212989185, -153.8750000013655779, -4.297418129356379346 ) ) ;
#38613=EDGE_CURVE ( 'NONE', #26042, #46511, #61031, .T. ) ;
#38628=CARTESIAN_POINT ( 'NONE',  ( -59.44456063193725015, -136.8125000013656063, -0.3552334253322034230 ) ) ;
#38634=CARTESIAN_POINT ( 'NONE',  ( -55.39835681537999790, -139.8750000000000284, 4.984105922594378235 ) ) ;
#38637=ORIENTED_EDGE ( 'NONE', *, *, #27086, .F. ) ;
#38646=( BOUNDED_CURVE ( )  B_SPLINE_CURVE ( 2, ( #44767, #10678, #3418, #54436, #24526, #728, #94, #54754, #29973 ),
 .UNSPECIFIED., .F., .F. ) 
 B_SPLINE_CURVE_WITH_KNOTS ( ( 3, 2, 2, 2, 3 ),
 ( 0.4750000000000004219, 0.4791666666666671293, 0.4833333333333337811, 0.4875000000000004330, 0.4916666666666670849 ),
 .UNSPECIFIED. ) 
 CURVE ( )  GEOMETRIC_REPRESENTATION_ITEM ( )  RATIONAL_B_SPLINE_CURVE ( ( 0.9999999999999918954, 0.9238795325112948431, 1.000000000000000000, 0.9238795325112867385, 1.000000000000000000, 0.9238795325112867385, 1.000000000000000000, 0.9238795325112786339, 1.000000000000008216 ) ) 
 REPRESENTATION_ITEM ( '' )  );
#38651=CARTESIAN_POINT ( 'NONE',  ( -51.75738570946856498, -143.8750000027312126, 3.805975901505576964 ) ) ;
#38661=CARTESIAN_POINT ( 'NONE',  ( -57.19623071787017210, -139.6250000013655779, 4.297418129356382899 ) ) ;
#38672=CARTESIAN_POINT ( 'NONE',  ( -58.80597590150559739, -143.1250000027312126, 3.242614290531460330 ) ) ;
#38678=CARTESIAN_POINT ( 'NONE',  ( -52.80376928212989185, -146.8750000013656063, -4.297418129356379346 ) ) ;
#38688=AXIS2_PLACEMENT_3D ( 'NONE', #59856, #30237, #5808 ) ;
#38693=( BOUNDED_CURVE ( )  B_SPLINE_CURVE ( 2, ( #44366, #39858, #15111, #34727, #44686, #60466, #40193, #54355, #25399 ),
 .UNSPECIFIED., .F., .F. ) 
 B_SPLINE_CURVE_WITH_KNOTS ( ( 3, 2, 2, 2, 3 ),
 ( 0.1583333333333334925, 0.1625000000000001721, 0.1666666666666668239, 0.1708333333333335036, 0.1750000000000001554 ),
 .UNSPECIFIED. ) 
 CURVE ( )  GEOMETRIC_REPRESENTATION_ITEM ( )  RATIONAL_B_SPLINE_CURVE ( ( 0.9999999999999970024, 0.9238795325112897361, 1.000000000000000000, 0.9238795325112867385, 1.000000000000000000, 0.9238795325112867385, 1.000000000000000000, 0.9238795325112837409, 1.000000000000003109 ) ) 
 REPRESENTATION_ITEM ( '' )  );
#38704=CARTESIAN_POINT ( 'NONE',  ( -53.51423613279429503, -147.5000000013656063, 4.591703134518082763 ) ) ;
#38708=CARTESIAN_POINT ( 'NONE',  ( -57.46284108482265651, -136.0625000027312126, 4.819101127000238627 ) ) ;
#38712=ORIENTED_EDGE ( 'NONE', *, *, #28051, .F. ) ;
#38714=CARTESIAN_POINT ( 'NONE',  ( -57.46284108482265651, -140.9375000000000000, 4.819101127000238627 ) ) ;
#38742=CARTESIAN_POINT ( 'NONE',  ( -49.85088928181150436, -133.5625000000000284, -1.666127454062680702 ) ) ;
#38752=CARTESIAN_POINT ( 'NONE',  ( -54.60164318462004474, -126.5000000027312126, -4.984105922594373794 ) ) ;
#38777=CARTESIAN_POINT ( 'NONE',  ( -50.70258187064364108, -129.1250000013655779, 2.196230717870141014 ) ) ;
#38778=CARTESIAN_POINT ( 'NONE',  ( -50.70258187064364108, -145.1250000013656063, 2.196230717870141014 ) ) ;
#38802=CARTESIAN_POINT ( 'NONE',  ( -56.66612745406286678, -144.4375000027312126, -5.149110718188528502 ) ) ;
#38809=CARTESIAN_POINT ( 'NONE',  ( -59.44456063193725015, -151.8125000013656063, -0.3552334253322034230 ) ) ;
#38820=CARTESIAN_POINT ( 'NONE',  ( -51.19402409849444524, -145.5000000000000284, -3.242614290531456334 ) ) ;
#38831=CARTESIAN_POINT ( 'NONE',  ( -57.89159099828107458, -150.9375000013656063, -3.393966926194107447 ) ) ;
#38832=CARTESIAN_POINT ( 'NONE',  ( -58.24261429053147765, -138.3750000027312126, -3.805975901505573855 ) ) ;
#38839=( BOUNDED_CURVE ( )  B_SPLINE_CURVE ( 2, ( #51734, #36937, #22783, #55924, #56879, #56563, #7987, #1907, #11839 ),
 .UNSPECIFIED., .F., .F. ) 
 B_SPLINE_CURVE_WITH_KNOTS ( ( 3, 2, 2, 2, 3 ),
 ( 0.4916666666666670849, 0.4958333333333337922, 0.5000000000000004441, 0.5041666666666670960, 0.5083333333333337478 ),
 .UNSPECIFIED. ) 
 CURVE ( )  GEOMETRIC_REPRESENTATION_ITEM ( )  RATIONAL_B_SPLINE_CURVE ( ( 0.9999999999999918954, 0.9238795325112948431, 1.000000000000000000, 0.9238795325112867385, 1.000000000000000000, 0.9238795325112867385, 1.000000000000000000, 0.9238795325112786339, 1.000000000000008216 ) ) 
 REPRESENTATION_ITEM ( '' )  );
#38845=CARTESIAN_POINT ( 'NONE',  ( -50.55543936806279248, -134.0625000013656063, 0.3552334253322060320 ) ) ;
#38860=CARTESIAN_POINT ( 'NONE',  ( -59.44456063193725015, -142.5625000013656063, -0.3552334253322034230 ) ) ;
#38872=CARTESIAN_POINT ( 'NONE',  ( -58.24261429053147765, -139.2500000000000000, -3.805975901505573855 ) ) ;
#38901=CARTESIAN_POINT ( 'NONE',  ( -50.40829686548195099, -126.2500000013656063, -1.485763867205728284 ) ) ;
#38910=CARTESIAN_POINT ( 'NONE',  ( -58.80597590150559739, -143.0000000000000284, 3.242614290531460330 ) ) ;
#38914=CARTESIAN_POINT ( 'NONE',  ( -50.18089887299979068, -149.8125000027312126, 2.462841084822635640 ) ) ;
#38932=CARTESIAN_POINT ( 'NONE',  ( -51.60603307380591787, -153.9375000013656063, -2.891590998281053704 ) ) ;
#38962=LINE ( 'NONE', #28684, #38016 ) ;
#38976=CARTESIAN_POINT ( 'NONE',  ( -57.89159099828107458, -137.9375000013656063, -3.393966926194107447 ) ) ;
#39000=CARTESIAN_POINT ( 'NONE',  ( -54.64476657466781973, -145.8125000013656063, -4.444560631937228834 ) ) ;
#39005=EDGE_CURVE ( 'NONE', #11960, #32525, #21946, .T. ) ;
#39016=CYLINDRICAL_SURFACE ( 'NONE', #21316, 5.000000000000000000 ) ;
#39020=CARTESIAN_POINT ( 'NONE',  ( -57.46284108482265651, -140.0625000027312126, 4.819101127000238627 ) ) ;
#39026=CARTESIAN_POINT ( 'NONE',  ( -57.19623071787017210, -144.6250000013656063, 4.297418129356382899 ) ) ;
#39044=CARTESIAN_POINT ( 'NONE',  ( -58.24261429053147765, -145.3750000027312126, -3.805975901505573855 ) ) ;
#39063=CARTESIAN_POINT ( 'NONE',  ( -50.18089887299979068, -132.6875000000000284, 2.462841084822635640 ) ) ;
#39073=CARTESIAN_POINT ( 'NONE',  ( -51.19402409849444524, -126.6250000027312126, -3.242614290531456334 ) ) ;
#39096=CARTESIAN_POINT ( 'NONE',  ( -53.51423613279429503, -129.2500000013656347, 4.591703134518082763 ) ) ;
#39097=CARTESIAN_POINT ( 'NONE',  ( -52.80376928212989185, -146.8750000013656063, -4.297418129356378458 ) ) ;
#39131=CARTESIAN_POINT ( 'NONE',  ( -57.89159099828107458, -152.9375000013656063, -3.393966926194107447 ) ) ;
#39136=CARTESIAN_POINT ( 'NONE',  ( -56.48576386720575471, -136.7500000013655779, -4.591703134518078322 ) ) ;
#39142=CARTESIAN_POINT ( 'NONE',  ( -56.66612745406270335, -147.3125000000000284, -5.149110718188516067 ) ) ;
#39144=EDGE_LOOP ( 'NONE', ( #29696, #7034, #32274, #30273 ) ) ;
#39149=CARTESIAN_POINT ( 'NONE',  ( -53.51423613279429503, -145.5000000013656063, 4.591703134518083651 ) ) ;
#39151=CARTESIAN_POINT ( 'NONE',  ( -60.14911071818854538, -138.1875000027312126, 1.666127454062681368 ) ) ;
#39162=CARTESIAN_POINT ( 'NONE',  ( -54.60164318462004474, -139.5000000027312126, -4.984105922594373794 ) ) ;
#39163=CARTESIAN_POINT ( 'NONE',  ( -53.51423613279429503, -134.2500000013656063, 4.591703134518082763 ) ) ;
#39177=CARTESIAN_POINT ( 'NONE',  ( -59.59170313451811296, -140.5000000013656347, 1.485763867205729394 ) ) ;
#39211=CARTESIAN_POINT ( 'NONE',  ( -58.39396692619412477, -154.4375000013656063, 2.891590998281057701 ) ) ;
#39218=CARTESIAN_POINT ( 'NONE',  ( -59.44456063193725015, -127.8125000013655921, -0.3552334253322034230 ) ) ;
#39225=CARTESIAN_POINT ( 'NONE',  ( -55.39835681537999790, -142.8750000000000284, 4.984105922594378235 ) ) ;
#39229=CARTESIAN_POINT ( 'NONE',  ( -53.33387254593733928, -149.9375000027312126, 5.149110718188519620 ) ) ;
#39246=CARTESIAN_POINT ( 'NONE',  ( -55.35523342533222291, -154.3125000013656347, 4.444560631937231499 ) ) ;
#39265=DIRECTION ( 'NONE',  ( 0.000000000000000000, 1.000000000000000000, 0.000000000000000000 ) ) ;
#39293=CARTESIAN_POINT ( 'NONE',  ( -59.59170313451811296, -137.7500000013656063, 1.485763867205729394 ) ) ;
#39304=CARTESIAN_POINT ( 'NONE',  ( -53.33387254593719717, -142.9375000027312410, 5.149110718188530278 ) ) ;
#39312=CARTESIAN_POINT ( 'NONE',  ( -52.10840900171896806, -142.1875000013656063, 3.393966926194110556 ) ) ;
#39314=ORIENTED_EDGE ( 'NONE', *, *, #10669, .F. ) ;
#39322=CARTESIAN_POINT ( 'NONE',  ( -50.18089887299977647, -142.8125000027311557, 2.462841084822486426 ) ) ;
#39335=CARTESIAN_POINT ( 'NONE',  ( -54.64476657466781973, -142.0625000013656063, -4.444560631937228834 ) ) ;
#39375=ORIENTED_EDGE ( 'NONE', *, *, #53840, .F. ) ;
#39377=CARTESIAN_POINT ( 'NONE',  ( -58.80597590150559739, -133.0000000000000284, 3.242614290531460330 ) ) ;
#39386=CARTESIAN_POINT ( 'NONE',  ( -58.80597590150559739, -125.1250000027312126, 3.242614290531460330 ) ) ;
#39408=CARTESIAN_POINT ( 'NONE',  ( -58.39396692619412477, -154.6875000013656063, 2.891590998281057701 ) ) ;
#39409=CARTESIAN_POINT ( 'NONE',  ( -51.60603307380591787, -147.9375000013656063, -2.891590998281053704 ) ) ;
#39437=ORIENTED_EDGE ( 'NONE', *, *, #40150, .T. ) ;
#39445=VERTEX_POINT ( 'NONE', #61552 ) ;
#39446=CARTESIAN_POINT ( 'NONE',  ( -52.10840900171896806, -151.4375000013656063, 3.393966926194110556 ) ) ;
#39458=CARTESIAN_POINT ( 'NONE',  ( -59.98410592259440222, -144.1250000000000284, -0.3983568153799752487 ) ) ;
#39466=CARTESIAN_POINT ( 'NONE',  ( -50.55543936806279248, -147.3125000013656063, 0.3552334253322060320 ) ) ;
#39467=CARTESIAN_POINT ( 'NONE',  ( -58.80597590150559739, -139.1250000027312410, 3.242614290531460330 ) ) ;
#39480=CARTESIAN_POINT ( 'NONE',  ( -52.80376928212989185, -134.8750000013656063, -4.297418129356379346 ) ) ;
#39482=CARTESIAN_POINT ( 'NONE',  ( -57.46284108482265651, -146.0625000027312126, 4.819101127000238627 ) ) ;
#39495=CARTESIAN_POINT ( 'NONE',  ( -50.55543936806279248, -138.0625000013656063, 0.3552334253322060320 ) ) ;
#39526=CARTESIAN_POINT ( 'NONE',  ( -50.70258187064364108, -151.1250000013656347, 2.196230717870141014 ) ) ;
#39533=CARTESIAN_POINT ( 'NONE',  ( -55.35523342533222291, -128.5625000013656063, 4.444560631937231499 ) ) ;
#39543=CARTESIAN_POINT ( 'NONE',  ( -58.24261429053147765, -152.3750000027312126, -3.805975901505573855 ) ) ;
#39558=CARTESIAN_POINT ( 'NONE',  ( -57.46284108482265651, -154.0625000027312126, 4.819101127000238627 ) ) ;
#39563=CARTESIAN_POINT ( 'NONE',  ( -53.51423613279429503, -153.2500000013655779, 4.591703134518082763 ) ) ;
#39587=CARTESIAN_POINT ( 'NONE',  ( -59.24072208773964832, -135.0000000000000568, 2.598697453439798188 ) ) ;
#39609=CARTESIAN_POINT ( 'NONE',  ( -54.64476657466781973, -139.0625000013656063, -4.444560631937228834 ) ) ;
#39613=ORIENTED_EDGE ( 'NONE', *, *, #17664, .F. ) ;
#39627=CARTESIAN_POINT ( 'NONE',  ( -50.55543936806279248, -139.0625000013656063, 0.3552334253322060320 ) ) ;
#39653=CARTESIAN_POINT ( 'NONE',  ( -50.40829686548195099, -145.2500000013656347, -1.485763867205728284 ) ) ;
#39692=CARTESIAN_POINT ( 'NONE',  ( -58.80597590150559739, -131.0000000000000284, 3.242614290531460330 ) ) ;
#39700=ORIENTED_EDGE ( 'NONE', *, *, #56215, .T. ) ;
#39702=CARTESIAN_POINT ( 'NONE',  ( -54.64476657466781973, -153.8125000013656347, -4.444560631937228834 ) ) ;
#39727=CARTESIAN_POINT ( 'NONE',  ( -50.40829686548195099, -154.2500000013656063, -1.485763867205728284 ) ) ;
#39728=CARTESIAN_POINT ( 'NONE',  ( -57.19623071787016499, -147.3750000013656063, 4.297418129356382899 ) ) ;
#39757=CARTESIAN_POINT ( 'NONE',  ( -59.44456063193725015, -147.8125000013656063, -0.3552334253322034230 ) ) ;
#39767=CARTESIAN_POINT ( 'NONE',  ( -52.53715891517739323, -142.4375000000000000, -4.819101127000233298 ) ) ;
#39778=CARTESIAN_POINT ( 'NONE',  ( -57.19623071787016499, -144.6250000013656063, 4.297418129356382899 ) ) ;
#39780=CARTESIAN_POINT ( 'NONE',  ( -49.85088928181150436, -133.6875000027312126, -1.666127454062680702 ) ) ;
#39795=CARTESIAN_POINT ( 'NONE',  ( -54.64476657466781973, -133.8125000013656063, -4.444560631937228834 ) ) ;
#39812=CARTESIAN_POINT ( 'NONE',  ( -51.60603307380591787, -136.9375000013655779, -2.891590998281053704 ) ) ;
#39820=CARTESIAN_POINT ( 'NONE',  ( -59.44456063193725015, -131.8125000013656063, -0.3552334253322034230 ) ) ;
#39825=CARTESIAN_POINT ( 'NONE',  ( -57.46284108482265651, -153.0625000027312126, 4.819101127000238627 ) ) ;
#39845=CARTESIAN_POINT ( 'NONE',  ( -50.40829686548195099, -151.0000000013656063, -1.485763867205728284 ) ) ;
#39852=CARTESIAN_POINT ( 'NONE',  ( -51.60603307380591787, -128.1875000013656063, -2.891590998281053704 ) ) ;
#39858=CARTESIAN_POINT ( 'NONE',  ( -59.81910112700027327, -150.1875000000000000, -2.462841084822540605 ) ) ;
#39862=CARTESIAN_POINT ( 'NONE',  ( -58.24261429053147765, -146.3750000027312126, -3.805975901505573855 ) ) ;
#39881=CARTESIAN_POINT ( 'NONE',  ( -49.85088928181150436, -143.5625000000000568, -1.666127454062680480 ) ) ;
#39883=CARTESIAN_POINT ( 'NONE',  ( -57.19623071787017210, -151.3750000013656063, 4.297418129356382899 ) ) ;
#39907=VERTEX_POINT ( 'NONE', #28688 ) ;
#39929=AXIS2_PLACEMENT_3D ( 'NONE', #1058, #6186, #10361 ) ;
#39930=CARTESIAN_POINT ( 'NONE',  ( -53.51423613279429503, -139.5000000013656063, 4.591703134518082763 ) ) ;
#39937=CARTESIAN_POINT ( 'NONE',  ( -50.75781946612335105, -135.0000000000005969, -1.372666862511563224 ) ) ;
#39946=CARTESIAN_POINT ( 'NONE',  ( -56.48576386720575471, -142.7500000013656063, -4.591703134518078322 ) ) ;
#39976=CARTESIAN_POINT ( 'NONE',  ( -56.48576386720575471, -146.0000000013656347, -4.591703134518078322 ) ) ;
#40014=( GEOMETRIC_REPRESENTATION_CONTEXT ( 3 ) GLOBAL_UNCERTAINTY_ASSIGNED_CONTEXT ( ( #24272 ) ) GLOBAL_UNIT_ASSIGNED_CONTEXT ( ( #7698, #27301, #21852 ) ) REPRESENTATION_CONTEXT ( 'NONE', 'WORKASPACE' ) );
#40016=CARTESIAN_POINT ( 'NONE',  ( -50.01589407740564042, -129.6250000000000284, 0.3983568153799778022 ) ) ;
#40020=ORIENTED_EDGE ( 'NONE', *, *, #37079, .F. ) ;
#40024=CARTESIAN_POINT ( 'NONE',  ( -54.60164318462004474, -124.5000000027311984, -4.984105922594373794 ) ) ;
#40036=CARTESIAN_POINT ( 'NONE',  ( -60.14911071818854538, -145.0625000000000284, 1.666127454062681146 ) ) ;
#40050=CARTESIAN_POINT ( 'NONE',  ( -50.70258187064364108, -126.1250000013656205, 2.196230717870141014 ) ) ;
#40051=CARTESIAN_POINT ( 'NONE',  ( -56.48576386720575471, -141.7500000013656063, -4.591703134518078322 ) ) ;
#40094=CARTESIAN_POINT ( 'NONE',  ( -57.46284108482265651, -139.9375000000000284, 4.819101127000239515 ) ) ;
#40103=CARTESIAN_POINT ( 'NONE',  ( -57.19623071787016499, -145.6250000013655779, 4.297418129356382899 ) ) ;
#40106=CARTESIAN_POINT ( 'NONE',  ( -57.46284108482265651, -136.0625000027311842, 4.819101127000239515 ) ) ;
#40120=CARTESIAN_POINT ( 'NONE',  ( -57.89159099828107458, -127.6875000013656063, -3.393966926194107447 ) ) ;
#40122=CARTESIAN_POINT ( 'NONE',  ( -58.24261429053147765, -154.2500000000000284, -3.805975901505573855 ) ) ;
#40127=DIRECTION ( 'NONE',  ( 0.000000000000000000, 1.000000000000000000, 0.000000000000000000 ) ) ;
#40128=LINE ( 'NONE', #49781, #27769 ) ;
#40135=CARTESIAN_POINT ( 'NONE',  ( -51.60603307380591787, -137.9375000013656063, -2.891590998281053704 ) ) ;
#40144=CARTESIAN_POINT ( 'NONE',  ( -50.40829686548195099, -132.2500000013656063, -1.485763867205728284 ) ) ;
#40150=EDGE_CURVE ( 'NONE', #37814, #45194, #31554, .T. ) ;
#40178=CARTESIAN_POINT ( 'NONE',  ( -59.29741812935640155, -149.6250000013655779, -2.196230717870135685 ) ) ;
#40187=CARTESIAN_POINT ( 'NONE',  ( -54.60164318462004474, -152.3750000000000284, -4.984105922594373794 ) ) ;
#40193=CARTESIAN_POINT ( 'NONE',  ( -55.39835681537999790, -149.8750000000000284, 4.984105922594378235 ) ) ;
#40194=ORIENTED_EDGE ( 'NONE', *, *, #63242, .F. ) ;
#40195=DIRECTION ( 'NONE',  ( -0.6485228581062915110, 0.000000000000000000, -0.7611951803011149931 ) ) ;
#40197=CARTESIAN_POINT ( 'NONE',  ( -52.53715891517739323, -145.5625000027312126, -4.819101127000233298 ) ) ;
#40215=CARTESIAN_POINT ( 'NONE',  ( -54.64476657466781973, -147.8125000013656063, -4.444560631937228834 ) ) ;
#40226=( BOUNDED_CURVE ( )  B_SPLINE_CURVE ( 2, ( #28674, #23861, #43464, #19340, #53751, #9374, #38634, #33822, #53441 ),
 .UNSPECIFIED., .F., .F. ) 
 B_SPLINE_CURVE_WITH_KNOTS ( ( 3, 2, 2, 2, 3 ),
 ( 0.4916666666666670849, 0.4958333333333337922, 0.5000000000000004441, 0.5041666666666670960, 0.5083333333333337478 ),
 .UNSPECIFIED. ) 
 CURVE ( )  GEOMETRIC_REPRESENTATION_ITEM ( )  RATIONAL_B_SPLINE_CURVE ( ( 0.9999999999999918954, 0.9238795325112948431, 1.000000000000000000, 0.9238795325112867385, 1.000000000000000000, 0.9238795325112867385, 1.000000000000000000, 0.9238795325112786339, 1.000000000000008216 ) ) 
 REPRESENTATION_ITEM ( '' )  );
#40235=CARTESIAN_POINT ( 'NONE',  ( -52.53715891517739323, -151.5625000027312126, -4.819101127000233298 ) ) ;
#40240=CARTESIAN_POINT ( 'NONE',  ( -57.11050704595625405, -135.0000000000000000, -4.001714258895231247 ) ) ;
#40253=VERTEX_POINT ( 'NONE', #23491 ) ;
#40262=CARTESIAN_POINT ( 'NONE',  ( -59.59170313451811296, -134.7500000013656063, 1.485763867205729394 ) ) ;
#40264=EDGE_CURVE ( 'NONE', #62694, #54373, #52131, .T. ) ;
#40272=DIRECTION ( 'NONE',  ( 0.000000000000000000, 1.000000000000000000, 0.000000000000000000 ) ) ;
#40281=CARTESIAN_POINT ( 'NONE',  ( -52.10840900171896806, -140.1875000013656063, 3.393966926194110556 ) ) ;
#40306=CARTESIAN_POINT ( 'NONE',  ( -57.89159099828107458, -142.9375000013656063, -3.393966926194107447 ) ) ;
#40341=CARTESIAN_POINT ( 'NONE',  ( -58.24261429053147765, -129.2500000000000284, -3.805975901505573855 ) ) ;
#40349=CARTESIAN_POINT ( 'NONE',  ( -55.35523342533222291, -153.3125000013656063, 4.444560631937231499 ) ) ;
#40370=ORIENTED_EDGE ( 'NONE', *, *, #21609, .F. ) ;
#40375=CARTESIAN_POINT ( 'NONE',  ( -50.40829686548195099, -127.0000000013656063, -1.485763867205728284 ) ) ;
#40376=CARTESIAN_POINT ( 'NONE',  ( -59.59170313451810586, -144.5000000013656063, 1.485763867205729394 ) ) ;
#40403=VECTOR ( 'NONE', #49764, 1000.000000000000000 ) ;
#40413=CARTESIAN_POINT ( 'NONE',  ( -50.18089887299979068, -139.6875000000000284, 2.462841084822635640 ) ) ;
#40423=CARTESIAN_POINT ( 'NONE',  ( -55.35523342533222291, -145.5625000013656063, 4.444560631937231499 ) ) ;
#40425=CARTESIAN_POINT ( 'NONE',  ( -51.75738570946856498, -132.8750000027312126, 3.805975901505576964 ) ) ;
#40439=CARTESIAN_POINT ( 'NONE',  ( -56.48576386720575471, -128.7500000013656063, -4.591703134518078322 ) ) ;
#40455=AXIS2_PLACEMENT_3D ( 'NONE', #56917, #58481, #48505 ) ;
#40456=CARTESIAN_POINT ( 'NONE',  ( -58.39396692619412477, -137.4375000013656063, 2.891590998281057701 ) ) ;
#40466=CARTESIAN_POINT ( 'NONE',  ( -50.55543936806279248, -132.3125000013656063, 0.3552334253322060320 ) ) ;
#40485=ORIENTED_EDGE ( 'NONE', *, *, #22896, .T. ) ;
#40489=ORIENTED_EDGE ( 'NONE', *, *, #16118, .T. ) ;
#40490=CARTESIAN_POINT ( 'NONE',  ( -51.60603307380591787, -148.9375000013656063, -2.891590998281053704 ) ) ;
#40497=CARTESIAN_POINT ( 'NONE',  ( -58.80597590150559739, -154.0000000000000284, 3.242614290531460330 ) ) ;
#40500=VECTOR ( 'NONE', #46351, 1000.000000000000000 ) ;
#40508=CARTESIAN_POINT ( 'NONE',  ( -58.80597590150559739, -147.1250000027312126, 3.242614290531460330 ) ) ;
#40524=CARTESIAN_POINT ( 'NONE',  ( -51.19402409849444524, -143.5000000000000284, -3.242614290531456334 ) ) ;
#40525=EDGE_CURVE ( 'NONE', #40939, #26042, #54335, .T. ) ;
#40528=CARTESIAN_POINT ( 'NONE',  ( -52.80376928212989185, -148.8750000013655779, -4.297418129356379346 ) ) ;
#40574=CARTESIAN_POINT ( 'NONE',  ( -59.59170313451811296, -136.7500000013655779, 1.485763867205729394 ) ) ;
#40576=ORIENTED_EDGE ( 'NONE', *, *, #32988, .T. ) ;
#40592=CARTESIAN_POINT ( 'NONE',  ( -54.64476657466781973, -142.8125000013656063, -4.444560631937228834 ) ) ;
#40601=CARTESIAN_POINT ( 'NONE',  ( -51.19402409849444524, -147.5000000000000284, -3.242614290531456334 ) ) ;
#40620=CARTESIAN_POINT ( 'NONE',  ( -59.59170313451811296, -140.7500000013655779, 1.485763867205729394 ) ) ;
#40635=CARTESIAN_POINT ( 'NONE',  ( -56.66612745406293783, -138.4375000027312126, -5.149110718188535607 ) ) ;
#40654=CARTESIAN_POINT ( 'NONE',  ( -58.24261429053147765, -137.2500000000000000, -3.805975901505573855 ) ) ;
#40656=CARTESIAN_POINT ( 'NONE',  ( -51.19402409849444524, -141.5000000000000284, -3.242614290531456334 ) ) ;
#40661=CARTESIAN_POINT ( 'NONE',  ( -55.39835681537999790, -128.8750000000000284, 4.984105922594378235 ) ) ;
#40667=CARTESIAN_POINT ( 'NONE',  ( -59.44456063193725015, -152.5625000013656063, -0.3552334253322034230 ) ) ;
#40668=LINE ( 'NONE', #60312, #54161 ) ;
#40691=CARTESIAN_POINT ( 'NONE',  ( -52.80376928212989185, -124.8750000013656205, -4.297418129356379346 ) ) ;
#40692=CARTESIAN_POINT ( 'NONE',  ( -51.60603307380591787, -142.9375000013656063, -2.891590998281053704 ) ) ;
#40720=VECTOR ( 'NONE', #58706, 1000.000000000000000 ) ;
#40730=ORIENTED_EDGE ( 'NONE', *, *, #41605, .T. ) ;
#40731=CARTESIAN_POINT ( 'NONE',  ( -51.75738570946856498, -140.7500000000000000, 3.805975901505576964 ) ) ;
#40740=CARTESIAN_POINT ( 'NONE',  ( -57.19623071787016499, -142.6250000013656063, 4.297418129356382899 ) ) ;
#40742=CARTESIAN_POINT ( 'NONE',  ( -58.24261429053147765, -133.3750000027312126, -3.805975901505573855 ) ) ;
#40755=CARTESIAN_POINT ( 'NONE',  ( -52.80376928212989185, -127.8750000013656063, -4.297418129356379346 ) ) ;
#40771=CARTESIAN_POINT ( 'NONE',  ( -51.60603307380591787, -135.9375000013656063, -2.891590998281053704 ) ) ;
#40781=CARTESIAN_POINT ( 'NONE',  ( -58.39396692619412477, -131.6875000013656063, 2.891590998281057701 ) ) ;
#40794=CARTESIAN_POINT ( 'NONE',  ( -59.98410592259440222, -138.2500000027312126, -0.3983568153799752487 ) ) ;
#40808=LINE ( 'NONE', #36001, #63544 ) ;
#40811=CARTESIAN_POINT ( 'NONE',  ( -50.18089887299979068, -153.6875000000000284, 2.462841084822635640 ) ) ;
#40822=CARTESIAN_POINT ( 'NONE',  ( -55.35523342533222291, -153.5625000013656063, 4.444560631937231499 ) ) ;
#40824=CARTESIAN_POINT ( 'NONE',  ( -59.81910112700025905, -145.3125000027312126, -2.462841084822630311 ) ) ;
#40825=( BOUNDED_CURVE ( )  B_SPLINE_CURVE ( 2, ( #42831, #42516, #33504, #62783, #8437, #37693, #43142, #32874, #12619 ),
 .UNSPECIFIED., .F., .F. ) 
 B_SPLINE_CURVE_WITH_KNOTS ( ( 3, 2, 2, 2, 3 ),
 ( 0.2916666666666669072, 0.2958333333333335591, 0.3000000000000002665, 0.3041666666666669183, 0.3083333333333336257 ),
 .UNSPECIFIED. ) 
 CURVE ( )  GEOMETRIC_REPRESENTATION_ITEM ( )  RATIONAL_B_SPLINE_CURVE ( ( 0.9999999999999958922, 0.9238795325112908463, 1.000000000000000000, 0.9238795325112867385, 1.000000000000000000, 0.9238795325112867385, 1.000000000000000000, 0.9238795325112816315, 1.000000000000005107 ) ) 
 REPRESENTATION_ITEM ( '' )  );
#40843=CARTESIAN_POINT ( 'NONE',  ( -58.39396692619412477, -151.4375000013656063, 2.891590998281057701 ) ) ;
#40849=CYLINDRICAL_SURFACE ( 'NONE', #21272, 5.000000000000000000 ) ;
#40878=VERTEX_POINT ( 'NONE', #61714 ) ;
#40889=CARTESIAN_POINT ( 'NONE',  ( -50.55543936806279248, -133.3125000013656063, 0.3552334253322060320 ) ) ;
#40931=CARTESIAN_POINT ( 'NONE',  ( -59.29741812935640155, -141.8750000013655779, -2.196230717870135685 ) ) ;
#40939=VERTEX_POINT ( 'NONE', #2539 ) ;
#40952=ADVANCED_FACE ( 'NONE', ( #62344 ), #18265, .T. ) ;
#40953=CARTESIAN_POINT ( 'NONE',  ( -53.51423613279429503, -135.5000000013656063, 4.591703134518083651 ) ) ;
#40956=ADVANCED_FACE ( 'NONE', ( #37892 ), #17063, .F. ) ;
#40960=CARTESIAN_POINT ( 'NONE',  ( -59.98410592259440222, -151.1250000000000284, -0.3983568153799752487 ) ) ;
#40966=CARTESIAN_POINT ( 'NONE',  ( -56.48576386720575471, -148.0000000013655779, -4.591703134518078322 ) ) ;
#40973=CARTESIAN_POINT ( 'NONE',  ( -54.60164318462004474, -141.3750000000000284, -4.984105922594373794 ) ) ;
#40982=CARTESIAN_POINT ( 'NONE',  ( -49.85088928181150436, -129.5625000000000284, -1.666127454062680702 ) ) ;
#40988=CARTESIAN_POINT ( 'NONE',  ( -52.10840900171896806, -150.1875000013656063, 3.393966926194110556 ) ) ;
#40996=CARTESIAN_POINT ( 'NONE',  ( -49.85088928181150436, -152.6875000027312126, -1.666127454062680480 ) ) ;
#41012=CARTESIAN_POINT ( 'NONE',  ( -57.89159099828107458, -151.9375000013656063, -3.393966926194107447 ) ) ;
#41013=CARTESIAN_POINT ( 'NONE',  ( -52.10840900171896806, -144.1875000013656063, 3.393966926194110556 ) ) ;
#41016=CARTESIAN_POINT ( 'NONE',  ( -51.75738570946856498, -153.8750000027312126, 3.805975901505576964 ) ) ;
#41036=MECHANICAL_DESIGN_GEOMETRIC_PRESENTATION_REPRESENTATION('',(#28718),#40014);
#41049=CARTESIAN_POINT ( 'NONE',  ( -56.66612745406270335, -142.3125000000000000, -5.149110718188516067 ) ) ;
#41059=CARTESIAN_POINT ( 'NONE',  ( -54.64476657466781973, -142.0625000013656063, -4.444560631937228834 ) ) ;
#41061=CARTESIAN_POINT ( 'NONE',  ( -50.01589407740564042, -135.7500000027312126, 0.3983568153799778022 ) ) ;
#41072=CARTESIAN_POINT ( 'NONE',  ( -58.39396692619412477, -128.4375000013656063, 2.891590998281057701 ) ) ;
#41086=CARTESIAN_POINT ( 'NONE',  ( -52.10840900171896806, -135.1875000013656063, 3.393966926194110556 ) ) ;
#41093=( LENGTH_UNIT ( ) NAMED_UNIT ( * ) SI_UNIT ( .MILLI., .METRE. ) );
#41096=CARTESIAN_POINT ( 'NONE',  ( -58.39396692619412477, -132.6875000013656063, 2.891590998281057701 ) ) ;
#41099=VECTOR ( 'NONE', #9649, 1000.000000000000114 ) ;
#41102=DIRECTION ( 'NONE',  ( -0.6485228581062915110, 0.000000000000000000, -0.7611951803011149931 ) ) ;
#41106=CARTESIAN_POINT ( 'NONE',  ( -54.60164318462004474, -151.3750000000000284, -4.984105922594373794 ) ) ;
#41122=CARTESIAN_POINT ( 'NONE',  ( -52.10840900171896806, -140.1875000013656063, 3.393966926194110556 ) ) ;
#41129=CARTESIAN_POINT ( 'NONE',  ( -59.29741812935640155, -124.8750000013656205, -2.196230717870135685 ) ) ;
#41139=CARTESIAN_POINT ( 'NONE',  ( -60.14911071818854538, -148.1875000027312126, 1.666127454062681368 ) ) ;
#41158=CARTESIAN_POINT ( 'NONE',  ( -58.80597590150559739, -138.0000000000000284, 3.242614290531460330 ) ) ;
#41159=CARTESIAN_POINT ( 'NONE',  ( -52.10840900171896806, -151.1875000013656063, 3.393966926194110556 ) ) ;
#41171=VECTOR ( 'NONE', #43782, 1000.000000000000000 ) ;
#41194=ORIENTED_EDGE ( 'NONE', *, *, #20950, .F. ) ;
#41203=CARTESIAN_POINT ( 'NONE',  ( -56.48576386720575471, -135.0000000013656347, -4.591703134518078322 ) ) ;
#41215=CARTESIAN_POINT ( 'NONE',  ( -52.53715891517739323, -149.4375000000000000, -4.819101127000233298 ) ) ;
#41222=CARTESIAN_POINT ( 'NONE',  ( -55.00000000000002132, -155.0000000000000284, 1.734723475976807094E-15 ) ) ;
#41228=CARTESIAN_POINT ( 'NONE',  ( -56.66612745406283125, -147.3125000000000284, -5.149110718188525837 ) ) ;
#41244=CARTESIAN_POINT ( 'NONE',  ( -51.60603307380591787, -140.1875000013656063, -2.891590998281053704 ) ) ;
#41277=CARTESIAN_POINT ( 'NONE',  ( -57.19623071787017210, -145.6250000013655779, 4.297418129356382899 ) ) ;
#41290=CARTESIAN_POINT ( 'NONE',  ( -55.39835681537999790, -125.8750000000000142, 4.984105922594378235 ) ) ;
#41298=CARTESIAN_POINT ( 'NONE',  ( -59.29741812935640155, -150.6250000013656063, -2.196230717870135685 ) ) ;
#41301=VERTEX_POINT ( 'NONE', #13211 ) ;
#41320=ORIENTED_EDGE ( 'NONE', *, *, #17333, .T. ) ;
#41325=CARTESIAN_POINT ( 'NONE',  ( -55.35523342533222291, -151.5625000013656063, 4.444560631937231499 ) ) ;
#41364=CARTESIAN_POINT ( 'NONE',  ( -57.46284108482265651, -136.9375000000000000, 4.819101127000239515 ) ) ;
#41373=CARTESIAN_POINT ( 'NONE',  ( -59.44456063193725015, -142.8125000013656063, -0.3552334253322034230 ) ) ;
#41375=CARTESIAN_POINT ( 'NONE',  ( -56.66612745406270335, -131.4375000027312126, -5.149110718188516067 ) ) ;
#41389=CARTESIAN_POINT ( 'NONE',  ( -54.64476657466781973, -128.8125000013656063, -4.444560631937228834 ) ) ;
#41402=CARTESIAN_POINT ( 'NONE',  ( -59.44456063193725015, -132.5625000013656063, -0.3552334253322034230 ) ) ;
#41413=CARTESIAN_POINT ( 'NONE',  ( -57.89159099828107458, -127.9375000013656063, -3.393966926194107447 ) ) ;
#41435=CARTESIAN_POINT ( 'NONE',  ( -57.89159099828107458, -153.9375000013656063, -3.393966926194107447 ) ) ;
#41439=CARTESIAN_POINT ( 'NONE',  ( -59.59170313451810586, -139.5000000013656063, 1.485763867205729394 ) ) ;
#41444=CARTESIAN_POINT ( 'NONE',  ( -59.81910112700025905, -152.1875000000000284, -2.462841084822630311 ) ) ;
#41454=CARTESIAN_POINT ( 'NONE',  ( -51.19402409849444524, -141.6250000027312126, -3.242614290531456334 ) ) ;
#41475=CARTESIAN_POINT ( 'NONE',  ( -59.29741812935640155, -144.6250000013656063, -2.196230717870135685 ) ) ;
#41517=ADVANCED_FACE ( 'NONE', ( #20249 ), #25717, .F. ) ;
#41518=CARTESIAN_POINT ( 'NONE',  ( -50.70258187064364108, -134.3750000013656347, 2.196230717870141014 ) ) ;
#41525=ORIENTED_EDGE ( 'NONE', *, *, #389, .T. ) ;
#41526=LINE ( 'NONE', #61177, #8018 ) ;
#41559=CARTESIAN_POINT ( 'NONE',  ( -57.19623071787017210, -139.6250000013655779, 4.297418129356382899 ) ) ;
#41591=CARTESIAN_POINT ( 'NONE',  ( -51.60603307380591787, -146.1875000013656063, -2.891590998281053704 ) ) ;
#41598=DIRECTION ( 'NONE',  ( -0.000000000000000000, 0.000000000000000000, 1.000000000000000000 ) ) ;
#41605=EDGE_CURVE ( 'NONE', #36935, #52748, #515, .T. ) ;
#41610=CARTESIAN_POINT ( 'NONE',  ( -53.51423613279429503, -149.2500000013655779, 4.591703134518082763 ) ) ;
#41625=DIRECTION ( 'NONE',  ( 0.5000000000000003331, 0.000000000000000000, 0.8660254037844385966 ) ) ;
#41633=CARTESIAN_POINT ( 'NONE',  ( -50.70258187064364108, -153.3750000013656347, 2.196230717870141014 ) ) ;
#41648=CARTESIAN_POINT ( 'NONE',  ( -53.33387254593758087, -135.8125000000000284, 5.149110718188498304 ) ) ;
#41676=CARTESIAN_POINT ( 'NONE',  ( -51.75738570946856498, -138.7500000000000000, 3.805975901505576964 ) ) ;
#41686=CARTESIAN_POINT ( 'NONE',  ( -59.81910112700027327, -137.3125000027312126, -2.462841084822392279 ) ) ;
#41689=CARTESIAN_POINT ( 'NONE',  ( -58.39396692619412477, -140.6875000013656063, 2.891590998281057701 ) ) ;
#41691=CARTESIAN_POINT ( 'NONE',  ( -51.75738570946856498, -131.8750000027312126, 3.805975901505576964 ) ) ;
#41702=CARTESIAN_POINT ( 'NONE',  ( -57.89159099828107458, -126.6875000013656063, -3.393966926194107447 ) ) ;
#41714=CARTESIAN_POINT ( 'NONE',  ( -59.59170313451811296, -132.5000000013656063, 1.485763867205729394 ) ) ;
#41725=CARTESIAN_POINT ( 'NONE',  ( -50.70258187064364108, -126.3750000013656489, 2.196230717870141014 ) ) ;
#41738=VERTEX_POINT ( 'NONE', #2243 ) ;
#41749=CARTESIAN_POINT ( 'NONE',  ( -52.10840900171896806, -154.4375000013656063, 3.393966926194110556 ) ) ;
#41753=CARTESIAN_POINT ( 'NONE',  ( -50.40829686548195099, -140.0000000013656063, -1.485763867205728284 ) ) ;
#41759=CARTESIAN_POINT ( 'NONE',  ( -56.66612745406270335, -149.3125000000000000, -5.149110718188516067 ) ) ;
#41771=CARTESIAN_POINT ( 'NONE',  ( -58.80597590150559739, -144.1250000027312126, 3.242614290531460330 ) ) ;
#41783=CARTESIAN_POINT ( 'NONE',  ( -57.19623071787017210, -137.3750000013656063, 4.297418129356382899 ) ) ;
#41798=CARTESIAN_POINT ( 'NONE',  ( -57.19623071787017210, -146.3750000013655779, 4.297418129356382899 ) ) ;
#41800=CARTESIAN_POINT ( 'NONE',  ( -54.60164318462004474, -148.3750000000000284, -4.984105922594373794 ) ) ;
#41841=CARTESIAN_POINT ( 'NONE',  ( -57.19623071787017210, -132.6250000013656347, 4.297418129356382899 ) ) ;
#41884=CARTESIAN_POINT ( 'NONE',  ( -50.40829686548195099, -139.2500000013656063, -1.485763867205728284 ) ) ;
#41903=CARTESIAN_POINT ( 'NONE',  ( -57.19623071787016499, -135.6250000013655779, 4.297418129356382899 ) ) ;
#41909=CARTESIAN_POINT ( 'NONE',  ( -58.80597590150559739, -139.0000000000000284, 3.242614290531460330 ) ) ;
#41918=CARTESIAN_POINT ( 'NONE',  ( -50.70258187064364108, -146.3750000013655779, 2.196230717870141014 ) ) ;
#41930=CARTESIAN_POINT ( 'NONE',  ( -59.98410592259440222, -125.1250000000000142, -0.3983568153799752487 ) ) ;
#41938=CARTESIAN_POINT ( 'NONE',  ( -57.19623071787017210, -147.3750000013656063, 4.297418129356382899 ) ) ;
#41953=( BOUNDED_CURVE ( )  B_SPLINE_CURVE ( 2, ( #13943, #55895, #18764, #61044, #62545, #3369, #7007, #51387, #57712 ),
 .UNSPECIFIED., .F., .F. ) 
 B_SPLINE_CURVE_WITH_KNOTS ( ( 3, 2, 2, 2, 3 ),
 ( 0.2750000000000002442, 0.2791666666666668961, 0.2833333333333335480, 0.2875000000000001998, 0.2916666666666669072 ),
 .UNSPECIFIED. ) 
 CURVE ( )  GEOMETRIC_REPRESENTATION_ITEM ( )  RATIONAL_B_SPLINE_CURVE ( ( 0.9999999999999958922, 0.9238795325112908463, 1.000000000000000000, 0.9238795325112867385, 1.000000000000000000, 0.9238795325112867385, 1.000000000000000000, 0.9238795325112826307, 1.000000000000003997 ) ) 
 REPRESENTATION_ITEM ( '' )  );
#41963=CARTESIAN_POINT ( 'NONE',  ( -50.40829686548195099, -153.2500000013655779, -1.485763867205728284 ) ) ;
#41974=CARTESIAN_POINT ( 'NONE',  ( -57.46284108482265651, -152.9375000000000000, 4.819101127000238627 ) ) ;
#41990=CARTESIAN_POINT ( 'NONE',  ( -55.00000000000002132, -135.0000000000000284, 1.734723475976807094E-15 ) ) ;
#42002=CARTESIAN_POINT ( 'NONE',  ( -57.46284108482265651, -135.9375000000000000, 4.819101127000239515 ) ) ;
#42012=CARTESIAN_POINT ( 'NONE',  ( -52.10840900171896806, -140.4375000013656063, 3.393966926194110556 ) ) ;
#42014=CARTESIAN_POINT ( 'NONE',  ( -51.19402409849444524, -132.6250000027312126, -3.242614290531456334 ) ) ;
#42038=( BOUNDED_CURVE ( )  B_SPLINE_CURVE ( 2, ( #47016, #61819, #27076, #37361, #3281, #2966, #60865, #46693, #2640 ),
 .UNSPECIFIED., .F., .F. ) 
 B_SPLINE_CURVE_WITH_KNOTS ( ( 3, 2, 2, 2, 3 ),
 ( 0.1750000000000001554, 0.1791666666666668351, 0.1833333333333334869, 0.1875000000000001665, 0.1916666666666668462 ),
 .UNSPECIFIED. ) 
 CURVE ( )  GEOMETRIC_REPRESENTATION_ITEM ( )  RATIONAL_B_SPLINE_CURVE ( ( 0.9999999999999970024, 0.9238795325112897361, 1.000000000000000000, 0.9238795325112867385, 1.000000000000000000, 0.9238795325112867385, 1.000000000000000000, 0.9238795325112837409, 1.000000000000003109 ) ) 
 REPRESENTATION_ITEM ( '' )  );
#42039=CARTESIAN_POINT ( 'NONE',  ( -57.19623071787017210, -134.3750000013656347, 4.297418129356382899 ) ) ;
#42048=CARTESIAN_POINT ( 'NONE',  ( -50.40829686548195099, -129.2500000013656347, -1.485763867205728284 ) ) ;
#42073=CARTESIAN_POINT ( 'NONE',  ( -57.19623071787017210, -153.6250000013655779, 4.297418129356382899 ) ) ;
#42077=CARTESIAN_POINT ( 'NONE',  ( -59.44456063193725015, -137.5625000013656063, -0.3552334253322034230 ) ) ;
#42082=CARTESIAN_POINT ( 'NONE',  ( -57.46284108482265651, -149.9375000000000284, 4.819101127000239515 ) ) ;
#42092=CARTESIAN_POINT ( 'NONE',  ( -58.24261429053147765, -141.3750000027312126, -3.805975901505573855 ) ) ;
#42098=CARTESIAN_POINT ( 'NONE',  ( -52.10840900171896806, -138.1875000013656347, 3.393966926194110556 ) ) ;
#42113=FACE_OUTER_BOUND ( 'NONE', #45480, .T. ) ;
#42114=CARTESIAN_POINT ( 'NONE',  ( -58.39396692619412477, -146.4375000013656063, 2.891590998281057701 ) ) ;
#42163=CARTESIAN_POINT ( 'NONE',  ( -58.39396692619412477, -131.6875000013656063, 2.891590998281057701 ) ) ;
#42205=CARTESIAN_POINT ( 'NONE',  ( -53.51423613279429503, -137.5000000013656063, 4.591703134518082763 ) ) ;
#42225=CARTESIAN_POINT ( 'NONE',  ( -57.89159099828107458, -135.9375000013656063, -3.393966926194107447 ) ) ;
#42238=CARTESIAN_POINT ( 'NONE',  ( -59.44456063193725015, -144.8125000013656063, -0.3552334253322034230 ) ) ;
#42249=CARTESIAN_POINT ( 'NONE',  ( -53.33387254593728954, -151.8125000000000284, 5.149110718188522284 ) ) ;
#42250=CARTESIAN_POINT ( 'NONE',  ( -57.46284108482265651, -125.9375000000000568, 4.819101127000239515 ) ) ;
#42257=CARTESIAN_POINT ( 'NONE',  ( -58.39396692619412477, -150.4375000013656063, 2.891590998281057701 ) ) ;
#42283=CARTESIAN_POINT ( 'NONE',  ( -52.80376928212989185, -150.1250000013656063, -4.297418129356379346 ) ) ;
#42318=CARTESIAN_POINT ( 'NONE',  ( -55.39835681537999790, -138.8750000000000284, 4.984105922594378235 ) ) ;
#42326=EDGE_LOOP ( 'NONE', ( #5725, #42767, #35087, #62351, #36312, #19670, #26866, #57686, #50384, #7006, #491, #51177, #9416, #18544, #56108, #30120, #32310, #9526, #11851, #55050, #6501, #33384, #38712, #18284, #46020, #10670, #26525, #32781, #30111, #32294, #58735, #21584, #50560, #24858, #42995, #44031, #18673, #9731, #9696, #48012, #27530, #28866, #16796, #39375 ) ) ;
#42328=CARTESIAN_POINT ( 'NONE',  ( -55.35523342533222291, -139.5625000013656063, 4.444560631937231499 ) ) ;
#42330=CARTESIAN_POINT ( 'NONE',  ( -52.53715891517739323, -132.5625000027312126, -4.819101127000233298 ) ) ;
#42343=CARTESIAN_POINT ( 'NONE',  ( -56.48576386720575471, -124.7500000013655921, -4.591703134518078322 ) ) ;
#42355=CARTESIAN_POINT ( 'NONE',  ( -59.29741812935640155, -132.6250000013656347, -2.196230717870135685 ) ) ;
#42365=CARTESIAN_POINT ( 'NONE',  ( -59.59170313451811296, -127.7500000013655921, 1.485763867205729394 ) ) ;
#42386=CARTESIAN_POINT ( 'NONE',  ( -50.40829686548195099, -154.2500000013656063, -1.485763867205728284 ) ) ;
#42390=CARTESIAN_POINT ( 'NONE',  ( -50.70258187064364108, -137.1250000013656063, 2.196230717870141014 ) ) ;
#42395=CARTESIAN_POINT ( 'NONE',  ( -57.46284108482265651, -148.9375000000000000, 4.819101127000239515 ) ) ;
#42403=CARTESIAN_POINT ( 'NONE',  ( -55.35523342533222291, -150.5625000013656063, 4.444560631937231499 ) ) ;
#42404=CARTESIAN_POINT ( 'NONE',  ( -51.19402409849444524, -144.6250000027312126, -3.242614290531456334 ) ) ;
#42413=CARTESIAN_POINT ( 'NONE',  ( -54.64476657466781973, -137.8125000013656063, -4.444560631937228834 ) ) ;
#42428=EDGE_CURVE ( 'NONE', #11960, #35585, #23350, .T. ) ;
#42429=CARTESIAN_POINT ( 'NONE',  ( -50.55543936806279248, -145.0625000013656063, 0.3552334253322060320 ) ) ;
#42455=DIRECTION ( 'NONE',  ( -0.6485228581062915110, 0.000000000000000000, -0.7611951803011149931 ) ) ;
#42471=CARTESIAN_POINT ( 'NONE',  ( -59.44456063193725015, -129.8125000013656063, -0.3552334253322034230 ) ) ;
#42483=CARTESIAN_POINT ( 'NONE',  ( -58.24261429053147765, -148.2500000000000284, -3.805975901505573855 ) ) ;
#42516=CARTESIAN_POINT ( 'NONE',  ( -59.81910112700026616, -145.3125000027311842, -2.462841084822510851 ) ) ;
#42519=CARTESIAN_POINT ( 'NONE',  ( -54.64476657466781973, -135.0625000013656063, -4.444560631937228834 ) ) ;
#42550=CARTESIAN_POINT ( 'NONE',  ( -54.64476657466781973, -145.0625000013656063, -4.444560631937228834 ) ) ;
#42561=CARTESIAN_POINT ( 'NONE',  ( -58.80597590150559739, -127.0000000000000284, 3.242614290531460330 ) ) ;
#42565=VERTEX_POINT ( 'NONE', #53237 ) ;
#42571=CARTESIAN_POINT ( 'NONE',  ( -53.51423613279429503, -146.2500000013656063, 4.591703134518082763 ) ) ;
#42590=VERTEX_POINT ( 'NONE', #54511 ) ;
#42598=( BOUNDED_CURVE ( )  B_SPLINE_CURVE ( 2, ( #28566, #24069, #38237, #53647, #9266, #58478, #39162, #62688, #28253 ),
 .UNSPECIFIED., .F., .F. ) 
 B_SPLINE_CURVE_WITH_KNOTS ( ( 3, 2, 2, 2, 3 ),
 ( 0.4750000000000004219, 0.4791666666666671293, 0.4833333333333337811, 0.4875000000000004330, 0.4916666666666670849 ),
 .UNSPECIFIED. ) 
 CURVE ( )  GEOMETRIC_REPRESENTATION_ITEM ( )  RATIONAL_B_SPLINE_CURVE ( ( 0.9999999999999918954, 0.9238795325112948431, 1.000000000000000000, 0.9238795325112867385, 1.000000000000000000, 0.9238795325112867385, 1.000000000000000000, 0.9238795325112786339, 1.000000000000008216 ) ) 
 REPRESENTATION_ITEM ( '' )  );
#42599=CARTESIAN_POINT ( 'NONE',  ( -50.70258187064364108, -146.3750000013655779, 2.196230717870141014 ) ) ;
#42635=CARTESIAN_POINT ( 'NONE',  ( -49.85088928181150436, -136.5625000000000284, -1.666127454062680702 ) ) ;
#42643=FACE_OUTER_BOUND ( 'NONE', #11210, .T. ) ;
#42644=CARTESIAN_POINT ( 'NONE',  ( -59.44456063193725015, -139.8125000013656063, -0.3552334253322034230 ) ) ;
#42646=CARTESIAN_POINT ( 'NONE',  ( -55.39835681537999790, -132.0000000027312126, 4.984105922594378235 ) ) ;
#42655=CARTESIAN_POINT ( 'NONE',  ( -55.00000000000002132, -155.0000000000000284, 1.734723475976807094E-15 ) ) ;
#42659=CARTESIAN_POINT ( 'NONE',  ( -58.39396692619412477, -125.4375000013656063, 2.891590998281057701 ) ) ;
#42669=CARTESIAN_POINT ( 'NONE',  ( -57.19623071787017210, -128.3750000013656631, 4.297418129356382899 ) ) ;
#42678=CARTESIAN_POINT ( 'NONE',  ( -50.40829686548195099, -127.2500000013656347, -1.485763867205728284 ) ) ;
#42706=( BOUNDED_CURVE ( )  B_SPLINE_CURVE ( 2, ( #51380, #17600, #7322, #17900, #26932, #46549, #57163, #62615, #43590 ),
 .UNSPECIFIED., .F., .F. ) 
 B_SPLINE_CURVE_WITH_KNOTS ( ( 3, 2, 2, 2, 3 ),
 ( 0.02500000000000002220, 0.02916666666666669488, 0.03333333333333336757, 0.03750000000000003331, 0.04166666666666670599 ),
 .UNSPECIFIED. ) 
 CURVE ( )  GEOMETRIC_REPRESENTATION_ITEM ( )  RATIONAL_B_SPLINE_CURVE ( ( 0.9999999999999996669, 0.9238795325112870716, 1.000000000000000000, 0.9238795325112867385, 1.000000000000000000, 0.9238795325112867385, 1.000000000000000000, 0.9238795325112859613, 1.000000000000000666 ) ) 
 REPRESENTATION_ITEM ( '' )  );
#42710=CARTESIAN_POINT ( 'NONE',  ( -51.75738570946856498, -149.7500000000000284, 3.805975901505576964 ) ) ;
#42719=CARTESIAN_POINT ( 'NONE',  ( -51.60603307380591787, -150.1875000013656063, -2.891590998281053704 ) ) ;
#42720=CARTESIAN_POINT ( 'NONE',  ( -55.39835681537999790, -144.0000000027312126, 4.984105922594378235 ) ) ;
#42727=CARTESIAN_POINT ( 'NONE',  ( -53.51423613279429503, -135.2500000013656347, 4.591703134518082763 ) ) ;
#42733=EDGE_LOOP ( 'NONE', ( #62214, #48861, #31191, #58389 ) ) ;
#42739=DIRECTION ( 'NONE',  ( -0.6485228581062916220, 0.000000000000000000, -0.7611951803011147710 ) ) ;
#42745=CARTESIAN_POINT ( 'NONE',  ( -59.44456063193725015, -146.5625000013656063, -0.3552334253322034230 ) ) ;
#42767=ORIENTED_EDGE ( 'NONE', *, *, #20327, .F. ) ;
#42786=CARTESIAN_POINT ( 'NONE',  ( -58.24261429053147765, -149.3750000027312126, -3.805975901505573855 ) ) ;
#42790=CARTESIAN_POINT ( 'NONE',  ( -57.89159099828107458, -132.9375000013656063, -3.393966926194107447 ) ) ;
#42831=CARTESIAN_POINT ( 'NONE',  ( -58.24261429053147765, -145.3750000027312126, -3.805975901505573855 ) ) ;
#42836=CARTESIAN_POINT ( 'NONE',  ( -56.48576386720575471, -136.0000000013656063, -4.591703134518078322 ) ) ;
#42838=CARTESIAN_POINT ( 'NONE',  ( -51.19402409849444524, -145.5000000000000284, -3.242614290531456334 ) ) ;
#42844=ORIENTED_EDGE ( 'NONE', *, *, #56295, .T. ) ;
#42865=CARTESIAN_POINT ( 'NONE',  ( -56.48576386720575471, -144.0000000013656063, -4.591703134518078322 ) ) ;
#42883=CARTESIAN_POINT ( 'NONE',  ( -57.19623071787017210, -143.3750000013656063, 4.297418129356382899 ) ) ;
#42900=CARTESIAN_POINT ( 'NONE',  ( -51.75738570946856498, -139.8750000027312126, 3.805975901505576964 ) ) ;
#42907=CARTESIAN_POINT ( 'NONE',  ( -52.80376928212989185, -146.1250000013656063, -4.297418129356379346 ) ) ;
#42917=CARTESIAN_POINT ( 'NONE',  ( -53.33387254593703375, -137.9375000027311842, 5.149110718188541824 ) ) ;
#42935=EDGE_CURVE ( 'NONE', #27373, #58935, #7535, .T. ) ;
#42941=EDGE_CURVE ( 'NONE', #28080, #46979, #34318, .T. ) ;
#42951=CARTESIAN_POINT ( 'NONE',  ( -51.75738570946856498, -132.7500000000000284, 3.805975901505576964 ) ) ;
#42958=CARTESIAN_POINT ( 'NONE',  ( -57.89159099828107458, -137.9375000013656063, -3.393966926194107447 ) ) ;
#42960=CARTESIAN_POINT ( 'NONE',  ( -58.80597590150559739, -126.1250000027312126, 3.242614290531460330 ) ) ;
#42970=CARTESIAN_POINT ( 'NONE',  ( -55.00000000000002132, -155.0000000000000284, 1.734723475976807094E-15 ) ) ;
#42986=CARTESIAN_POINT ( 'NONE',  ( -54.64476657466781973, -127.8125000013655921, -4.444560631937228834 ) ) ;
#42995=ORIENTED_EDGE ( 'NONE', *, *, #15698, .F. ) ;
#43013=CARTESIAN_POINT ( 'NONE',  ( -51.19402409849444524, -144.6250000027312126, -3.242614290531456334 ) ) ;
#43022=CARTESIAN_POINT ( 'NONE',  ( -53.51423613279429503, -151.5000000013655779, 4.591703134518082763 ) ) ;
#43026=CARTESIAN_POINT ( 'NONE',  ( -59.59170313451810586, -136.5000000013656063, 1.485763867205729394 ) ) ;
#43031=CARTESIAN_POINT ( 'NONE',  ( -52.53715891517739323, -151.4375000000000284, -4.819101127000233298 ) ) ;
#43040=CARTESIAN_POINT ( 'NONE',  ( -50.40829686548195099, -150.2500000013656347, -1.485763867205728284 ) ) ;
#43041=CARTESIAN_POINT ( 'NONE',  ( -55.39835681537999790, -137.0000000027312126, 4.984105922594378235 ) ) ;
#43049=CARTESIAN_POINT ( 'NONE',  ( -56.48576386720575471, -138.7500000013656063, -4.591703134518078322 ) ) ;
#43054=AXIS2_PLACEMENT_3D ( 'NONE', #62200, #38367, #13919 ) ;
#43065=CARTESIAN_POINT ( 'NONE',  ( -59.44456063193725015, -143.5625000013656063, -0.3552334253322034230 ) ) ;
#43096=CARTESIAN_POINT ( 'NONE',  ( -55.00000000000002132, -155.0000000000000284, 1.734723475976807094E-15 ) ) ;
#43104=CARTESIAN_POINT ( 'NONE',  ( -59.29741812935640155, -129.8750000013656063, -2.196230717870135685 ) ) ;
#43110=LINE ( 'NONE', #28940, #46148 ) ;
#43131=CARTESIAN_POINT ( 'NONE',  ( -50.70258187064364108, -152.1250000013656063, 2.196230717870141014 ) ) ;
#43133=FACE_BOUND ( 'NONE', #59325, .T. ) ;
#43142=CARTESIAN_POINT ( 'NONE',  ( -55.39835681537999790, -145.0000000027312126, 4.984105922594378235 ) ) ;
#43146=CARTESIAN_POINT ( 'NONE',  ( -53.51423613279429503, -136.5000000013656347, 4.591703134518082763 ) ) ;
#43166=CARTESIAN_POINT ( 'NONE',  ( -60.14911071818854538, -144.1875000027312410, 1.666127454062681146 ) ) ;
#43170=CARTESIAN_POINT ( 'NONE',  ( -58.24261429053147765, -142.2500000000000284, -3.805975901505573855 ) ) ;
#43176=CARTESIAN_POINT ( 'NONE',  ( -55.35523342533222291, -144.5625000013656063, 4.444560631937231499 ) ) ;
#43194=CARTESIAN_POINT ( 'NONE',  ( -59.44456063193725015, -144.5625000013656063, -0.3552334253322034230 ) ) ;
#43204=ADVANCED_FACE ( 'NONE', ( #35060 ), #59831, .F. ) ;
#43205=CARTESIAN_POINT ( 'NONE',  ( -51.75738570946856498, -142.8750000027312126, 3.805975901505576964 ) ) ;
#43221=CARTESIAN_POINT ( 'NONE',  ( -52.10840900171896806, -149.4375000013656063, 3.393966926194110556 ) ) ;
#43257=CARTESIAN_POINT ( 'NONE',  ( -60.14911071818854538, -134.0625000000000284, 1.666127454062681368 ) ) ;
#43268=CARTESIAN_POINT ( 'NONE',  ( -50.70258187064364108, -137.3750000013656063, 2.196230717870141014 ) ) ;
#43270=CARTESIAN_POINT ( 'NONE',  ( -51.75738570946856498, -127.8750000027312268, 3.805975901505576964 ) ) ;
#43275=CARTESIAN_POINT ( 'NONE',  ( -55.39835681537999790, -151.0000000027312410, 4.984105922594378235 ) ) ;
#43297=CARTESIAN_POINT ( 'NONE',  ( -50.55543936806279248, -131.0625000013656063, 0.3552334253322060320 ) ) ;
#43298=CARTESIAN_POINT ( 'NONE',  ( -57.89159099828107458, -146.6875000013656063, -3.393966926194107447 ) ) ;
#43328=CARTESIAN_POINT ( 'NONE',  ( -56.48576386720575471, -153.0000000013656063, -4.591703134518078322 ) ) ;
#43337=CARTESIAN_POINT ( 'NONE',  ( -49.85088928181150436, -145.5625000000000568, -1.666127454062680702 ) ) ;
#43348=CARTESIAN_POINT ( 'NONE',  ( -57.19623071787016499, -149.6250000013655779, 4.297418129356382899 ) ) ;
#43349=CARTESIAN_POINT ( 'NONE',  ( -50.18089887299979068, -136.8125000027311842, 2.462841084822635640 ) ) ;
#43358=CARTESIAN_POINT ( 'NONE',  ( -58.39396692619412477, -132.4375000013656063, 2.891590998281057701 ) ) ;
#43374=CARTESIAN_POINT ( 'NONE',  ( -51.75738570946856498, -151.7500000000000284, 3.805975901505576964 ) ) ;
#43375=CARTESIAN_POINT ( 'NONE',  ( -55.35523342533222291, -143.3125000013656063, 4.444560631937231499 ) ) ;
#43405=ORIENTED_EDGE ( 'NONE', *, *, #18804, .T. ) ;
#43406=CARTESIAN_POINT ( 'NONE',  ( -59.59170313451810586, -152.5000000013655779, 1.485763867205729394 ) ) ;
#43414=CARTESIAN_POINT ( 'NONE',  ( -58.39396692619412477, -125.6875000013656063, 2.891590998281057701 ) ) ;
#43424=CARTESIAN_POINT ( 'NONE',  ( -55.39835681537999790, -150.0000000027312126, 4.984105922594378235 ) ) ;
#43444=CARTESIAN_POINT ( 'NONE',  ( -54.64476657466781973, -151.8125000013656063, -4.444560631937228834 ) ) ;
#43458=CARTESIAN_POINT ( 'NONE',  ( -52.80376928212989185, -137.1250000013655779, -4.297418129356379346 ) ) ;
#43464=CARTESIAN_POINT ( 'NONE',  ( -59.98410592259440222, -140.1250000000000284, -0.3983568153799752487 ) ) ;
#43472=EDGE_CURVE ( 'NONE', #12526, #55226, #51262, .T. ) ;
#43478=CARTESIAN_POINT ( 'NONE',  ( -55.39835681537999790, -144.0000000027312126, 4.984105922594378235 ) ) ;
#43488=CARTESIAN_POINT ( 'NONE',  ( -50.40829686548195099, -141.2500000013656347, -1.485763867205728284 ) ) ;
#43504=CARTESIAN_POINT ( 'NONE',  ( -54.64476657466781973, -144.8125000013656063, -4.444560631937228834 ) ) ;
#43517=CARTESIAN_POINT ( 'NONE',  ( -48.00000000000002132, -135.0000000000000284, 4.041451884327384114 ) ) ;
#43529=CARTESIAN_POINT ( 'NONE',  ( -59.44456063193725015, -146.8125000013656063, -0.3552334253322034230 ) ) ;
#43533=CARTESIAN_POINT ( 'NONE',  ( -55.39835681537999790, -136.8750000000000284, 4.984105922594378235 ) ) ;
#43550=CARTESIAN_POINT ( 'NONE',  ( -50.01589407740564042, -145.7500000027312126, 0.3983568153799778022 ) ) ;
#43553=CARTESIAN_POINT ( 'NONE',  ( -51.75738570946856498, -135.8750000027312410, 3.805975901505576964 ) ) ;
#43566=CARTESIAN_POINT ( 'NONE',  ( -51.75738570946856498, -131.7500000000000284, 3.805975901505576964 ) ) ;
#43577=CARTESIAN_POINT ( 'NONE',  ( -51.75738570946856498, -126.8750000027312126, 3.805975901505576964 ) ) ;
#43590=CARTESIAN_POINT ( 'NONE',  ( -51.75738570946856498, -153.7500000000000284, 3.805975901505576964 ) ) ;
#43601=CARTESIAN_POINT ( 'NONE',  ( -55.35523342533222291, -129.3125000013656063, 4.444560631937231499 ) ) ;
#43602=CARTESIAN_POINT ( 'NONE',  ( -57.19623071787016499, -145.3750000013656063, 4.297418129356382899 ) ) ;
#43629=CARTESIAN_POINT ( 'NONE',  ( -49.85088928181150436, -144.6875000027312410, -1.666127454062680480 ) ) ;
#43637=CARTESIAN_POINT ( 'NONE',  ( -57.89159099828107458, -151.9375000013656063, -3.393966926194107447 ) ) ;
#43643=CARTESIAN_POINT ( 'NONE',  ( -53.51423613279429503, -135.2500000013656347, 4.591703134518083651 ) ) ;
#43648=CARTESIAN_POINT ( 'NONE',  ( -58.24261429053147765, -146.2500000000000284, -3.805975901505573855 ) ) ;
#43655=CARTESIAN_POINT ( 'NONE',  ( -53.51423613279429503, -149.5000000013656063, 4.591703134518083651 ) ) ;
#43656=CARTESIAN_POINT ( 'NONE',  ( -59.98410592259440222, -138.2500000027312126, -0.3983568153799752487 ) ) ;
#43666=CARTESIAN_POINT ( 'NONE',  ( -50.70258187064364108, -133.1250000013656063, 2.196230717870141014 ) ) ;
#43681=CARTESIAN_POINT ( 'NONE',  ( -52.80376928212989185, -140.8750000013656063, -4.297418129356379346 ) ) ;
#43685=LINE ( 'NONE', #53668, #30486 ) ;
#43726=CARTESIAN_POINT ( 'NONE',  ( -52.10840900171896806, -127.4375000013656063, 3.393966926194110556 ) ) ;
#43734=FACE_OUTER_BOUND ( 'NONE', #21457, .T. ) ;
#43736=CARTESIAN_POINT ( 'NONE',  ( -51.75738570946856498, -155.0000000000000284, 3.805975901505577408 ) ) ;
#43738=CARTESIAN_POINT ( 'NONE',  ( -56.66612745406270335, -150.4375000027312126, -5.149110718188516067 ) ) ;
#43770=CARTESIAN_POINT ( 'NONE',  ( -59.59170313451811296, -132.7500000013656063, 1.485763867205729394 ) ) ;
#43772=CARTESIAN_POINT ( 'NONE',  ( -49.85088928181150436, -145.5625000000000568, -1.666127454062680480 ) ) ;
#43782=DIRECTION ( 'NONE',  ( 0.000000000000000000, 1.000000000000000000, 0.000000000000000000 ) ) ;
#43800=CARTESIAN_POINT ( 'NONE',  ( -51.60603307380591787, -139.1875000013656347, -2.891590998281053704 ) ) ;
#43812=CARTESIAN_POINT ( 'NONE',  ( -58.24261429053147765, -155.0000000000000284, -3.805975901505573411 ) ) ;
#43819=CARTESIAN_POINT ( 'NONE',  ( -57.89159099828107458, -146.6875000013656063, -3.393966926194107447 ) ) ;
#43836=CARTESIAN_POINT ( 'NONE',  ( -53.33387254593719717, -143.8125000000000284, 5.149110718188530278 ) ) ;
#43842=CARTESIAN_POINT ( 'NONE',  ( -57.89159099828107458, -147.9375000013656063, -3.393966926194107447 ) ) ;
#43847=CARTESIAN_POINT ( 'NONE',  ( -58.24261429053147765, -148.2500000000000284, -3.805975901505573855 ) ) ;
#43879=CARTESIAN_POINT ( 'NONE',  ( -53.33387254593733928, -134.8125000000000568, 5.149110718188519620 ) ) ;
#43888=CARTESIAN_POINT ( 'NONE',  ( -50.01589407740564042, -126.7500000027312126, 0.3983568153799778022 ) ) ;
#43890=CARTESIAN_POINT ( 'NONE',  ( -50.44383482147011222, -135.0000000000000000, 0.1418284928502891451 ) ) ;
#43915=CARTESIAN_POINT ( 'NONE',  ( -52.80376928212989185, -130.8750000013656063, -4.297418129356379346 ) ) ;
#43917=CARTESIAN_POINT ( 'NONE',  ( -50.55543936806279248, -146.0625000013656063, 0.3552334253322060320 ) ) ;
#43928=CARTESIAN_POINT ( 'NONE',  ( -57.89159099828107458, -125.9375000013656063, -3.393966926194107447 ) ) ;
#43949=CARTESIAN_POINT ( 'NONE',  ( -59.59170313451811296, -150.7500000013655495, 1.485763867205729394 ) ) ;
#43954=CARTESIAN_POINT ( 'NONE',  ( -59.29741812935640155, -136.6250000013656063, -2.196230717870135685 ) ) ;
#43956=( BOUNDED_CURVE ( )  B_SPLINE_CURVE ( 2, ( #23473, #8055, #3234, #61772, #14114, #22851, #38556, #33741, #18938 ),
 .UNSPECIFIED., .F., .F. ) 
 B_SPLINE_CURVE_WITH_KNOTS ( ( 3, 2, 2, 2, 3 ),
 ( 0.1916666666666668462, 0.1958333333333334980, 0.2000000000000001776, 0.2041666666666668295, 0.2083333333333335091 ),
 .UNSPECIFIED. ) 
 CURVE ( )  GEOMETRIC_REPRESENTATION_ITEM ( )  RATIONAL_B_SPLINE_CURVE ( ( 0.9999999999999970024, 0.9238795325112897361, 1.000000000000000000, 0.9238795325112867385, 1.000000000000000000, 0.9238795325112867385, 1.000000000000000000, 0.9238795325112837409, 1.000000000000003109 ) ) 
 REPRESENTATION_ITEM ( '' )  );
#43960=CARTESIAN_POINT ( 'NONE',  ( -50.01589407740564042, -146.6250000000000284, 0.3983568153799778022 ) ) ;
#43961=AXIS2_PLACEMENT_3D ( 'NONE', #13985, #57446, #33615 ) ;
#43968=VERTEX_POINT ( 'NONE', #28652 ) ;
#43969=CARTESIAN_POINT ( 'NONE',  ( -56.48576386720575471, -147.0000000013656063, -4.591703134518078322 ) ) ;
#43970=CARTESIAN_POINT ( 'NONE',  ( -56.66612745406270335, -138.4375000027312126, -5.149110718188516067 ) ) ;
#43974=CARTESIAN_POINT ( 'NONE',  ( -59.81910112700024484, -135.1875000000000284, -2.462841084822808835 ) ) ;
#43982=CARTESIAN_POINT ( 'NONE',  ( -58.39396692619412477, -133.4375000013656063, 2.891590998281057701 ) ) ;
#43984=CARTESIAN_POINT ( 'NONE',  ( -60.14911071818854538, -146.1875000027312126, 1.666127454062681146 ) ) ;
#43988=ORIENTED_EDGE ( 'NONE', *, *, #14786, .T. ) ;
#43994=CARTESIAN_POINT ( 'NONE',  ( -58.24261429053147765, -143.3750000027312126, -3.805975901505573855 ) ) ;
#43998=CARTESIAN_POINT ( 'NONE',  ( -59.59170313451811296, -143.5000000013656347, 1.485763867205729394 ) ) ;
#44031=ORIENTED_EDGE ( 'NONE', *, *, #14941, .F. ) ;
#44032=CARTESIAN_POINT ( 'NONE',  ( -50.40829686548195099, -152.0000000013656063, -1.485763867205728284 ) ) ;
#44036=CARTESIAN_POINT ( 'NONE',  ( -51.19402409849444524, -149.6250000027312126, -3.242614290531456334 ) ) ;
#44039=CARTESIAN_POINT ( 'NONE',  ( -55.35523342533222291, -126.5625000013655921, 4.444560631937231499 ) ) ;
#44042=CARTESIAN_POINT ( 'NONE',  ( -49.85088928181150436, -136.6875000027312126, -1.666127454062680480 ) ) ;
#44049=CARTESIAN_POINT ( 'NONE',  ( -50.18089887299979068, -151.8125000027312126, 2.462841084822635640 ) ) ;
#44056=DIRECTION ( 'NONE',  ( 0.8660254037844385966, 0.000000000000000000, 0.4999999999999999445 ) ) ;
#44071=FACE_OUTER_BOUND ( 'NONE', #53545, .T. ) ;
#44084=CARTESIAN_POINT ( 'NONE',  ( -51.19402409849444524, -142.5000000000000284, -3.242614290531456334 ) ) ;
#44092=CARTESIAN_POINT ( 'NONE',  ( -50.18089887299979068, -151.8125000027312126, 2.462841084822605442 ) ) ;
#44095=DIRECTION ( 'NONE',  ( -0.000000000000000000, 0.000000000000000000, -1.000000000000000000 ) ) ;
#44117=CARTESIAN_POINT ( 'NONE',  ( -58.39396692619412477, -139.6875000013656347, 2.891590998281057701 ) ) ;
#44128=FACE_OUTER_BOUND ( 'NONE', #59655, .T. ) ;
#44136=CARTESIAN_POINT ( 'NONE',  ( -59.59170313451811296, -139.5000000013656063, 1.485763867205729394 ) ) ;
#44139=VERTEX_POINT ( 'NONE', #6762 ) ;
#44158=EDGE_CURVE ( 'NONE', #27913, #7221, #7301, .T. ) ;
#44160=CARTESIAN_POINT ( 'NONE',  ( -58.24261429053147765, -154.2500000000000284, -3.805975901505573855 ) ) ;
#44164=CARTESIAN_POINT ( 'NONE',  ( -52.80376928212989185, -142.1250000013656063, -4.297418129356379346 ) ) ;
#44176=VERTEX_POINT ( 'NONE', #50179 ) ;
#44187=VECTOR ( 'NONE', #53414, 1000.000000000000000 ) ;
#44204=CARTESIAN_POINT ( 'NONE',  ( -59.98410592259440222, -134.1250000000000284, -0.3983568153799752487 ) ) ;
#44210=CARTESIAN_POINT ( 'NONE',  ( -50.01589407740564042, -149.6250000000000284, 0.3983568153799778022 ) ) ;
#44213=CARTESIAN_POINT ( 'NONE',  ( -54.60164318462004474, -125.5000000027311984, -4.984105922594373794 ) ) ;
#44215=CARTESIAN_POINT ( 'NONE',  ( -54.61975348727955293, -134.9999999999999716, 4.958636921927378260 ) ) ;
#44216=CARTESIAN_POINT ( 'NONE',  ( -48.00000000000002132, -135.0000000000000284, 4.041451884327384114 ) ) ;
#44234=VECTOR ( 'NONE', #35986, 1000.000000000000227 ) ;
#44238=CARTESIAN_POINT ( 'NONE',  ( -50.55543936806279248, -127.0625000013655921, 0.3552334253322060320 ) ) ;
#44239=CARTESIAN_POINT ( 'NONE',  ( -53.51423613279429503, -145.2500000013656347, 4.591703134518083651 ) ) ;
#44250=CARTESIAN_POINT ( 'NONE',  ( -50.40829686548195099, -125.2500000013656347, -1.485763867205728284 ) ) ;
#44265=LINE ( 'NONE', #48469, #51169 ) ;
#44273=CARTESIAN_POINT ( 'NONE',  ( -51.60603307380591787, -152.1875000013656063, -2.891590998281053704 ) ) ;
#44284=CARTESIAN_POINT ( 'NONE',  ( -58.24261429053147765, -147.2500000000000284, -3.805975901505573855 ) ) ;
#44292=CARTESIAN_POINT ( 'NONE',  ( -52.80376928212989185, -145.1250000013656063, -4.297418129356378458 ) ) ;
#44293=CARTESIAN_POINT ( 'NONE',  ( -59.98410592259440222, -137.2500000027312126, -0.3983568153799752487 ) ) ;
#44299=ORIENTED_EDGE ( 'NONE', *, *, #30353, .F. ) ;
#44303=CARTESIAN_POINT ( 'NONE',  ( -51.75738570946856498, -153.7500000000000284, 3.805975901505576964 ) ) ;
#44304=CARTESIAN_POINT ( 'NONE',  ( -50.40829686548195099, -132.0000000013656063, -1.485763867205728284 ) ) ;
#44306=CARTESIAN_POINT ( 'NONE',  ( -58.24261429053147765, -146.3750000027312126, -3.805975901505573855 ) ) ;
#44319=CARTESIAN_POINT ( 'NONE',  ( -57.89159099828107458, -136.6875000013656063, -3.393966926194107447 ) ) ;
#44358=CARTESIAN_POINT ( 'NONE',  ( -58.39396692619412477, -127.6875000013656063, 2.891590998281057701 ) ) ;
#44366=CARTESIAN_POINT ( 'NONE',  ( -58.24261429053147765, -150.2500000000000284, -3.805975901505573855 ) ) ;
#44367=VERTEX_POINT ( 'NONE', #14046 ) ;
#44370=CARTESIAN_POINT ( 'NONE',  ( -58.80597590150559739, -150.1250000027312126, 3.242614290531460330 ) ) ;
#44413=CARTESIAN_POINT ( 'NONE',  ( -59.82678653332929741, -135.0000000000000284, 0.3596868101039389365 ) ) ;
#44438=CARTESIAN_POINT ( 'NONE',  ( -57.89159099828107458, -139.9375000013656063, -3.393966926194107447 ) ) ;
#44439=EDGE_CURVE ( 'NONE', #54748, #41738, #26240, .T. ) ;
#44458=CARTESIAN_POINT ( 'NONE',  ( -53.51423613279429503, -139.2500000013656063, 4.591703134518082763 ) ) ;
#44482=CARTESIAN_POINT ( 'NONE',  ( -54.64476657466781973, -144.0625000013656063, -4.444560631937228834 ) ) ;
#44525=CARTESIAN_POINT ( 'NONE',  ( -56.66612745406270335, -130.3125000000000284, -5.149110718188516067 ) ) ;
#44536=CARTESIAN_POINT ( 'NONE',  ( -56.48576386720575471, -152.7500000013655779, -4.591703134518078322 ) ) ;
#44559=CARTESIAN_POINT ( 'NONE',  ( -58.39396692619412477, -125.4375000013656063, 2.891590998281057701 ) ) ;
#44560=CARTESIAN_POINT ( 'NONE',  ( -59.44456063193725015, -146.5625000013656063, -0.3552334253322034230 ) ) ;
#44592=CARTESIAN_POINT ( 'NONE',  ( -59.59170313451811296, -146.7500000013655495, 1.485763867205729394 ) ) ;
#44602=CARTESIAN_POINT ( 'NONE',  ( -50.01589407740564042, -143.6250000000000284, 0.3983568153799778022 ) ) ;
#44611=CARTESIAN_POINT ( 'NONE',  ( -52.10840900171896806, -145.4375000013656063, 3.393966926194110556 ) ) ;
#44613=CARTESIAN_POINT ( 'NONE',  ( -59.81910112700025905, -135.3125000027312126, -2.462841084822630311 ) ) ;
#44618=CARTESIAN_POINT ( 'NONE',  ( -58.24261429053147765, -135.2500000000000284, -3.805975901505573855 ) ) ;
#44626=CARTESIAN_POINT ( 'NONE',  ( -53.51423613279429503, -133.2500000013656347, 4.591703134518082763 ) ) ;
#44641=CARTESIAN_POINT ( 'NONE',  ( -53.51423613279429503, -139.2500000013656063, 4.591703134518082763 ) ) ;
#44673=CARTESIAN_POINT ( 'NONE',  ( -57.19623071787016499, -151.3750000013656063, 4.297418129356382899 ) ) ;
#44680=CARTESIAN_POINT ( 'NONE',  ( -54.64476657466781973, -126.0625000013655921, -4.444560631937228834 ) ) ;
#44686=CARTESIAN_POINT ( 'NONE',  ( -58.80597590150559739, -150.0000000000000284, 3.242614290531460330 ) ) ;
#44690=CARTESIAN_POINT ( 'NONE',  ( -50.18089887299979068, -150.8125000027311842, 2.462841084822635640 ) ) ;
#44692=ORIENTED_EDGE ( 'NONE', *, *, #15698, .T. ) ;
#44709=CARTESIAN_POINT ( 'NONE',  ( -50.55543936806279248, -149.0625000013656063, 0.3552334253322060320 ) ) ;
#44711=CARTESIAN_POINT ( 'NONE',  ( -50.18089887299978358, -148.6875000000000000, 2.462841084822545934 ) ) ;
#44722=CARTESIAN_POINT ( 'NONE',  ( -52.53715891517739323, -142.4375000000000000, -4.819101127000233298 ) ) ;
#44732=FACE_OUTER_BOUND ( 'NONE', #21911, .T. ) ;
#44734=ORIENTED_EDGE ( 'NONE', *, *, #38220, .T. ) ;
#44739=ADVANCED_FACE ( 'NONE', ( #17231 ), #56485, .F. ) ;
#44756=CARTESIAN_POINT ( 'NONE',  ( -50.40829686548195099, -139.2500000013656063, -1.485763867205728284 ) ) ;
#44764=CARTESIAN_POINT ( 'NONE',  ( -54.35296922496373639, -135.0000000000000000, -4.421185004030076193 ) ) ;
#44767=CARTESIAN_POINT ( 'NONE',  ( -51.75738570946856498, -140.7500000000000000, 3.805975901505576964 ) ) ;
#44776=CARTESIAN_POINT ( 'NONE',  ( -53.51423613279429503, -141.2500000013656347, 4.591703134518082763 ) ) ;
#44804=AXIS2_PLACEMENT_3D ( 'NONE', #32146, #52721, #17048 ) ;
#44805=CARTESIAN_POINT ( 'NONE',  ( -55.35523342533222291, -144.5625000013656063, 4.444560631937231499 ) ) ;
#44808=EDGE_CURVE ( 'NONE', #1423, #59424, #14594, .T. ) ;
#44840=CARTESIAN_POINT ( 'NONE',  ( -52.53715891517739323, -141.4375000000000284, -4.819101127000233298 ) ) ;
#44846=CARTESIAN_POINT ( 'NONE',  ( -49.85088928181150436, -131.5625000000000284, -1.666127454062680702 ) ) ;
#44856=CARTESIAN_POINT ( 'NONE',  ( -50.40829686548195099, -153.0000000013656063, -1.485763867205728284 ) ) ;
#44859=CARTESIAN_POINT ( 'NONE',  ( -62.00000000000001421, -135.0000000000000284, -4.041451884327373456 ) ) ;
#44869=CARTESIAN_POINT ( 'NONE',  ( -59.81910112700026616, -145.1874999999999716, -2.462841084822481541 ) ) ;
#44887=CARTESIAN_POINT ( 'NONE',  ( -59.44456063193725015, -127.5625000013655921, -0.3552334253322034230 ) ) ;
#44888=CARTESIAN_POINT ( 'NONE',  ( -59.44456063193725015, -142.5625000013656063, -0.3552334253322034230 ) ) ;
#44932=CARTESIAN_POINT ( 'NONE',  ( -58.80597590150559739, -142.0000000000000284, 3.242614290531460330 ) ) ;
#44940=CARTESIAN_POINT ( 'NONE',  ( -57.89159099828107458, -145.9375000013656063, -3.393966926194107447 ) ) ;
#44942=CARTESIAN_POINT ( 'NONE',  ( -59.81910112700025905, -134.3125000027312126, -2.462841084822630311 ) ) ;
#44956=CARTESIAN_POINT ( 'NONE',  ( -56.48576386720575471, -127.7500000013655921, -4.591703134518078322 ) ) ;
#44963=VERTEX_POINT ( 'NONE', #32130 ) ;
#44970=CARTESIAN_POINT ( 'NONE',  ( -52.10840900171896806, -138.1875000013656347, 3.393966926194110556 ) ) ;
#44979=CARTESIAN_POINT ( 'NONE',  ( -50.40829686548195099, -130.2500000013656063, -1.485763867205728284 ) ) ;
#44984=CARTESIAN_POINT ( 'NONE',  ( -58.24261429053147765, -155.0000000000000284, -3.805975901505573411 ) ) ;
#44988=CARTESIAN_POINT ( 'NONE',  ( -49.85088928181150436, -151.5625000000000284, -1.666127454062680480 ) ) ;
#45004=CARTESIAN_POINT ( 'NONE',  ( -55.35523342533222291, -150.3125000013656063, 4.444560631937231499 ) ) ;
#45011=CARTESIAN_POINT ( 'NONE',  ( -49.85088928181150436, -153.5625000000000284, -1.666127454062680702 ) ) ;
#45014=CARTESIAN_POINT ( 'NONE',  ( -54.60164318462004474, -136.5000000027312126, -4.984105922594373794 ) ) ;
#45021=CARTESIAN_POINT ( 'NONE',  ( -53.33387254593733928, -145.9375000027312126, 5.149110718188519620 ) ) ;
#45036=CARTESIAN_POINT ( 'NONE',  ( -58.24261429053147765, -143.2500000000000284, -3.805975901505573855 ) ) ;
#45039=CARTESIAN_POINT ( 'NONE',  ( -50.70258187064364108, -151.1250000013655779, 2.196230717870141014 ) ) ;
#45073=ORIENTED_EDGE ( 'NONE', *, *, #38544, .T. ) ;
#45087=CARTESIAN_POINT ( 'NONE',  ( -59.29741812935640155, -140.8750000013656063, -2.196230717870135685 ) ) ;
#45103=CARTESIAN_POINT ( 'NONE',  ( -59.29741812935640155, -140.6250000013656063, -2.196230717870135685 ) ) ;
#45129=CARTESIAN_POINT ( 'NONE',  ( -50.55543936806279248, -144.3125000013656063, 0.3552334253322060320 ) ) ;
#45171=CARTESIAN_POINT ( 'NONE',  ( -58.24261429053147765, -130.2500000000000284, -3.805975901505573855 ) ) ;
#45179=CARTESIAN_POINT ( 'NONE',  ( -52.10840900171896806, -152.1875000013656063, 3.393966926194110556 ) ) ;
#45181=CARTESIAN_POINT ( 'NONE',  ( -59.98410592259440222, -147.2500000027312126, -0.3983568153799752487 ) ) ;
#45194=VERTEX_POINT ( 'NONE', #4439 ) ;
#45203=CARTESIAN_POINT ( 'NONE',  ( -52.10840900171896806, -127.1875000013656063, 3.393966926194110556 ) ) ;
#45204=CARTESIAN_POINT ( 'NONE',  ( -57.19623071787016499, -141.3750000013656063, 4.297418129356382899 ) ) ;
#45234=EDGE_CURVE ( 'NONE', #27373, #24115, #42598, .T. ) ;
#45245=CARTESIAN_POINT ( 'NONE',  ( -59.81910112700025905, -142.1875000000000284, -2.462841084822630311 ) ) ;
#45252=EDGE_CURVE ( 'NONE', #42565, #44963, #3541, .T. ) ;
#45257=CARTESIAN_POINT ( 'NONE',  ( -53.51423613279429503, -146.5000000013656347, 4.591703134518083651 ) ) ;
#45259=CARTESIAN_POINT ( 'NONE',  ( -58.80597590150559739, -134.1250000027312126, 3.242614290531460330 ) ) ;
#45271=CARTESIAN_POINT ( 'NONE',  ( -50.70258187064364108, -129.1250000013655779, 2.196230717870141014 ) ) ;
#45285=CARTESIAN_POINT ( 'NONE',  ( -59.29741812935640155, -137.6250000013655779, -2.196230717870135685 ) ) ;
#45295=CARTESIAN_POINT ( 'NONE',  ( -55.35523342533222291, -130.5625000013656063, 4.444560631937231499 ) ) ;
#45320=ORIENTED_EDGE ( 'NONE', *, *, #45234, .T. ) ;
#45322=CARTESIAN_POINT ( 'NONE',  ( -50.70258187064364108, -150.1250000013656063, 2.196230717870141014 ) ) ;
#45329=CARTESIAN_POINT ( 'NONE',  ( -53.33387254593733928, -154.8125000000000000, 5.149110718188519620 ) ) ;
#45340=CARTESIAN_POINT ( 'NONE',  ( -59.98410592259440222, -146.2500000027312126, -0.3983568153799752487 ) ) ;
#45344=EDGE_LOOP ( 'NONE', ( #24519, #11197, #55560, #44692 ) ) ;
#45358=AXIS2_PLACEMENT_3D ( 'NONE', #42655, #3748, #48421 ) ;
#45360=CARTESIAN_POINT ( 'NONE',  ( -56.48576386720575471, -148.7500000013655779, -4.591703134518078322 ) ) ;
#45377=CYLINDRICAL_SURFACE ( 'NONE', #54261, 5.000000000000000000 ) ;
#45405=CARTESIAN_POINT ( 'NONE',  ( -58.39396692619412477, -133.6875000013656063, 2.891590998281057701 ) ) ;
#45423=CARTESIAN_POINT ( 'NONE',  ( -59.44456063193725015, -139.5625000013656063, -0.3552334253322034230 ) ) ;
#45449=CARTESIAN_POINT ( 'NONE',  ( -52.10840900171896806, -138.4375000013656063, 3.393966926194110556 ) ) ;
#45451=CARTESIAN_POINT ( 'NONE',  ( -58.24261429053147765, -155.0000000000000284, -3.805975901505573411 ) ) ;
#45475=CARTESIAN_POINT ( 'NONE',  ( -56.66612745406251861, -135.4375000027312126, -5.149110718188501856 ) ) ;
#45480=EDGE_LOOP ( 'NONE', ( #5522, #30506, #46055, #3895 ) ) ;
#45484=CARTESIAN_POINT ( 'NONE',  ( -49.85088928181150436, -141.5625000000000568, -1.666127454062680480 ) ) ;
#45490=CARTESIAN_POINT ( 'NONE',  ( -56.66612745406270335, -131.3125000000000284, -5.149110718188516067 ) ) ;
#45497=CARTESIAN_POINT ( 'NONE',  ( -50.70258187064364108, -151.1250000013655779, 2.196230717870141014 ) ) ;
#45510=CARTESIAN_POINT ( 'NONE',  ( -56.66612745406293783, -138.3125000000000000, -5.149110718188535607 ) ) ;
#45523=CARTESIAN_POINT ( 'NONE',  ( -50.55543936806279248, -125.0625000013655921, 0.3552334253322060320 ) ) ;
#45524=CARTESIAN_POINT ( 'NONE',  ( -50.70258187064364108, -141.1250000013656063, 2.196230717870141014 ) ) ;
#45563=CARTESIAN_POINT ( 'NONE',  ( -51.75738570946856498, -142.7500000000000284, 3.805975901505576964 ) ) ;
#45574=CARTESIAN_POINT ( 'NONE',  ( -51.60603307380591787, -141.1875000013656063, -2.891590998281053704 ) ) ;
#45576=CARTESIAN_POINT ( 'NONE',  ( -57.46284108482265651, -135.0625000027312410, 4.819101127000239515 ) ) ;
#45589=CARTESIAN_POINT ( 'NONE',  ( -51.60603307380591787, -128.9375000013656063, -2.891590998281053704 ) ) ;
#45591=CARTESIAN_POINT ( 'NONE',  ( -60.14911071818854538, -142.1875000027312126, 1.666127454062681146 ) ) ;
#45605=CARTESIAN_POINT ( 'NONE',  ( -50.70258187064364108, -136.1250000013656063, 2.196230717870141014 ) ) ;
#45617=CARTESIAN_POINT ( 'NONE',  ( -59.29741812935640155, -133.8750000013656063, -2.196230717870135685 ) ) ;
#45649=CARTESIAN_POINT ( 'NONE',  ( -50.18089887299979068, -154.6875000000000568, 2.462841084822635640 ) ) ;
#45660=CARTESIAN_POINT ( 'NONE',  ( -51.75738570946856498, -146.8750000027312126, 3.805975901505576964 ) ) ;
#45678=CARTESIAN_POINT ( 'NONE',  ( -57.19623071787017210, -150.3750000013656063, 4.297418129356382899 ) ) ;
#45682=CARTESIAN_POINT ( 'NONE',  ( -52.53715891517739323, -148.4375000000000000, -4.819101127000233298 ) ) ;
#45704=EDGE_CURVE ( 'NONE', #38280, #42565, #42706, .T. ) ;
#45717=ORIENTED_EDGE ( 'NONE', *, *, #30216, .F. ) ;
#45729=CARTESIAN_POINT ( 'NONE',  ( -50.55543936806279248, -135.3125000013656063, 0.3552334253322060320 ) ) ;
#45769=CARTESIAN_POINT ( 'NONE',  ( -57.89159099828107458, -141.9375000013656063, -3.393966926194107447 ) ) ;
#45789=CARTESIAN_POINT ( 'NONE',  ( -55.35523342533222291, -135.5625000013656063, 4.444560631937231499 ) ) ;
#45796=CARTESIAN_POINT ( 'NONE',  ( -50.01589407740564042, -135.7500000027312126, 0.3983568153799778022 ) ) ;
#45800=CARTESIAN_POINT ( 'NONE',  ( -50.55543936806279248, -147.3125000013656063, 0.3552334253322060320 ) ) ;
#45811=CARTESIAN_POINT ( 'NONE',  ( -57.46284108482265651, -127.9375000000000568, 4.819101127000239515 ) ) ;
#45819=CARTESIAN_POINT ( 'NONE',  ( -58.39396692619412477, -152.4375000013656063, 2.891590998281057701 ) ) ;
#45828=CARTESIAN_POINT ( 'NONE',  ( -50.01589407740564042, -152.7500000027312410, 0.3983568153799778022 ) ) ;
#45836=CARTESIAN_POINT ( 'NONE',  ( -48.00000000000002132, -135.0000000000000284, 4.041451884327384114 ) ) ;
#45843=CARTESIAN_POINT ( 'NONE',  ( -52.80376928212989185, -153.1250000013656063, -4.297418129356379346 ) ) ;
#45844=CARTESIAN_POINT ( 'NONE',  ( -57.89159099828107458, -144.6875000013656063, -3.393966926194107447 ) ) ;
#45847=CARTESIAN_POINT ( 'NONE',  ( -59.98410592259440222, -137.1250000000000284, -0.3983568153799752487 ) ) ;
#45875=EDGE_LOOP ( 'NONE', ( #4679, #4125, #253, #38637 ) ) ;
#45881=CARTESIAN_POINT ( 'NONE',  ( -60.14911071818854538, -142.0625000000000000, 1.666127454062681368 ) ) ;
#45891=CARTESIAN_POINT ( 'NONE',  ( -59.59170313451810586, -141.7500000013656063, 1.485763867205729394 ) ) ;
#45893=CARTESIAN_POINT ( 'NONE',  ( -58.80597590150559739, -136.1250000027312410, 3.242614290531460330 ) ) ;
#45907=CARTESIAN_POINT ( 'NONE',  ( -54.64476657466781973, -129.8125000013656063, -4.444560631937228834 ) ) ;
#45914=FACE_OUTER_BOUND ( 'NONE', #25614, .T. ) ;
#45921=CARTESIAN_POINT ( 'NONE',  ( -59.44456063193725015, -135.5625000013656063, -0.3552334253322034230 ) ) ;
#45931=CARTESIAN_POINT ( 'NONE',  ( -59.59170313451811296, -130.7500000013656063, 1.485763867205729394 ) ) ;
#45956=CARTESIAN_POINT ( 'NONE',  ( -50.40829686548195099, -139.0000000013655779, -1.485763867205728284 ) ) ;
#45963=CARTESIAN_POINT ( 'NONE',  ( -59.98410592259440222, -154.1250000000000284, -0.3983568153799752487 ) ) ;
#45976=CARTESIAN_POINT ( 'NONE',  ( -56.66612745406270335, -146.4375000027312126, -5.149110718188516067 ) ) ;
#45996=CARTESIAN_POINT ( 'NONE',  ( -53.51423613279429503, -151.2500000013656063, 4.591703134518082763 ) ) ;
#46020=ORIENTED_EDGE ( 'NONE', *, *, #46137, .F. ) ;
#46026=CYLINDRICAL_SURFACE ( 'NONE', #18505, 5.000000000000000000 ) ;
#46040=CARTESIAN_POINT ( 'NONE',  ( -52.80376928212989185, -137.1250000013655779, -4.297418129356379346 ) ) ;
#46055=ORIENTED_EDGE ( 'NONE', *, *, #45252, .T. ) ;
#46086=CARTESIAN_POINT ( 'NONE',  ( -59.29741812935640155, -140.8750000013656063, -2.196230717870135685 ) ) ;
#46096=ORIENTED_EDGE ( 'NONE', *, *, #9968, .T. ) ;
#46107=CARTESIAN_POINT ( 'NONE',  ( -51.60603307380591787, -135.1875000013656063, -2.891590998281053704 ) ) ;
#46118=CARTESIAN_POINT ( 'NONE',  ( -54.64476657466781973, -149.0625000013656063, -4.444560631937228834 ) ) ;
#46130=CARTESIAN_POINT ( 'NONE',  ( -60.14911071818854538, -127.0625000000000142, 1.666127454062681368 ) ) ;
#46137=EDGE_CURVE ( 'NONE', #44176, #41301, #22134, .T. ) ;
#46139=CARTESIAN_POINT ( 'NONE',  ( -51.60603307380591787, -148.9375000013656063, -2.891590998281053704 ) ) ;
#46148=VECTOR ( 'NONE', #62439, 1000.000000000000000 ) ;
#46150=ADVANCED_FACE ( 'NONE', ( #57002 ), #27394, .F. ) ;
#46159=CARTESIAN_POINT ( 'NONE',  ( -51.75738570946856498, -143.7500000000000284, 3.805975901505576964 ) ) ;
#46166=CARTESIAN_POINT ( 'NONE',  ( -59.44456063193725015, -151.8125000013656063, -0.3552334253322034230 ) ) ;
#46167=CARTESIAN_POINT ( 'NONE',  ( -59.29741812935640155, -142.6250000013656063, -2.196230717870135685 ) ) ;
#46204=CARTESIAN_POINT ( 'NONE',  ( -60.14911071818854538, -141.0625000000000284, 1.666127454062681368 ) ) ;
#46213=CARTESIAN_POINT ( 'NONE',  ( -52.80376928212989185, -143.1250000013656063, -4.297418129356378458 ) ) ;
#46215=CARTESIAN_POINT ( 'NONE',  ( -59.98410592259440222, -131.2500000027312126, -0.3983568153799752487 ) ) ;
#46227=CARTESIAN_POINT ( 'NONE',  ( -59.44456063193725015, -128.5625000013656063, -0.3552334253322034230 ) ) ;
#46233=CARTESIAN_POINT ( 'NONE',  ( -54.60164318462004474, -139.3750000000000284, -4.984105922594373794 ) ) ;
#46238=VECTOR ( 'NONE', #12562, 1000.000000000000114 ) ;
#46241=CARTESIAN_POINT ( 'NONE',  ( -58.39396692619412477, -134.4375000013656063, 2.891590998281057701 ) ) ;
#46253=CARTESIAN_POINT ( 'NONE',  ( -50.55543936806279248, -129.3125000013656063, 0.3552334253322060320 ) ) ;
#46280=CARTESIAN_POINT ( 'NONE',  ( -54.64476657466781973, -136.8125000013656063, -4.444560631937228834 ) ) ;
#46281=AXIS2_PLACEMENT_3D ( 'NONE', #360, #24161, #6700 ) ;
#46286=AXIS2_PLACEMENT_3D ( 'NONE', #51499, #37960, #17711 ) ;
#46287=CARTESIAN_POINT ( 'NONE',  ( -51.19402409849444524, -152.5000000000000284, -3.242614290531456334 ) ) ;
#46291=FILL_AREA_STYLE_COLOUR ( '', #59555 ) ;
#46298=CARTESIAN_POINT ( 'NONE',  ( -49.85088928181150436, -146.6875000027312126, -1.666127454062680702 ) ) ;
#46318=CARTESIAN_POINT ( 'NONE',  ( -53.51423613279429503, -144.2500000013656063, 4.591703134518082763 ) ) ;
#46351=DIRECTION ( 'NONE',  ( 0.000000000000000000, -1.000000000000000000, 0.000000000000000000 ) ) ;
#46363=CARTESIAN_POINT ( 'NONE',  ( -53.51423613279429503, -135.5000000013656063, 4.591703134518082763 ) ) ;
#46407=CARTESIAN_POINT ( 'NONE',  ( -57.89159099828107458, -139.9375000013656063, -3.393966926194107447 ) ) ;
#46415=DIRECTION ( 'NONE',  ( 0.000000000000000000, 1.000000000000000000, 0.000000000000000000 ) ) ;
#46427=CARTESIAN_POINT ( 'NONE',  ( -50.40829686548195099, -135.2500000013656347, -1.485763867205728284 ) ) ;
#46434=CARTESIAN_POINT ( 'NONE',  ( -58.24261429053147765, -139.2500000000000000, -3.805975901505573855 ) ) ;
#46441=CARTESIAN_POINT ( 'NONE',  ( -50.55543936806279248, -145.3125000013656063, 0.3552334253322060320 ) ) ;
#46446=ORIENTED_EDGE ( 'NONE', *, *, #518, .F. ) ;
#46448=CARTESIAN_POINT ( 'NONE',  ( -55.00000000000002132, -155.0000000000000284, 1.734723475976807094E-15 ) ) ;
#46453=CARTESIAN_POINT ( 'NONE',  ( -58.80597590150559739, -126.0000000000000284, 3.242614290531460330 ) ) ;
#46460=CARTESIAN_POINT ( 'NONE',  ( -57.19623071787017210, -150.3750000013656063, 4.297418129356382899 ) ) ;
#46483=CARTESIAN_POINT ( 'NONE',  ( -59.44456063193725015, -150.8125000013656063, -0.3552334253322034230 ) ) ;
#46485=EDGE_CURVE ( 'NONE', #24595, #12526, #4226, .T. ) ;
#46503=CARTESIAN_POINT ( 'NONE',  ( -58.24261429053147765, -152.2500000000000284, -3.805975901505573855 ) ) ;
#46511=VERTEX_POINT ( 'NONE', #63398 ) ;
#46527=CARTESIAN_POINT ( 'NONE',  ( -50.18089887299979068, -135.6875000000000000, 2.462841084822635640 ) ) ;
#46536=CARTESIAN_POINT ( 'NONE',  ( -51.60603307380591787, -143.1875000013656063, -2.891590998281053704 ) ) ;
#46538=CARTESIAN_POINT ( 'NONE',  ( -59.81910112700025905, -132.3125000027312126, -2.462841084822630311 ) ) ;
#46549=CARTESIAN_POINT ( 'NONE',  ( -57.46284108482265651, -153.9375000000000284, 4.819101127000238627 ) ) ;
#46550=CARTESIAN_POINT ( 'NONE',  ( -59.29741812935640155, -125.6250000013656205, -2.196230717870135685 ) ) ;
#46564=CARTESIAN_POINT ( 'NONE',  ( -55.35523342533222291, -132.3125000013656063, 4.444560631937231499 ) ) ;
#46574=CARTESIAN_POINT ( 'NONE',  ( -50.70258187064364108, -129.3750000013656347, 2.196230717870141014 ) ) ;
#46594=ORIENTED_EDGE ( 'NONE', *, *, #42428, .T. ) ;
#46595=CARTESIAN_POINT ( 'NONE',  ( -50.40829686548195099, -153.2500000013655779, -1.485763867205728284 ) ) ;
#46597=ORIENTED_EDGE ( 'NONE', *, *, #61399, .T. ) ;
#46599=CARTESIAN_POINT ( 'NONE',  ( -57.19623071787016499, -140.3750000013656063, 4.297418129356382899 ) ) ;
#46604=CARTESIAN_POINT ( 'NONE',  ( -60.14911071818854538, -149.0625000000000000, 1.666127454062681368 ) ) ;
#46613=CARTESIAN_POINT ( 'NONE',  ( -53.33387254593733928, -143.9375000027311842, 5.149110718188519620 ) ) ;
#46620=CARTESIAN_POINT ( 'NONE',  ( -58.39396692619412477, -136.4375000013655779, 2.891590998281057701 ) ) ;
#46635=CARTESIAN_POINT ( 'NONE',  ( -50.70258187064364108, -147.1250000013656063, 2.196230717870141014 ) ) ;
#46640=CARTESIAN_POINT ( 'NONE',  ( -52.53715891517739323, -141.5625000027312126, -4.819101127000233298 ) ) ;
#46662=AXIS2_PLACEMENT_3D ( 'NONE', #28331, #37991, #33474 ) ;
#46678=CARTESIAN_POINT ( 'NONE',  ( -52.10840900171896806, -132.4375000013656063, 3.393966926194110556 ) ) ;
#46693=CARTESIAN_POINT ( 'NONE',  ( -56.66612745406278151, -148.4375000027311842, -5.149110718188523173 ) ) ;
#46719=CARTESIAN_POINT ( 'NONE',  ( -58.39396692619412477, -139.6875000013656347, 2.891590998281057701 ) ) ;
#46738=EDGE_CURVE ( 'NONE', #58682, #26042, #29542, .T. ) ;
#46751=CARTESIAN_POINT ( 'NONE',  ( -50.70258187064364108, -147.3750000013656063, 2.196230717870141014 ) ) ;
#46764=CARTESIAN_POINT ( 'NONE',  ( -51.19402409849444524, -127.5000000000000284, -3.242614290531456334 ) ) ;
#46772=CARTESIAN_POINT ( 'NONE',  ( -55.35523342533222291, -149.3125000013656063, 4.444560631937231499 ) ) ;
#46797=CARTESIAN_POINT ( 'NONE',  ( -53.51423613279429503, -152.5000000013655779, 4.591703134518082763 ) ) ;
#46812=CARTESIAN_POINT ( 'NONE',  ( -51.75738570946856498, -135.7500000000000284, 3.805975901505576964 ) ) ;
#46835=CARTESIAN_POINT ( 'NONE',  ( -59.98410592259440222, -138.1250000000000284, -0.3983568153799752487 ) ) ;
#46847=CARTESIAN_POINT ( 'NONE',  ( -55.35523342533222291, -140.5625000013656063, 4.444560631937231499 ) ) ;
#46849=CARTESIAN_POINT ( 'NONE',  ( -55.39835681537999790, -130.0000000027312126, 4.984105922594378235 ) ) ;
#46853=CARTESIAN_POINT ( 'NONE',  ( -51.75738570946856498, -155.0000000000000284, 3.805975901505576520 ) ) ;
#46865=CARTESIAN_POINT ( 'NONE',  ( -59.59170313451811296, -125.5000000013656205, 1.485763867205729394 ) ) ;
#46871=ADVANCED_FACE ( 'NONE', ( #42113 ), #18308, .F. ) ;
#46879=CARTESIAN_POINT ( 'NONE',  ( -54.64476657466781973, -133.8125000013656063, -4.444560631937228834 ) ) ;
#46890=CARTESIAN_POINT ( 'NONE',  ( -52.10840900171896806, -129.4375000013656063, 3.393966926194110556 ) ) ;
#46918=CARTESIAN_POINT ( 'NONE',  ( -59.44456063193725015, -138.5625000013656063, -0.3552334253322034230 ) ) ;
#46923=CARTESIAN_POINT ( 'NONE',  ( -59.81910112700025905, -149.1875000000000000, -2.462841084822630311 ) ) ;
#46931=CARTESIAN_POINT ( 'NONE',  ( -51.60603307380591787, -153.1875000013656063, -2.891590998281053704 ) ) ;
#46932=CARTESIAN_POINT ( 'NONE',  ( -53.33387254593733928, -141.9375000027312126, 5.149110718188519620 ) ) ;
#46943=CARTESIAN_POINT ( 'NONE',  ( -50.70258187064364108, -138.1250000013656063, 2.196230717870141014 ) ) ;
#46959=CARTESIAN_POINT ( 'NONE',  ( -52.80376928212989185, -145.8750000013655779, -4.297418129356379346 ) ) ;
#46979=VERTEX_POINT ( 'NONE', #43374 ) ;
#47000=CARTESIAN_POINT ( 'NONE',  ( -54.64476657466781973, -133.0625000013656063, -4.444560631937228834 ) ) ;
#47016=CARTESIAN_POINT ( 'NONE',  ( -51.75738570946856498, -148.8750000027312126, 3.805975901505576964 ) ) ;
#47042=CARTESIAN_POINT ( 'NONE',  ( -52.80376928212989185, -136.1250000013656063, -4.297418129356379346 ) ) ;
#47075=CARTESIAN_POINT ( 'NONE',  ( -57.89159099828107458, -142.9375000013656063, -3.393966926194107447 ) ) ;
#47086=CARTESIAN_POINT ( 'NONE',  ( -58.24261429053147765, -126.2500000000000284, -3.805975901505573855 ) ) ;
#47093=CARTESIAN_POINT ( 'NONE',  ( -59.44456063193725015, -150.5625000013656063, -0.3552334253322034230 ) ) ;
#47118=CARTESIAN_POINT ( 'NONE',  ( -50.55543936806279248, -150.3125000013656063, 0.3552334253322060320 ) ) ;
#47129=CARTESIAN_POINT ( 'NONE',  ( -58.80597590150559739, -153.0000000000000284, 3.242614290531460330 ) ) ;
#47136=CARTESIAN_POINT ( 'NONE',  ( -50.18089887299979068, -152.6875000000000000, 2.462841084822605442 ) ) ;
#47158=CARTESIAN_POINT ( 'NONE',  ( -54.60164318462004474, -137.3750000000000284, -4.984105922594373794 ) ) ;
#47162=ORIENTED_EDGE ( 'NONE', *, *, #22427, .F. ) ;
#47169=CARTESIAN_POINT ( 'NONE',  ( -54.64476657466781973, -137.0625000013656063, -4.444560631937228834 ) ) ;
#47171=CARTESIAN_POINT ( 'NONE',  ( -59.81910112700025905, -129.3125000027312694, -2.462841084822630311 ) ) ;
#47183=CARTESIAN_POINT ( 'NONE',  ( -50.55543936806279248, -125.0625000013655921, 0.3552334253322060320 ) ) ;
#47195=CARTESIAN_POINT ( 'NONE',  ( -53.51423613279429503, -133.2500000013656347, 4.591703134518082763 ) ) ;
#47205=AXIS2_PLACEMENT_3D ( 'NONE', #7425, #31533, #11277 ) ;
#47206=CARTESIAN_POINT ( 'NONE',  ( -58.39396692619412477, -128.6875000013656063, 2.891590998281057701 ) ) ;
#47217=LINE ( 'NONE', #51095, #54211 ) ;
#47230=CARTESIAN_POINT ( 'NONE',  ( -50.70258187064364108, -154.3750000013656063, 2.196230717870141014 ) ) ;
#47235=CARTESIAN_POINT ( 'NONE',  ( -56.48576386720575471, -137.7500000013656063, -4.591703134518078322 ) ) ;
#47240=CARTESIAN_POINT ( 'NONE',  ( -56.66612745406270335, -151.3125000000000284, -5.149110718188516067 ) ) ;
#47249=CARTESIAN_POINT ( 'NONE',  ( -51.60603307380591787, -149.1875000013656063, -2.891590998281053704 ) ) ;
#47250=CARTESIAN_POINT ( 'NONE',  ( -52.53715891517739323, -144.5625000027311842, -4.819101127000233298 ) ) ;
#47252=CYLINDRICAL_SURFACE ( 'NONE', #35269, 5.000000000000000000 ) ;
#47258=CARTESIAN_POINT ( 'NONE',  ( -51.60603307380591787, -135.9375000013656063, -2.891590998281053704 ) ) ;
#47272=CARTESIAN_POINT ( 'NONE',  ( -53.51423613279429503, -145.2500000013656347, 4.591703134518082763 ) ) ;
#47303=EDGE_LOOP ( 'NONE', ( #55236, #55037, #23766, #163 ) ) ;
#47314=CARTESIAN_POINT ( 'NONE',  ( -57.19623071787017210, -130.6250000013656347, 4.297418129356382899 ) ) ;
#47356=CARTESIAN_POINT ( 'NONE',  ( -50.70258187064364108, -137.3750000013656063, 2.196230717870141014 ) ) ;
#47359=CARTESIAN_POINT ( 'NONE',  ( -52.53715891517739323, -145.4375000000000284, -4.819101127000233298 ) ) ;
#47378=CYLINDRICAL_SURFACE ( 'NONE', #60760, 5.000000000000000000 ) ;
#47387=CARTESIAN_POINT ( 'NONE',  ( -57.89159099828107458, -141.9375000013656063, -3.393966926194107447 ) ) ;
#47394=CARTESIAN_POINT ( 'NONE',  ( -58.24261429053147765, -155.0000000000000284, -3.805975901505573411 ) ) ;
#47403=CARTESIAN_POINT ( 'NONE',  ( -50.55543936806279248, -149.0625000013656063, 0.3552334253322060320 ) ) ;
#47407=EDGE_LOOP ( 'NONE', ( #62793, #7501, #6323, #49526 ) ) ;
#47416=CARTESIAN_POINT ( 'NONE',  ( -54.60164318462004474, -140.5000000027312126, -4.984105922594373794 ) ) ;
#47429=CARTESIAN_POINT ( 'NONE',  ( -58.39396692619412477, -147.6875000013656063, 2.891590998281057701 ) ) ;
#47463=CARTESIAN_POINT ( 'NONE',  ( -51.75738570946856498, -136.7500000000000284, 3.805975901505576964 ) ) ;
#47470=DIRECTION ( 'NONE',  ( -0.6485228581062915110, 0.000000000000000000, -0.7611951803011149931 ) ) ;
#47471=CARTESIAN_POINT ( 'NONE',  ( -57.89159099828107458, -139.9375000013656063, -3.393966926194107447 ) ) ;
#47473=CARTESIAN_POINT ( 'NONE',  ( -56.66612745406270335, -132.4375000027312410, -5.149110718188516067 ) ) ;
#47497=CARTESIAN_POINT ( 'NONE',  ( -52.10840900171896806, -130.1875000013656063, 3.393966926194110556 ) ) ;
#47510=CARTESIAN_POINT ( 'NONE',  ( -50.55543936806279248, -127.3125000013655921, 0.3552334253322060320 ) ) ;
#47537=CARTESIAN_POINT ( 'NONE',  ( -50.55543936806279248, -136.0625000013656063, 0.3552334253322060320 ) ) ;
#47542=CARTESIAN_POINT ( 'NONE',  ( -59.81910112700025905, -151.1875000000000000, -2.462841084822630311 ) ) ;
#47551=CARTESIAN_POINT ( 'NONE',  ( -51.60603307380591787, -151.1875000013656063, -2.891590998281053704 ) ) ;
#47552=CARTESIAN_POINT ( 'NONE',  ( -59.81910112700025905, -144.3125000027312126, -2.462841084822630311 ) ) ;
#47562=CARTESIAN_POINT ( 'NONE',  ( -57.19623071787017210, -135.3750000013656063, 4.297418129356382899 ) ) ;
#47576=CARTESIAN_POINT ( 'NONE',  ( -50.70258187064364108, -144.1250000013656063, 2.196230717870141014 ) ) ;
#47596=DIRECTION ( 'NONE',  ( 0.000000000000000000, 1.000000000000000000, 0.000000000000000000 ) ) ;
#47618=CARTESIAN_POINT ( 'NONE',  ( -50.40829686548195099, -129.2500000013656347, -1.485763867205728284 ) ) ;
#47625=CARTESIAN_POINT ( 'NONE',  ( -53.33387254593733928, -152.9375000027312126, 5.149110718188519620 ) ) ;
#47631=ADVANCED_FACE ( 'NONE', ( #22756 ), #21806, .F. ) ;
#47664=CARTESIAN_POINT ( 'NONE',  ( -59.29741812935640155, -137.8750000013655779, -2.196230717870135685 ) ) ;
#47694=CARTESIAN_POINT ( 'NONE',  ( -50.40829686548195099, -144.2500000013656063, -1.485763867205728284 ) ) ;
#47712=CARTESIAN_POINT ( 'NONE',  ( -58.39396692619412477, -143.4375000013656063, 2.891590998281057701 ) ) ;
#47721=CARTESIAN_POINT ( 'NONE',  ( -58.24261429053147765, -142.2500000000000284, -3.805975901505573855 ) ) ;
#47723=CARTESIAN_POINT ( 'NONE',  ( -52.53715891517739323, -140.5625000027311842, -4.819101127000233298 ) ) ;
#47726=CARTESIAN_POINT ( 'NONE',  ( -51.19402409849444524, -139.5000000000000284, -3.242614290531456334 ) ) ;
#47737=CARTESIAN_POINT ( 'NONE',  ( -59.29741812935640155, -147.8750000013656063, -2.196230717870135685 ) ) ;
#47744=CARTESIAN_POINT ( 'NONE',  ( -60.14911071818854538, -148.0625000000000000, 1.666127454062681146 ) ) ;
#47774=CARTESIAN_POINT ( 'NONE',  ( -49.85088928181150436, -132.5625000000000568, -1.666127454062680702 ) ) ;
#47781=CARTESIAN_POINT ( 'NONE',  ( -51.60603307380591787, -138.1875000013656347, -2.891590998281053704 ) ) ;
#47783=CARTESIAN_POINT ( 'NONE',  ( -51.19402409849444524, -127.6250000027312268, -3.242614290531456334 ) ) ;
#47791=CYLINDRICAL_SURFACE ( 'NONE', #45358, 5.000000000000000000 ) ;
#47795=CARTESIAN_POINT ( 'NONE',  ( -57.89159099828107458, -124.6875000013656063, -3.393966926194107447 ) ) ;
#47806=CARTESIAN_POINT ( 'NONE',  ( -58.39396692619412477, -128.4375000013656063, 2.891590998281057701 ) ) ;
#47814=VERTEX_POINT ( 'NONE', #58724 ) ;
#47816=CARTESIAN_POINT ( 'NONE',  ( -50.55543936806279248, -125.3125000013655921, 0.3552334253322060320 ) ) ;
#47828=CARTESIAN_POINT ( 'NONE',  ( -51.75738570946856498, -135.7500000000000284, 3.805975901505576964 ) ) ;
#47838=ORIENTED_EDGE ( 'NONE', *, *, #54323, .F. ) ;
#47839=CARTESIAN_POINT ( 'NONE',  ( -52.80376928212989185, -153.1250000013656063, -4.297418129356379346 ) ) ;
#47843=CARTESIAN_POINT ( 'NONE',  ( -53.51423613279429503, -136.2500000013656063, 4.591703134518083651 ) ) ;
#47848=CARTESIAN_POINT ( 'NONE',  ( -50.01589407740564042, -148.6250000000000284, 0.3983568153799778022 ) ) ;
#47858=CARTESIAN_POINT ( 'NONE',  ( -50.70258187064364108, -149.3750000013656063, 2.196230717870141014 ) ) ;
#47859=CARTESIAN_POINT ( 'NONE',  ( -49.85088928181150436, -142.6875000027312126, -1.666127454062680702 ) ) ;
#47867=CARTESIAN_POINT ( 'NONE',  ( -57.89159099828107458, -135.6875000013656063, -3.393966926194107447 ) ) ;
#47884=CARTESIAN_POINT ( 'NONE',  ( -59.29741812935640155, -140.6250000013656063, -2.196230717870135685 ) ) ;
#47888=CARTESIAN_POINT ( 'NONE',  ( -58.24261429053147765, -144.2500000000000284, -3.805975901505573855 ) ) ;
#47927=CARTESIAN_POINT ( 'NONE',  ( -50.55543936806279248, -130.3125000013656063, 0.3552334253322060320 ) ) ;
#47954=LINE ( 'NONE', #62767, #44187 ) ;
#47958=CARTESIAN_POINT ( 'NONE',  ( -50.70258187064364108, -153.1250000013656063, 2.196230717870141014 ) ) ;
#47974=CARTESIAN_POINT ( 'NONE',  ( -50.55543936806279248, -137.3125000013656063, 0.3552334253322060320 ) ) ;
#48006=CARTESIAN_POINT ( 'NONE',  ( -58.39396692619412477, -143.6875000013656063, 2.891590998281057701 ) ) ;
#48012=ORIENTED_EDGE ( 'NONE', *, *, #51599, .F. ) ;
#48024=VECTOR ( 'NONE', #4325, 1000.000000000000114 ) ;
#48027=CARTESIAN_POINT ( 'NONE',  ( -59.44456063193725015, -146.5625000013656063, -0.3552334253322034230 ) ) ;
#48030=ORIENTED_EDGE ( 'NONE', *, *, #23605, .T. ) ;
#48037=CARTESIAN_POINT ( 'NONE',  ( -58.80597590150559739, -142.0000000000000284, 3.242614290531460330 ) ) ;
#48050=CARTESIAN_POINT ( 'NONE',  ( -58.39396692619412477, -148.6875000013656063, 2.891590998281057701 ) ) ;
#48058=CARTESIAN_POINT ( 'NONE',  ( -55.39835681537999790, -138.0000000027312126, 4.984105922594378235 ) ) ;
#48075=CARTESIAN_POINT ( 'NONE',  ( -50.18089887299981200, -135.6875000000000000, 2.462841084822874116 ) ) ;
#48089=CARTESIAN_POINT ( 'NONE',  ( -59.81910112700025905, -133.1875000000000284, -2.462841084822630311 ) ) ;
#48092=EDGE_CURVE ( 'NONE', #19422, #6296, #24559, .T. ) ;
#48097=ORIENTED_EDGE ( 'NONE', *, *, #12660, .F. ) ;
#48098=CARTESIAN_POINT ( 'NONE',  ( -50.55543936806279248, -138.3125000013656063, 0.3552334253322060320 ) ) ;
#48100=CARTESIAN_POINT ( 'NONE',  ( -50.01589407740564042, -127.7500000027312126, 0.3983568153799778022 ) ) ;
#48110=CARTESIAN_POINT ( 'NONE',  ( -58.24261429053147765, -155.0000000000000284, -3.805975901505573411 ) ) ;
#48126=CARTESIAN_POINT ( 'NONE',  ( -59.59170313451811296, -130.5000000013656063, 1.485763867205729394 ) ) ;
#48127=CARTESIAN_POINT ( 'NONE',  ( -50.40829686548195099, -148.0000000013656063, -1.485763867205728284 ) ) ;
#48138=LINE ( 'NONE', #13419, #53431 ) ;
#48145=CARTESIAN_POINT ( 'NONE',  ( -50.01589407740564042, -137.7500000027312126, 0.3983568153799778022 ) ) ;
#48160=CARTESIAN_POINT ( 'NONE',  ( -50.40829686548195099, -149.2500000013655779, -1.485763867205728284 ) ) ;
#48164=CARTESIAN_POINT ( 'NONE',  ( -50.40829686548195099, -136.0000000013656063, -1.485763867205728284 ) ) ;
#48169=CARTESIAN_POINT ( 'NONE',  ( -53.33387254593733928, -144.8125000000000284, 5.149110718188519620 ) ) ;
#48179=CARTESIAN_POINT ( 'NONE',  ( -59.59170313451810586, -149.7500000013656063, 1.485763867205729394 ) ) ;
#48180=CARTESIAN_POINT ( 'NONE',  ( -54.60164318462004474, -140.5000000027312126, -4.984105922594373794 ) ) ;
#48188=CARTESIAN_POINT ( 'NONE',  ( -59.59170313451811296, -133.5000000013656347, 1.485763867205729394 ) ) ;
#48204=CARTESIAN_POINT ( 'NONE',  ( -51.60603307380591787, -140.9375000013656063, -2.891590998281053704 ) ) ;
#48233=CYLINDRICAL_SURFACE ( 'NONE', #59736, 5.000000000000000000 ) ;
#48242=CARTESIAN_POINT ( 'NONE',  ( -56.48576386720575471, -127.0000000013656063, -4.591703134518078322 ) ) ;
#48251=CARTESIAN_POINT ( 'NONE',  ( -52.53715891517739323, -150.5625000027311842, -4.819101127000233298 ) ) ;
#48255=CARTESIAN_POINT ( 'NONE',  ( -62.00000000000001421, -155.0000000000000284, -4.041451884327373456 ) ) ;
#48265=CARTESIAN_POINT ( 'NONE',  ( -58.80597590150559739, -154.1250000027312126, 3.242614290531460330 ) ) ;
#48270=LINE ( 'NONE', #48586, #697 ) ;
#48285=CARTESIAN_POINT ( 'NONE',  ( -51.60603307380591787, -134.1875000013656063, -2.891590998281053704 ) ) ;
#48318=CARTESIAN_POINT ( 'NONE',  ( -59.29741812935640155, -143.8750000013655779, -2.196230717870135685 ) ) ;
#48322=EDGE_CURVE ( 'NONE', #40253, #7528, #19783, .T. ) ;
#48328=ORIENTED_EDGE ( 'NONE', *, *, #20950, .T. ) ;
#48338=CARTESIAN_POINT ( 'NONE',  ( -53.51423613279429503, -145.2500000013656347, 4.591703134518082763 ) ) ;
#48349=EDGE_CURVE ( 'NONE', #27617, #4086, #2914, .T. ) ;
#48359=CARTESIAN_POINT ( 'NONE',  ( -59.81910112700027327, -140.3125000027311842, -2.462841084822392279 ) ) ;
#48366=CARTESIAN_POINT ( 'NONE',  ( -50.55543936806279248, -147.3125000013656063, 0.3552334253322060320 ) ) ;
#48402=CARTESIAN_POINT ( 'NONE',  ( -55.39835681537999790, -131.8750000000000284, 4.984105922594378235 ) ) ;
#48405=ORIENTED_EDGE ( 'NONE', *, *, #26298, .F. ) ;
#48411=CARTESIAN_POINT ( 'NONE',  ( -58.80597590150559739, -128.1250000027312126, 3.242614290531460330 ) ) ;
#48413=CARTESIAN_POINT ( 'NONE',  ( -52.47078701390809385, -134.9999999999999716, 4.127771267674353872 ) ) ;
#48416=CARTESIAN_POINT ( 'NONE',  ( -57.46284108482265651, -145.9375000000000284, 4.819101127000238627 ) ) ;
#48421=DIRECTION ( 'NONE',  ( -0.6485228581062915110, 0.000000000000000000, -0.7611951803011149931 ) ) ;
#48440=CARTESIAN_POINT ( 'NONE',  ( -59.29741812935640155, -129.6250000013655779, -2.196230717870135685 ) ) ;
#48441=CARTESIAN_POINT ( 'NONE',  ( -59.44456063193725015, -147.5625000013656063, -0.3552334253322034230 ) ) ;
#48468=CARTESIAN_POINT ( 'NONE',  ( -54.60164318462004474, -144.5000000027312126, -4.984105922594373794 ) ) ;
#48469=CARTESIAN_POINT ( 'NONE',  ( -58.24261429053147765, -155.0000000000000284, -3.805975901505573411 ) ) ;
#48475=CARTESIAN_POINT ( 'NONE',  ( -57.89159099828107458, -150.9375000013656063, -3.393966926194107447 ) ) ;
#48485=CARTESIAN_POINT ( 'NONE',  ( -49.85088928181150436, -146.5625000000000284, -1.666127454062680702 ) ) ;
#48494=CARTESIAN_POINT ( 'NONE',  ( -50.40829686548195099, -151.2500000013656063, -1.485763867205728284 ) ) ;
#48495=CARTESIAN_POINT ( 'NONE',  ( -56.66612745406270335, -139.4375000027312410, -5.149110718188516067 ) ) ;
#48503=CARTESIAN_POINT ( 'NONE',  ( -50.70258187064364108, -131.1250000013655779, 2.196230717870141014 ) ) ;
#48505=DIRECTION ( 'NONE',  ( -0.6485228581062915110, 0.000000000000000000, -0.7611951803011149931 ) ) ;
#48518=CARTESIAN_POINT ( 'NONE',  ( -50.55543936806279248, -141.0625000013656063, 0.3552334253322060320 ) ) ;
#48540=DIRECTION ( 'NONE',  ( 0.000000000000000000, 1.000000000000000000, 0.000000000000000000 ) ) ;
#48551=CARTESIAN_POINT ( 'NONE',  ( -54.64476657466781973, -152.8125000013656063, -4.444560631937228834 ) ) ;
#48558=CARTESIAN_POINT ( 'NONE',  ( -50.55543936806279248, -125.3125000013655921, 0.3552334253322060320 ) ) ;
#48569=CARTESIAN_POINT ( 'NONE',  ( -51.75738570946856498, -151.8750000027312126, 3.805975901505576964 ) ) ;
#48586=CARTESIAN_POINT ( 'NONE',  ( -62.00000000000001421, -135.0000000000000284, -4.041451884327373456 ) ) ;
#48588=CARTESIAN_POINT ( 'NONE',  ( -51.75738570946856498, -147.8750000027312126, 3.805975901505576964 ) ) ;
#48601=CARTESIAN_POINT ( 'NONE',  ( -54.64476657466781973, -132.0625000013656063, -4.444560631937228834 ) ) ;
#48603=DIRECTION ( 'NONE',  ( 0.000000000000000000, 1.000000000000000000, 0.000000000000000000 ) ) ;
#48604=CARTESIAN_POINT ( 'NONE',  ( -51.75738570946856498, -152.8750000027312126, 3.805975901505576964 ) ) ;
#48622=CARTESIAN_POINT ( 'NONE',  ( -50.18089887299980489, -136.6875000000000568, 2.462841084822814164 ) ) ;
#48631=CARTESIAN_POINT ( 'NONE',  ( -52.10840900171896806, -139.4375000013656063, 3.393966926194110556 ) ) ;
#48634=ORIENTED_EDGE ( 'NONE', *, *, #10669, .T. ) ;
#48636=ORIENTED_EDGE ( 'NONE', *, *, #51902, .T. ) ;
#48648=CARTESIAN_POINT ( 'NONE',  ( -54.64476657466781973, -146.8125000013656063, -4.444560631937228834 ) ) ;
#48667=CARTESIAN_POINT ( 'NONE',  ( -53.33387254593710480, -139.9375000027311557, 5.149110718188539160 ) ) ;
#48670=CARTESIAN_POINT ( 'NONE',  ( -52.53715891517739323, -154.4375000000000000, -4.819101127000233298 ) ) ;
#48673=CARTESIAN_POINT ( 'NONE',  ( -52.80376928212989185, -147.1250000013656063, -4.297418129356379346 ) ) ;
#48692=LINE ( 'NONE', #15243, #53389 ) ;
#48714=CARTESIAN_POINT ( 'NONE',  ( -58.80597590150559739, -134.0000000000000284, 3.242614290531460330 ) ) ;
#48723=CARTESIAN_POINT ( 'NONE',  ( -55.39835681537999790, -126.0000000027311984, 4.984105922594378235 ) ) ;
#48724=CARTESIAN_POINT ( 'NONE',  ( -53.31921341345466203, -135.0000000000000000, 4.586462452526608224 ) ) ;
#48745=CARTESIAN_POINT ( 'NONE',  ( -59.59170313451811296, -128.5000000013656063, 1.485763867205729394 ) ) ;
#48746=CARTESIAN_POINT ( 'NONE',  ( -54.64476657466781973, -144.8125000013656063, -4.444560631937228834 ) ) ;
#48781=CARTESIAN_POINT ( 'NONE',  ( -57.19623071787017210, -152.6250000013656063, 4.297418129356382899 ) ) ;
#48792=CARTESIAN_POINT ( 'NONE',  ( -60.14911071818854538, -147.0625000000000000, 1.666127454062681368 ) ) ;
#48800=CARTESIAN_POINT ( 'NONE',  ( -58.24261429053147765, -135.3750000027312410, -3.805975901505573855 ) ) ;
#48803=CARTESIAN_POINT ( 'NONE',  ( -57.89159099828107458, -146.9375000013656063, -3.393966926194107447 ) ) ;
#48804=CARTESIAN_POINT ( 'NONE',  ( -58.24261429053147765, -140.3750000027312126, -3.805975901505573855 ) ) ;
#48814=CARTESIAN_POINT ( 'NONE',  ( -50.01589407740564042, -153.6250000000000284, 0.3983568153799778022 ) ) ;
#48815=CARTESIAN_POINT ( 'NONE',  ( -52.10840900171896806, -133.1875000013656063, 3.393966926194110556 ) ) ;
#48830=CARTESIAN_POINT ( 'NONE',  ( -54.64476657466781973, -141.8125000013656063, -4.444560631937228834 ) ) ;
#48861=ORIENTED_EDGE ( 'NONE', *, *, #33924, .T. ) ;
#48862=CARTESIAN_POINT ( 'NONE',  ( -59.29741812935640155, -151.6250000013655779, -2.196230717870135685 ) ) ;
#48866=CARTESIAN_POINT ( 'NONE',  ( -50.18089887299978358, -149.8125000027312126, 2.462841084822575688 ) ) ;
#48869=CARTESIAN_POINT ( 'NONE',  ( -59.29741812935640155, -126.8750000013656205, -2.196230717870135685 ) ) ;
#48878=DIRECTION ( 'NONE',  ( 0.000000000000000000, 1.000000000000000000, 0.000000000000000000 ) ) ;
#48880=CARTESIAN_POINT ( 'NONE',  ( -53.33387254593733928, -148.9375000027311842, 5.149110718188519620 ) ) ;
#48936=CARTESIAN_POINT ( 'NONE',  ( -54.60164318462004474, -136.3750000000000284, -4.984105922594373794 ) ) ;
#48944=CARTESIAN_POINT ( 'NONE',  ( -50.70258187064364108, -140.3750000013656063, 2.196230717870141014 ) ) ;
#48961=CARTESIAN_POINT ( 'NONE',  ( -59.29741812935640155, -143.6250000013655779, -2.196230717870135685 ) ) ;
#48976=CARTESIAN_POINT ( 'NONE',  ( -56.66612745406288099, -142.4375000027312126, -5.149110718188529390 ) ) ;
#48990=CARTESIAN_POINT ( 'NONE',  ( -51.60603307380591787, -142.1875000013656063, -2.891590998281053704 ) ) ;
#48995=CARTESIAN_POINT ( 'NONE',  ( -59.98410592259440222, -148.1250000000000284, -0.3983568153799752487 ) ) ;
#49009=CARTESIAN_POINT ( 'NONE',  ( -54.60164318462004474, -145.5000000027312126, -4.984105922594373794 ) ) ;
#49031=CARTESIAN_POINT ( 'NONE',  ( -51.19402409849444524, -134.5000000000000284, -3.242614290531456334 ) ) ;
#49039=CARTESIAN_POINT ( 'NONE',  ( -51.75738570946856498, -125.8750000027312126, 3.805975901505576964 ) ) ;
#49065=CARTESIAN_POINT ( 'NONE',  ( -57.19623071787017210, -127.3750000013656205, 4.297418129356382899 ) ) ;
#49066=CARTESIAN_POINT ( 'NONE',  ( -56.48576386720575471, -146.7500000013656063, -4.591703134518078322 ) ) ;
#49077=CARTESIAN_POINT ( 'NONE',  ( -54.64476657466781973, -125.0625000013655921, -4.444560631937228834 ) ) ;
#49101=CARTESIAN_POINT ( 'NONE',  ( -58.39396692619412477, -150.6875000013656063, 2.891590998281057701 ) ) ;
#49112=CARTESIAN_POINT ( 'NONE',  ( -59.81910112700025905, -144.1875000000000000, -2.462841084822630311 ) ) ;
#49122=CARTESIAN_POINT ( 'NONE',  ( -57.19623071787016499, -146.6250000013656063, 4.297418129356382899 ) ) ;
#49123=CARTESIAN_POINT ( 'NONE',  ( -54.60164318462004474, -138.5000000027312126, -4.984105922594373794 ) ) ;
#49135=CARTESIAN_POINT ( 'NONE',  ( -50.40829686548195099, -133.0000000013656063, -1.485763867205728284 ) ) ;
#49137=CARTESIAN_POINT ( 'NONE',  ( -58.80597590150559739, -146.1250000027312126, 3.242614290531460330 ) ) ;
#49138=CARTESIAN_POINT ( 'NONE',  ( -56.66612745406283125, -146.4375000027312694, -5.149110718188525837 ) ) ;
#49150=CARTESIAN_POINT ( 'NONE',  ( -50.40829686548195099, -140.0000000013656063, -1.485763867205728284 ) ) ;
#49167=DIRECTION ( 'NONE',  ( 0.000000000000000000, 1.000000000000000000, 0.000000000000000000 ) ) ;
#49190=CARTESIAN_POINT ( 'NONE',  ( -58.39396692619412477, -153.4375000013656063, 2.891590998281057701 ) ) ;
#49197=CARTESIAN_POINT ( 'NONE',  ( -53.51423613279429503, -128.5000000013656063, 4.591703134518082763 ) ) ;
#49207=CARTESIAN_POINT ( 'NONE',  ( -50.01589407740564042, -148.7500000027312126, 0.3983568153799778022 ) ) ;
#49225=CARTESIAN_POINT ( 'NONE',  ( -58.39396692619412477, -154.5625000013656063, 2.891590998281057701 ) ) ;
#49226=CARTESIAN_POINT ( 'NONE',  ( -53.51423613279429503, -154.2500000013656063, 4.591703134518082763 ) ) ;
#49259=VECTOR ( 'NONE', #34856, 1000.000000000000000 ) ;
#49277=CARTESIAN_POINT ( 'NONE',  ( -52.10840900171896806, -140.4375000013656063, 3.393966926194110556 ) ) ;
#49294=CARTESIAN_POINT ( 'NONE',  ( -55.35523342533222291, -139.3125000013656063, 4.444560631937231499 ) ) ;
#49317=CARTESIAN_POINT ( 'NONE',  ( -57.19623071787017210, -143.6250000013655779, 4.297418129356382899 ) ) ;
#49356=CARTESIAN_POINT ( 'NONE',  ( -51.19402409849444524, -130.5000000000000284, -3.242614290531456334 ) ) ;
#49366=CARTESIAN_POINT ( 'NONE',  ( -57.19623071787017210, -152.3750000013656063, 4.297418129356382899 ) ) ;
#49392=CARTESIAN_POINT ( 'NONE',  ( -57.19623071787017210, -125.3750000013656205, 4.297418129356382899 ) ) ;
#49393=CARTESIAN_POINT ( 'NONE',  ( -52.80376928212989185, -147.8750000013655779, -4.297418129356378458 ) ) ;
#49423=CARTESIAN_POINT ( 'NONE',  ( -50.70258187064364108, -148.3750000013656063, 2.196230717870141014 ) ) ;
#49434=CARTESIAN_POINT ( 'NONE',  ( -55.39835681537999790, -143.8750000000000284, 4.984105922594378235 ) ) ;
#49444=CARTESIAN_POINT ( 'NONE',  ( -57.89159099828107458, -147.9375000013656063, -3.393966926194107447 ) ) ;
#49446=CARTESIAN_POINT ( 'NONE',  ( -60.14911071818854538, -136.1875000027312126, 1.666127454062681368 ) ) ;
#49453=VERTEX_POINT ( 'NONE', #18993 ) ;
#49455=CARTESIAN_POINT ( 'NONE',  ( -58.24261429053147765, -143.3750000027312126, -3.805975901505573855 ) ) ;
#49460=CARTESIAN_POINT ( 'NONE',  ( -54.64476657466781973, -134.8125000013656063, -4.444560631937228834 ) ) ;
#49462=CARTESIAN_POINT ( 'NONE',  ( -51.19402409849444524, -146.6250000027312126, -3.242614290531456334 ) ) ;
#49467=CARTESIAN_POINT ( 'NONE',  ( -55.00000000000002132, -155.0000000000000284, 1.734723475976807094E-15 ) ) ;
#49475=EDGE_CURVE ( 'NONE', #36935, #59502, #4840, .T. ) ;
#49476=CARTESIAN_POINT ( 'NONE',  ( -50.40829686548195099, -136.0000000013656063, -1.485763867205728284 ) ) ;
#49506=CARTESIAN_POINT ( 'NONE',  ( -52.80376928212989185, -148.8750000013656063, -4.297418129356378458 ) ) ;
#49513=CARTESIAN_POINT ( 'NONE',  ( -56.48576386720575471, -128.0000000013656063, -4.591703134518078322 ) ) ;
#49524=CARTESIAN_POINT ( 'NONE',  ( -58.80597590150559739, -152.1250000027312126, 3.242614290531460330 ) ) ;
#49526=ORIENTED_EDGE ( 'NONE', *, *, #21949, .T. ) ;
#49544=CARTESIAN_POINT ( 'NONE',  ( -59.59170313451811296, -151.5000000013655779, 1.485763867205729394 ) ) ;
#49548=DIRECTION ( 'NONE',  ( -0.6485228581062915110, 0.000000000000000000, -0.7611951803011149931 ) ) ;
#49588=CARTESIAN_POINT ( 'NONE',  ( -51.60603307380591787, -140.1875000013656063, -2.891590998281053704 ) ) ;
#49591=EDGE_CURVE ( 'NONE', #44139, #13129, #63083, .T. ) ;
#49592=VERTEX_POINT ( 'NONE', #53413 ) ;
#49611=CARTESIAN_POINT ( 'NONE',  ( -58.39396692619412477, -142.4375000013656063, 2.891590998281057701 ) ) ;
#49615=CARTESIAN_POINT ( 'NONE',  ( -55.00000000000002132, -155.0000000000000284, 1.734723475976807094E-15 ) ) ;
#49638=CARTESIAN_POINT ( 'NONE',  ( -50.70258187064364108, -145.3750000013656347, 2.196230717870141014 ) ) ;
#49651=SHAPE_REPRESENTATION ( 'coupler', ( #43054 ), #60569 ) ;
#49677=CARTESIAN_POINT ( 'NONE',  ( -59.98410592259440222, -131.1250000000000284, -0.3983568153799752487 ) ) ;
#49685=CARTESIAN_POINT ( 'NONE',  ( -59.81910112700025905, -124.3125000027312268, -2.462841084822630311 ) ) ;
#49689=CARTESIAN_POINT ( 'NONE',  ( -59.98410592259440222, -146.1250000000000284, -0.3983568153799752487 ) ) ;
#49695=CARTESIAN_POINT ( 'NONE',  ( -59.98410592259440222, -145.1250000000000284, -0.3983568153799752487 ) ) ;
#49700=VERTEX_POINT ( 'NONE', #17043 ) ;
#49709=CARTESIAN_POINT ( 'NONE',  ( -59.59170313451811296, -125.5000000013656205, 1.485763867205729394 ) ) ;
#49710=CARTESIAN_POINT ( 'NONE',  ( -56.48576386720575471, -144.7500000013655779, -4.591703134518078322 ) ) ;
#49736=ORIENTED_EDGE ( 'NONE', *, *, #518, .T. ) ;
#49751=CARTESIAN_POINT ( 'NONE',  ( -58.24261429053147765, -142.2500000000000284, -3.805975901505573855 ) ) ;
#49759=CARTESIAN_POINT ( 'NONE',  ( -50.40829686548195099, -145.2500000013656347, -1.485763867205728284 ) ) ;
#49761=CARTESIAN_POINT ( 'NONE',  ( -51.19402409849444524, -136.6250000027312410, -3.242614290531456334 ) ) ;
#49764=DIRECTION ( 'NONE',  ( 0.000000000000000000, 1.000000000000000000, 0.000000000000000000 ) ) ;
#49773=CARTESIAN_POINT ( 'NONE',  ( -57.89159099828107458, -129.6875000013656063, -3.393966926194107447 ) ) ;
#49779=ORIENTED_EDGE ( 'NONE', *, *, #62174, .T. ) ;
#49781=CARTESIAN_POINT ( 'NONE',  ( -58.24261429053147765, -155.0000000000000284, -3.805975901505573411 ) ) ;
#49788=CARTESIAN_POINT ( 'NONE',  ( -56.48576386720575471, -135.7500000013656063, -4.591703134518078322 ) ) ;
#49797=CARTESIAN_POINT ( 'NONE',  ( -50.55543936806279248, -130.3125000013656063, 0.3552334253322060320 ) ) ;
#49821=CARTESIAN_POINT ( 'NONE',  ( -52.10840900171896806, -150.1875000013656063, 3.393966926194110556 ) ) ;
#49828=CARTESIAN_POINT ( 'NONE',  ( -57.46284108482265651, -154.9375000000000000, 4.819101127000239515 ) ) ;
#49838=CARTESIAN_POINT ( 'NONE',  ( -53.33387254593733928, -147.9375000027312126, 5.149110718188519620 ) ) ;
#49855=CARTESIAN_POINT ( 'NONE',  ( -51.60603307380591787, -147.9375000013656063, -2.891590998281053704 ) ) ;
#49860=FACE_OUTER_BOUND ( 'NONE', #39144, .T. ) ;
#49874=CARTESIAN_POINT ( 'NONE',  ( -54.60164318462004474, -151.5000000027312410, -4.984105922594373794 ) ) ;
#49879=CARTESIAN_POINT ( 'NONE',  ( -56.37266686252615955, -135.0000000000000284, -4.242180533871957593 ) ) ;
#49902=CARTESIAN_POINT ( 'NONE',  ( -52.10840900171896806, -137.4375000013656063, 3.393966926194110556 ) ) ;
#49921=CARTESIAN_POINT ( 'NONE',  ( -58.39396692619412477, -141.4375000013656063, 2.891590998281057701 ) ) ;
#49950=CARTESIAN_POINT ( 'NONE',  ( -57.89159099828107458, -143.9375000013656063, -3.393966926194107447 ) ) ;
#49951=FACE_OUTER_BOUND ( 'NONE', #42733, .T. ) ;
#49960=CYLINDRICAL_SURFACE ( 'NONE', #23338, 5.000000000000000000 ) ;
#49970=CYLINDRICAL_SURFACE ( 'NONE', #26729, 5.000000000000000000 ) ;
#49974=CARTESIAN_POINT ( 'NONE',  ( -58.24261429053147765, -139.3750000027312126, -3.805975901505573855 ) ) ;
#49986=CARTESIAN_POINT ( 'NONE',  ( -53.33387254593725402, -148.9375000027311842, 5.149110718188524949 ) ) ;
#49992=CARTESIAN_POINT ( 'NONE',  ( -54.60164318462004474, -130.3750000000000284, -4.984105922594373794 ) ) ;
#49995=AXIS2_PLACEMENT_3D ( 'NONE', #8844, #63510, #58991 ) ;
#50001=CARTESIAN_POINT ( 'NONE',  ( -54.64476657466781973, -152.8125000013656063, -4.444560631937228834 ) ) ;
#50027=CARTESIAN_POINT ( 'NONE',  ( -57.89159099828107458, -127.6875000013656063, -3.393966926194107447 ) ) ;
#50028=CARTESIAN_POINT ( 'NONE',  ( -58.39396692619412477, -142.4375000013656063, 2.891590998281057701 ) ) ;
#50071=CARTESIAN_POINT ( 'NONE',  ( -59.81910112700025905, -143.1875000000000000, -2.462841084822630311 ) ) ;
#50079=CARTESIAN_POINT ( 'NONE',  ( -52.10840900171896806, -146.4375000013656063, 3.393966926194110556 ) ) ;
#50081=CARTESIAN_POINT ( 'NONE',  ( -57.46284108482265651, -133.0625000027312410, 4.819101127000239515 ) ) ;
#50096=CARTESIAN_POINT ( 'NONE',  ( -50.55543936806279248, -128.0625000013656063, 0.3552334253322060320 ) ) ;
#50108=CARTESIAN_POINT ( 'NONE',  ( -59.44456063193725015, -139.5625000013656063, -0.3552334253322034230 ) ) ;
#50117=CARTESIAN_POINT ( 'NONE',  ( -59.29741812935640155, -131.8750000013656347, -2.196230717870135685 ) ) ;
#50126=CARTESIAN_POINT ( 'NONE',  ( -58.24261429053147765, -151.2500000000000284, -3.805975901505573855 ) ) ;
#50142=CARTESIAN_POINT ( 'NONE',  ( -57.19623071787016499, -149.3750000013656063, 4.297418129356382899 ) ) ;
#50149=CARTESIAN_POINT ( 'NONE',  ( -51.75738570946856498, -153.7500000000000284, 3.805975901505576964 ) ) ;
#50159=CARTESIAN_POINT ( 'NONE',  ( -50.01589407740564042, -146.7500000027312126, 0.3983568153799778022 ) ) ;
#50179=CARTESIAN_POINT ( 'NONE',  ( -58.24261429053147765, -145.2500000000000284, -3.805975901505573855 ) ) ;
#50180=CARTESIAN_POINT ( 'NONE',  ( -55.35523342533222291, -149.3125000013656063, 4.444560631937231499 ) ) ;
#50212=CARTESIAN_POINT ( 'NONE',  ( -51.75738570946856498, -147.8750000027312126, 3.805975901505576964 ) ) ;
#50229=AXIS2_PLACEMENT_3D ( 'NONE', #46448, #2394, #61249 ) ;
#50230=CARTESIAN_POINT ( 'NONE',  ( -56.48576386720575471, -137.0000000013655779, -4.591703134518078322 ) ) ;
#50237=ORIENTED_EDGE ( 'NONE', *, *, #24837, .F. ) ;
#50241=ADVANCED_FACE ( 'NONE', ( #45914 ), #25666, .F. ) ;
#50247=CARTESIAN_POINT ( 'NONE',  ( -50.40829686548195099, -140.0000000013656063, -1.485763867205728284 ) ) ;
#50248=CARTESIAN_POINT ( 'NONE',  ( -55.39835681537999790, -154.8750000000000284, 4.984105922594378235 ) ) ;
#50276=CARTESIAN_POINT ( 'NONE',  ( -50.70258187064364108, -142.3750000013656063, 2.196230717870141014 ) ) ;
#50317=CARTESIAN_POINT ( 'NONE',  ( -57.46284108482265651, -130.9375000000000000, 4.819101127000239515 ) ) ;
#50329=CARTESIAN_POINT ( 'NONE',  ( -53.51423613279429503, -151.2500000013656063, 4.591703134518082763 ) ) ;
#50353=CARTESIAN_POINT ( 'NONE',  ( -59.29741812935640155, -125.6250000013656205, -2.196230717870135685 ) ) ;
#50354=CARTESIAN_POINT ( 'NONE',  ( -57.89159099828107458, -141.6875000013656063, -3.393966926194107447 ) ) ;
#50357=CARTESIAN_POINT ( 'NONE',  ( -56.66612745406272467, -153.4375000027312126, -5.149110718188517843 ) ) ;
#50384=ORIENTED_EDGE ( 'NONE', *, *, #1467, .F. ) ;
#50392=CARTESIAN_POINT ( 'NONE',  ( -58.24261429053147765, -143.2500000000000284, -3.805975901505573855 ) ) ;
#50397=EDGE_CURVE ( 'NONE', #7528, #27617, #41953, .T. ) ;
#50404=CARTESIAN_POINT ( 'NONE',  ( -56.48576386720575471, -142.0000000013656063, -4.591703134518078322 ) ) ;
#50407=CARTESIAN_POINT ( 'NONE',  ( -53.33387254593733928, -133.9375000027312410, 5.149110718188519620 ) ) ;
#50419=EDGE_CURVE ( 'NONE', #58935, #17875, #28798, .T. ) ;
#50425=CARTESIAN_POINT ( 'NONE',  ( -52.80376928212989185, -130.8750000013656063, -4.297418129356379346 ) ) ;
#50432=DIRECTION ( 'NONE',  ( -0.6485228581062915110, 0.000000000000000000, -0.7611951803011149931 ) ) ;
#50441=CARTESIAN_POINT ( 'NONE',  ( -55.35523342533222291, -136.3125000013656063, 4.444560631937231499 ) ) ;
#50453=CARTESIAN_POINT ( 'NONE',  ( -59.59170313451811296, -133.7500000013656063, 1.485763867205729394 ) ) ;
#50466=CARTESIAN_POINT ( 'NONE',  ( -58.24261429053147765, -138.3750000027312126, -3.805975901505573855 ) ) ;
#50473=ORIENTED_EDGE ( 'NONE', *, *, #61012, .F. ) ;
#50484=CARTESIAN_POINT ( 'NONE',  ( -55.39835681537999790, -151.8750000000000284, 4.984105922594378235 ) ) ;
#50494=CARTESIAN_POINT ( 'NONE',  ( -54.60164318462004474, -146.5000000027312126, -4.984105922594373794 ) ) ;
#50513=CARTESIAN_POINT ( 'NONE',  ( -58.39396692619412477, -150.4375000013656063, 2.891590998281057701 ) ) ;
#50516=DIRECTION ( 'NONE',  ( 0.000000000000000000, 1.000000000000000000, 0.000000000000000000 ) ) ;
#50553=CARTESIAN_POINT ( 'NONE',  ( -57.89159099828107458, -135.9375000013656063, -3.393966926194107447 ) ) ;
#50555=EDGE_LOOP ( 'NONE', ( #48097, #1689, #20594, #3257 ) ) ;
#50559=CARTESIAN_POINT ( 'NONE',  ( -55.80335512604638382, -135.0000000000000284, -4.395415492492952048 ) ) ;
#50560=ORIENTED_EDGE ( 'NONE', *, *, #10335, .F. ) ;
#50596=CARTESIAN_POINT ( 'NONE',  ( -56.48576386720575471, -139.0000000013655779, -4.591703134518078322 ) ) ;
#50621=CARTESIAN_POINT ( 'NONE',  ( -59.81910112700025905, -151.1875000000000000, -2.462841084822570359 ) ) ;
#50628=CARTESIAN_POINT ( 'NONE',  ( -52.80376928212989185, -147.1250000013656063, -4.297418129356379346 ) ) ;
#50632=CARTESIAN_POINT ( 'NONE',  ( -49.85088928181150436, -137.5625000000000000, -1.666127454062680480 ) ) ;
#50633=ORIENTED_EDGE ( 'NONE', *, *, #30288, .T. ) ;
#50634=CARTESIAN_POINT ( 'NONE',  ( -51.75738570946856498, -141.7500000000000284, 3.805975901505576964 ) ) ;
#50639=CARTESIAN_POINT ( 'NONE',  ( -59.98410592259440222, -128.1250000000000284, -0.3983568153799752487 ) ) ;
#50646=CARTESIAN_POINT ( 'NONE',  ( -56.48576386720575471, -153.7500000013656063, -4.591703134518078322 ) ) ;
#50662=DIRECTION ( 'NONE',  ( 0.8660254037844384856, 0.000000000000000000, -0.5000000000000002220 ) ) ;
#50669=CARTESIAN_POINT ( 'NONE',  ( -52.10840900171896806, -153.4375000013656063, 3.393966926194110556 ) ) ;
#50670=CARTESIAN_POINT ( 'NONE',  ( -52.80376928212989185, -140.8750000013656063, -4.297418129356378458 ) ) ;
#50709=CARTESIAN_POINT ( 'NONE',  ( -58.80597590150559739, -143.0000000000000284, 3.242614290531460330 ) ) ;
#50718=CARTESIAN_POINT ( 'NONE',  ( -58.39396692619412477, -143.6875000013656063, 2.891590998281057701 ) ) ;
#50720=CARTESIAN_POINT ( 'NONE',  ( -56.66612745406270335, -136.4375000027312126, -5.149110718188516067 ) ) ;
#50733=CARTESIAN_POINT ( 'NONE',  ( -53.51423613279429503, -127.2500000013656347, 4.591703134518082763 ) ) ;
#50748=CARTESIAN_POINT ( 'NONE',  ( -58.39396692619412477, -136.4375000013655779, 2.891590998281057701 ) ) ;
#50759=CARTESIAN_POINT ( 'NONE',  ( -52.10840900171896806, -131.4375000013656063, 3.393966926194110556 ) ) ;
#50799=CARTESIAN_POINT ( 'NONE',  ( -54.60164318462004474, -154.3750000000000284, -4.984105922594373794 ) ) ;
#50807=CARTESIAN_POINT ( 'NONE',  ( -58.39396692619412477, -152.6875000013656063, 2.891590998281057701 ) ) ;
#50809=CARTESIAN_POINT ( 'NONE',  ( -55.39835681537999790, -145.0000000027312126, 4.984105922594378235 ) ) ;
#50827=CARTESIAN_POINT ( 'NONE',  ( -50.40829686548195099, -149.0000000013656063, -1.485763867205728284 ) ) ;
#50833=CARTESIAN_POINT ( 'NONE',  ( -50.18089887299977647, -141.8125000027311842, 2.462841084822456672 ) ) ;
#50856=CARTESIAN_POINT ( 'NONE',  ( -55.00000000000002132, -155.0000000000000284, 1.734723475976807094E-15 ) ) ;
#50862=ORIENTED_EDGE ( 'NONE', *, *, #27921, .F. ) ;
#50872=CARTESIAN_POINT ( 'NONE',  ( -59.29741812935640155, -136.8750000013656063, -2.196230717870135685 ) ) ;
#50879=CARTESIAN_POINT ( 'NONE',  ( -51.41708869693315620, -135.0000000000000284, -2.669894875933531253 ) ) ;
#50899=CARTESIAN_POINT ( 'NONE',  ( -52.53715891517739323, -147.4375000000000284, -4.819101127000233298 ) ) ;
#50914=CARTESIAN_POINT ( 'NONE',  ( -53.51423613279429503, -138.5000000013656347, 4.591703134518082763 ) ) ;
#50936=CARTESIAN_POINT ( 'NONE',  ( -51.60603307380591787, -136.1875000013656063, -2.891590998281053704 ) ) ;
#50948=CARTESIAN_POINT ( 'NONE',  ( -54.64476657466781973, -147.0625000013656063, -4.444560631937228834 ) ) ;
#50955=CARTESIAN_POINT ( 'NONE',  ( -51.75738570946856498, -148.8750000027312126, 3.805975901505576964 ) ) ;
#50967=CARTESIAN_POINT ( 'NONE',  ( -50.40829686548195099, -148.0000000013655779, -1.485763867205728284 ) ) ;
#50982=CARTESIAN_POINT ( 'NONE',  ( -53.33387254593723270, -146.8125000000000284, 5.149110718188528502 ) ) ;
#50987=( BOUNDED_CURVE ( )  B_SPLINE_CURVE ( 2, ( #16907, #47136, #3397, #16595, #32017, #12716, #36525, #27197, #46503 ),
 .UNSPECIFIED., .F., .F. ) 
 B_SPLINE_CURVE_WITH_KNOTS ( ( 3, 2, 2, 2, 3 ),
 ( 0.07500000000000005274, 0.07916666666666671848, 0.08333333333333339810, 0.08750000000000007772, 0.09166666666666674346 ),
 .UNSPECIFIED. ) 
 CURVE ( )  GEOMETRIC_REPRESENTATION_ITEM ( )  RATIONAL_B_SPLINE_CURVE ( ( 0.9999999999999990008, 0.9238795325112877377, 1.000000000000000000, 0.9238795325112867385, 1.000000000000000000, 0.9238795325112867385, 1.000000000000000000, 0.9238795325112851842, 1.000000000000001554 ) ) 
 REPRESENTATION_ITEM ( '' )  );
#50995=CARTESIAN_POINT ( 'NONE',  ( -52.10840900171896806, -151.4375000013656063, 3.393966926194110556 ) ) ;
#50996=CARTESIAN_POINT ( 'NONE',  ( -56.48576386720575471, -142.7500000013655779, -4.591703134518078322 ) ) ;
#50999=CARTESIAN_POINT ( 'NONE',  ( -58.80597590150559739, -137.0000000000000284, 3.242614290531460330 ) ) ;
#51033=CARTESIAN_POINT ( 'NONE',  ( -52.53715891517739323, -140.4375000000000000, -4.819101127000233298 ) ) ;
#51042=CARTESIAN_POINT ( 'NONE',  ( -51.60603307380591787, -144.1875000013656063, -2.891590998281053704 ) ) ;
#51044=CARTESIAN_POINT ( 'NONE',  ( -50.01589407740564042, -128.7500000027312126, 0.3983568153799778022 ) ) ;
#51057=CARTESIAN_POINT ( 'NONE',  ( -51.60603307380591787, -130.9375000013656063, -2.891590998281053704 ) ) ;
#51063=CARTESIAN_POINT ( 'NONE',  ( -52.53715891517739323, -139.4375000000000284, -4.819101127000233298 ) ) ;
#51073=CARTESIAN_POINT ( 'NONE',  ( -58.39396692619412477, -133.4375000013656063, 2.891590998281057701 ) ) ;
#51086=CARTESIAN_POINT ( 'NONE',  ( -52.80376928212989185, -127.1250000013656205, -4.297418129356379346 ) ) ;
#51095=CARTESIAN_POINT ( 'NONE',  ( -48.00000000000002132, -135.0000000000000284, 4.041451884327384114 ) ) ;
#51098=DIRECTION ( 'NONE',  ( 0.000000000000000000, 1.000000000000000000, 0.000000000000000000 ) ) ;
#51112=CARTESIAN_POINT ( 'NONE',  ( -57.19623071787016499, -137.3750000013656063, 4.297418129356382899 ) ) ;
#51117=CARTESIAN_POINT ( 'NONE',  ( -51.60603307380591787, -125.1875000013656063, -2.891590998281053704 ) ) ;
#51131=CARTESIAN_POINT ( 'NONE',  ( -59.81910112700025905, -146.3125000027312410, -2.462841084822630311 ) ) ;
#51136=EDGE_CURVE ( 'NONE', #24361, #34224, #26368, .T. ) ;
#51154=CARTESIAN_POINT ( 'NONE',  ( -50.40829686548195099, -145.0000000013656063, -1.485763867205728284 ) ) ;
#51169=VECTOR ( 'NONE', #59077, 1000.000000000000000 ) ;
#51177=ORIENTED_EDGE ( 'NONE', *, *, #52869, .F. ) ;
#51190=VERTEX_POINT ( 'NONE', #60920 ) ;
#51199=CARTESIAN_POINT ( 'NONE',  ( -54.64476657466781973, -136.0625000013656063, -4.444560631937228834 ) ) ;
#51212=CARTESIAN_POINT ( 'NONE',  ( -58.24261429053147765, -149.2500000000000284, -3.805975901505573855 ) ) ;
#51222=ORIENTED_EDGE ( 'NONE', *, *, #23961, .T. ) ;
#51226=EDGE_CURVE ( 'NONE', #17875, #51190, #55120, .T. ) ;
#51231=DIRECTION ( 'NONE',  ( -0.6485228581062915110, 0.000000000000000000, -0.7611951803011149931 ) ) ;
#51244=CARTESIAN_POINT ( 'NONE',  ( -50.55543936806279248, -140.3125000013656063, 0.3552334253322060320 ) ) ;
#51262=( BOUNDED_CURVE ( )  B_SPLINE_CURVE ( 2, ( #6432, #2558, #1939, #36326, #21857, #12196, #55954, #7064, #31812, #51759, #51447, #21214, #22172, #26043, #61419, #7703, #2881, #17343, #40822, #56592, #12512, #32123, #61733, #27306, #46931, #22495, #17662, #37278, #56906, #12825, #32445, #60468, #50807, #16393, #11558, #36012, #55644, #53324, #33084, #33704, #9257, #4131, #62680, #52698, #27930, #18602, #62046, #52396, #13145, #32765, #13466, #8015, #8632, #3195, #27619, #48494, #47551, #8944, #17962, #22811, #38831, #18904, #28872, #3501, #33390, #38518, #42403, #37585, #23115, #4431, #28558, #43040, #42719, #57226, #28244, #24058, #58146, #8331, #57540, #48179, #14075, #43348, #62362, #43655, #63296, #47858, #57850, #14392, #47249, #19214, #58468, #3816, #18285, #52074, #37909, #23439, #38228, #23753, #13768, #53005, #62994, #6036, #35291, #15029, #15672, #54911, #63615, #19852, #49444, #59747, #58775, #19535, #14705, #29811, #60063, #59425, #10838, #34978, #39466, #25641, #30454, #9880, #54594, #43969, #48803, #20822, #34645, #898, #24683, #49122, #34324, #45257, #50079, #59102, #54269, #5386, #10516, #25001, #53949, #34015, #44940, #20505, #29486, #10209, #30130, #40103, #40423, #39149, #44611, #29177, #25320, #49759, #5064, #44292, #24367, #5705, #1223, #254, #53637, #571, #20180, #39778, #9570, #4742, #15354, #17259, #31097, #55874, #51042, #2175, #21781, #6985, #61336, #16313, #26596, #12109, #50718, #27226, #31736, #15987, #22413, #35934, #36882, #11786, #46536, #46213, #16625, #30782, #31404, #11160, #41373, #61019, #16945, #40740, #21459, #36558, #35612, #11477, #55561, #6662, #56189, #55238, #41059, #50404, #26269, #56512, #12433, #45891, #6353, #51366, #1853, #7307, #26919, #60705, #7622, #25957, #45574, #2477, #36247, #22090, #1530, #32045, #60387, #21135, #41689, #51681, #46847, #2794, #42012, #23359, #8250, #22730, #33310, #23041, #18524, #37828, #47471, #56829, #42644, #12747, #62285, #8553, #42328, #17889, #18207, #57462, #13064, #37509, #13381, #13691, #33002, #17586, #27850, #37203, #61968, #52930, #28482, #57149, #32367, #28166, #32684, #38144, #48098, #52619, #47781, #3738, #52315, #3425, #42958, #62601, #57769, #8867, #3112, #51991, #27537, #4052, #23670, #43268, #62907, #18821, #61652, #7935, #47169, #56081, #31299, #21985, #1748, #55764, #16520, #36143, #16834, #11366, #36454, #6554, #30989, #51886, #50936, #12333, #21349, #26168, #42225, #22304, #56722, #6877, #36777, #41903, #45789, #40953, #26491, #7827, #31944, #46427, #46107, #60601, #31629, #27429, #61550 ),
 .UNSPECIFIED., .F., .F. ) 
 B_SPLINE_CURVE_WITH_KNOTS ( ( 3, 2, 2, 2, 2, 2, 2, 2, 2, 2, 2, 2, 2, 2, 2, 2, 2, 2, 2, 2, 2, 2, 2, 2, 2, 2, 2, 2, 2, 2, 2, 2, 2, 2, 2, 2, 2, 2, 2, 2, 2, 2, 2, 2, 2, 2, 2, 2, 2, 2, 2, 2, 2, 2, 2, 2, 2, 2, 2, 2, 2, 2, 2, 2, 2, 2, 2, 2, 2, 2, 2, 2, 2, 2, 2, 2, 2, 2, 2, 2, 2, 2, 2, 2, 2, 2, 2, 2, 2, 2, 2, 2, 2, 2, 2, 2, 2, 2, 2, 2, 2, 2, 2, 2, 2, 2, 2, 2, 2, 2, 2, 2, 2, 2, 2, 2, 2, 2, 2, 2, 2, 2, 2, 2, 2, 2, 2, 2, 2, 2, 2, 2, 2, 2, 2, 2, 2, 2, 2, 2, 2, 2, 2, 2, 2, 2, 2, 2, 2, 2, 2, 2, 2, 2, 2, 2, 2, 2, 3 ),
 ( 0.000000000000000000, 0.004166666666666666609, 0.008333333333333333218, 0.01250000000000000243, 0.01666666666666666644, 0.02083333333333333218, 0.02500000000000000486, 0.02916666666666666713, 0.03333333333333333287, 0.03749999999999999861, 0.04166666666666666435, 0.04583333333333333010, 0.05000000000000000971, 0.05416666666666666852, 0.05833333333333333426, 0.06250000000000000000, 0.06666666666666666574, 0.07083333333333333148, 0.07499999999999999722, 0.07916666666666666297, 0.08333333333333332871, 0.08749999999999999445, 0.09166666666666666019, 0.09583333333333333981, 0.1000000000000000194, 0.1041666666666666713, 0.1083333333333333370, 0.1124999999999999889, 0.1166666666666666685, 0.1208333333333333204, 0.1250000000000000000, 0.1291666666666666796, 0.1333333333333333315, 0.1375000000000000111, 0.1416666666666666630, 0.1458333333333333426, 0.1499999999999999944, 0.1541666666666666741, 0.1583333333333333259, 0.1625000000000000056, 0.1666666666666666574, 0.1708333333333333370, 0.1749999999999999889, 0.1791666666666666685, 0.1833333333333333204, 0.1875000000000000000, 0.1916666666666666796, 0.1958333333333333592, 0.2000000000000000389, 0.2041666666666666630, 0.2083333333333333426, 0.2125000000000000222, 0.2166666666666666741, 0.2208333333333333259, 0.2249999999999999778, 0.2291666666666666574, 0.2333333333333333370, 0.2374999999999999611, 0.2416666666666666408, 0.2458333333333333204, 0.2500000000000000000, 0.2541666666666666519, 0.2583333333333333592, 0.2625000000000000111, 0.2666666666666666630, 0.2708333333333333148, 0.2750000000000000222, 0.2791666666666666741, 0.2833333333333333259, 0.2874999999999999778, 0.2916666666666666852, 0.2958333333333333370, 0.2999999999999999889, 0.3041666666666666408, 0.3083333333333333481, 0.3125000000000000000, 0.3166666666666666519, 0.3208333333333333592, 0.3250000000000000111, 0.3291666666666666630, 0.3333333333333333148, 0.3375000000000000222, 0.3416666666666666741, 0.3458333333333333259, 0.3499999999999999778, 0.3541666666666666852, 0.3583333333333333370, 0.3624999999999999889, 0.3666666666666666408, 0.3708333333333333481, 0.3750000000000000000, 0.3791666666666666519, 0.3833333333333333592, 0.3874999999999999556, 0.3916666666666667185, 0.3958333333333333148, 0.4000000000000000777, 0.4041666666666666741, 0.4083333333333333259, 0.4124999999999999223, 0.4166666666666666852, 0.4208333333333332815, 0.4250000000000000444, 0.4291666666666666408, 0.4333333333333333481, 0.4375000000000000000, 0.4416666666666666519, 0.4458333333333333592, 0.4499999999999999556, 0.4541666666666667185, 0.4583333333333333148, 0.4625000000000000777, 0.4666666666666666741, 0.4708333333333333259, 0.4749999999999999223, 0.4791666666666666852, 0.4833333333333332815, 0.4875000000000000444, 0.4916666666666666408, 0.4958333333333333481, 0.5000000000000000000, 0.5041666666666666519, 0.5083333333333333037, 0.5124999999999999556, 0.5166666666666667185, 0.5208333333333333703, 0.5250000000000000222, 0.5291666666666666741, 0.5333333333333333259, 0.5374999999999999778, 0.5416666666666666297, 0.5458333333333332815, 0.5500000000000000444, 0.5541666666666666963, 0.5583333333333333481, 0.5625000000000000000, 0.5666666666666666519, 0.5708333333333333037, 0.5749999999999999556, 0.5791666666666667185, 0.5833333333333333703, 0.5875000000000000222, 0.5916666666666666741, 0.5958333333333333259, 0.5999999999999999778, 0.6041666666666666297, 0.6083333333333332815, 0.6125000000000000444, 0.6166666666666666963, 0.6208333333333333481, 0.6250000000000000000, 0.6291666666666666519, 0.6333333333333333037, 0.6374999999999999556, 0.6416666666666667185, 0.6458333333333333703, 0.6500000000000000222, 0.6541666666666666741, 0.6562500000437863079 ),
 .UNSPECIFIED. ) 
 CURVE ( )  GEOMETRIC_REPRESENTATION_ITEM ( )  RATIONAL_B_SPLINE_CURVE ( ( 1.000000000000000000, 0.9238795325112867385, 1.000000000000000000, 0.9238795325112867385, 1.000000000000000000, 0.9238795325112867385, 1.000000000000000000, 0.9238795325112867385, 1.000000000000000000, 0.9238795325112867385, 1.000000000000000000, 0.9238795325112867385, 1.000000000000000000, 0.9238795325112867385, 1.000000000000000000, 0.9238795325112867385, 1.000000000000000000, 0.9238795325112867385, 1.000000000000000000, 0.9238795325112867385, 1.000000000000000000, 0.9238795325112867385, 1.000000000000000000, 0.9238795325112867385, 1.000000000000000000, 0.9238795325112867385, 1.000000000000000000, 0.9238795325112867385, 1.000000000000000000, 0.9238795325112867385, 1.000000000000000000, 0.9238795325112867385, 1.000000000000000000, 0.9238795325112867385, 1.000000000000000000, 0.9238795325112867385, 1.000000000000000000, 0.9238795325112867385, 1.000000000000000000, 0.9238795325112867385, 1.000000000000000000, 0.9238795325112867385, 1.000000000000000000, 0.9238795325112867385, 1.000000000000000000, 0.9238795325112867385, 1.000000000000000000, 0.9238795325112867385, 1.000000000000000000, 0.9238795325112867385, 1.000000000000000000, 0.9238795325112867385, 1.000000000000000000, 0.9238795325112867385, 1.000000000000000000, 0.9238795325112867385, 1.000000000000000000, 0.9238795325112867385, 1.000000000000000000, 0.9238795325112867385, 1.000000000000000000, 0.9238795325112867385, 1.000000000000000000, 0.9238795325112867385, 1.000000000000000000, 0.9238795325112867385, 1.000000000000000000, 0.9238795325112867385, 1.000000000000000000, 0.9238795325112867385, 1.000000000000000000, 0.9238795325112867385, 1.000000000000000000, 0.9238795325112867385, 1.000000000000000000, 0.9238795325112867385, 1.000000000000000000, 0.9238795325112867385, 1.000000000000000000, 0.9238795325112867385, 1.000000000000000000, 0.9238795325112867385, 1.000000000000000000, 0.9238795325112867385, 1.000000000000000000, 0.9238795325112867385, 1.000000000000000000, 0.9238795325112867385, 1.000000000000000000, 0.9238795325112867385, 1.000000000000000000, 0.9238795325112867385, 1.000000000000000000, 0.9238795325112867385, 1.000000000000000000, 0.9238795325112867385, 1.000000000000000000, 0.9238795325112867385, 1.000000000000000000, 0.9238795325112867385, 1.000000000000000000, 0.9238795325112867385, 1.000000000000000000, 0.9238795325112867385, 1.000000000000000000, 0.9238795325112867385, 1.000000000000000000, 0.9238795325112867385, 1.000000000000000000, 0.9238795325112867385, 1.000000000000000000, 0.9238795325112867385, 1.000000000000000000, 0.9238795325112867385, 1.000000000000000000, 0.9238795325112867385, 1.000000000000000000, 0.9238795325112867385, 1.000000000000000000, 0.9238795325112867385, 1.000000000000000000, 0.9238795325112867385, 1.000000000000000000, 0.9238795325112867385, 1.000000000000000000, 0.9238795325112867385, 1.000000000000000000, 0.9238795325112867385, 1.000000000000000000, 0.9238795325112867385, 1.000000000000000000, 0.9238795325112867385, 1.000000000000000000, 0.9238795325112867385, 1.000000000000000000, 0.9238795325112867385, 1.000000000000000000, 0.9238795325112867385, 1.000000000000000000, 0.9238795325112867385, 1.000000000000000000, 0.9238795325112867385, 1.000000000000000000, 0.9238795325112867385, 1.000000000000000000, 0.9238795325112867385, 1.000000000000000000, 0.9238795325112867385, 1.000000000000000000, 0.9238795325112867385, 1.000000000000000000, 0.9238795325112867385, 1.000000000000000000, 0.9238795325112867385, 1.000000000000000000, 0.9238795325112867385, 1.000000000000000000, 0.9238795325112867385, 1.000000000000000000, 0.9238795325112867385, 1.000000000000000000, 0.9238795325112867385, 1.000000000000000000, 0.9238795325112867385, 1.000000000000000000, 0.9238795325112867385, 1.000000000000000000, 0.9238795325112867385, 1.000000000000000000, 0.9238795325112867385, 1.000000000000000000, 0.9238795325112867385, 1.000000000000000000, 0.9238795325112867385, 1.000000000000000000, 0.9238795325112867385, 1.000000000000000000, 0.9238795325112867385, 1.000000000000000000, 0.9238795325112867385, 1.000000000000000000, 0.9238795325112867385, 1.000000000000000000, 0.9238795325112867385, 1.000000000000000000, 0.9238795325112867385, 1.000000000000000000, 0.9238795325112867385, 1.000000000000000000, 0.9238795325112867385, 1.000000000000000000, 0.9238795325112867385, 1.000000000000000000, 0.9238795325112867385, 1.000000000000000000, 0.9238795325112867385, 1.000000000000000000, 0.9238795325112867385, 1.000000000000000000, 0.9238795325112867385, 1.000000000000000000, 0.9238795325112867385, 1.000000000000000000, 0.9238795325112867385, 1.000000000000000000, 0.9238795325112867385, 1.000000000000000000, 0.9238795325112867385, 1.000000000000000000, 0.9238795325112867385, 1.000000000000000000, 0.9238795325112867385, 1.000000000000000000, 0.9238795325112867385, 1.000000000000000000, 0.9238795325112867385, 1.000000000000000000, 0.9238795325112867385, 1.000000000000000000, 0.9238795325112867385, 1.000000000000000000, 0.9238795325112867385, 1.000000000000000000, 0.9238795325112867385, 1.000000000000000000, 0.9238795325112867385, 1.000000000000000000, 0.9238795325112867385, 1.000000000000000000, 0.9238795325112867385, 1.000000000000000000, 0.9238795325112867385, 1.000000000000000000, 0.9238795325112867385, 1.000000000000000000, 0.9238795325112867385, 1.000000000000000000, 0.9238795325112867385, 1.000000000000000000, 0.9238795325112867385, 1.000000000000000000, 0.9238795325112867385, 1.000000000000000000, 0.9238795325112867385, 1.000000000000000000, 0.9238795325112867385, 1.000000000000000000, 0.9238795325112867385, 1.000000000000000000, 0.9238795325112867385, 1.000000000000000000, 0.9238795325112867385, 1.000000000000000000, 0.9238795325112867385, 1.000000000000000000, 0.9238795325112867385, 1.000000000000000000, 0.9238795325112867385, 1.000000000000000000, 0.9238795325112867385, 1.000000000000000000, 0.9238795325112867385, 1.000000000000000000, 0.9238795325112867385, 1.000000000000000000, 0.9238795325112867385, 1.000000000000000000, 0.9238795325112867385, 1.000000000000000000, 0.9238795325112867385, 1.000000000000000000, 0.9238795325112867385, 1.000000000000000000, 0.9238795325112867385, 1.000000000000000000, 0.9238795325112867385, 1.000000000000000000, 0.9238795325112867385, 1.000000000000000000, 0.9238795325112867385, 1.000000000000000000, 0.9238795325112867385, 1.000000000000000000, 0.9238795325112867385, 1.000000000000000000, 0.9238795325112867385, 1.000000000000000000, 0.9238795325112867385, 1.000000000000000000, 0.9238795325112867385, 1.000000000000000000, 0.9238795325112867385, 1.000000000000000000, 0.9238795325112867385, 1.000000000000000000, 0.9238795325112867385, 1.000000000000000000, 0.9238795325112867385, 1.000000000000000000, 0.9238795325112867385, 1.000000000000000000, 0.9238795325112867385, 1.000000000000000000, 0.9238795325112867385, 1.000000000000000000, 0.9238795325112867385, 1.000000000000000000, 0.9238795325112867385, 1.000000000000000000, 0.9238795325112867385, 1.000000000000000000, 0.9238795325112867385, 1.000000000000000000, 0.9238795325112867385, 1.000000000000000000, 0.9619397654557151345, 0.9619397662556433692 ) ) 
 REPRESENTATION_ITEM ( '' )  );
#51277=CARTESIAN_POINT ( 'NONE',  ( -55.35523342533222291, -145.5625000013656063, 4.444560631937231499 ) ) ;
#51285=PLANE ( 'NONE',  #11203 ) ;
#51297=CARTESIAN_POINT ( 'NONE',  ( -52.10840900171896806, -149.1875000013656063, 3.393966926194110556 ) ) ;
#51301=ORIENTED_EDGE ( 'NONE', *, *, #54250, .T. ) ;
#51310=CYLINDRICAL_SURFACE ( 'NONE', #36783, 5.000000000000000000 ) ;
#51320=CARTESIAN_POINT ( 'NONE',  ( -50.70258187064364108, -151.3750000013656063, 2.196230717870141014 ) ) ;
#51330=ORIENTED_EDGE ( 'NONE', *, *, #30288, .F. ) ;
#51344=DIRECTION ( 'NONE',  ( -0.000000000000000000, 1.000000000000000000, -0.000000000000000000 ) ) ;
#51345=VERTEX_POINT ( 'NONE', #43170 ) ;
#51357=CARTESIAN_POINT ( 'NONE',  ( -59.98410592259440222, -137.1250000000000284, -0.3983568153799752487 ) ) ;
#51366=CARTESIAN_POINT ( 'NONE',  ( -57.19623071787016499, -141.6250000013655495, 4.297418129356382899 ) ) ;
#51368=CARTESIAN_POINT ( 'NONE',  ( -49.85088928181150436, -128.6875000027312410, -1.666127454062680702 ) ) ;
#51380=CARTESIAN_POINT ( 'NONE',  ( -58.24261429053147765, -154.2500000000000284, -3.805975901505573855 ) ) ;
#51381=CARTESIAN_POINT ( 'NONE',  ( -53.51423613279429503, -125.2500000013656347, 4.591703134518082763 ) ) ;
#51383=CARTESIAN_POINT ( 'NONE',  ( -59.81910112700026616, -142.3125000027311842, -2.462841084822451343 ) ) ;
#51387=CARTESIAN_POINT ( 'NONE',  ( -56.66612745406283125, -146.3125000000000284, -5.149110718188525837 ) ) ;
#51394=CARTESIAN_POINT ( 'NONE',  ( -57.89159099828107458, -132.6875000013656063, -3.393966926194107447 ) ) ;
#51403=CARTESIAN_POINT ( 'NONE',  ( -53.51423613279429503, -126.5000000013656063, 4.591703134518082763 ) ) ;
#51425=CARTESIAN_POINT ( 'NONE',  ( -50.70258187064364108, -153.3750000013656347, 2.196230717870141014 ) ) ;
#51429=CARTESIAN_POINT ( 'NONE',  ( -53.51423613279429503, -138.2500000013656063, 4.591703134518083651 ) ) ;
#51436=CARTESIAN_POINT ( 'NONE',  ( -58.24261429053147765, -151.2500000000000284, -3.805975901505573855 ) ) ;
#51447=CARTESIAN_POINT ( 'NONE',  ( -54.64476657466781973, -154.0625000013656347, -4.444560631937228834 ) ) ;
#51448=CARTESIAN_POINT ( 'NONE',  ( -59.81910112700025905, -141.3125000027312126, -2.462841084822630311 ) ) ;
#51457=CARTESIAN_POINT ( 'NONE',  ( -59.29741812935640155, -136.6250000013655779, -2.196230717870135685 ) ) ;
#51469=CARTESIAN_POINT ( 'NONE',  ( -52.80376928212989185, -146.8750000013656063, -4.297418129356379346 ) ) ;
#51475=CARTESIAN_POINT ( 'NONE',  ( -51.75738570946856498, -141.8750000027312126, 3.805975901505576964 ) ) ;
#51499=CARTESIAN_POINT ( 'NONE',  ( -55.00000000000002132, -155.0000000000000284, 1.734723475976807094E-15 ) ) ;
#51515=CARTESIAN_POINT ( 'NONE',  ( -50.40829686548195099, -134.2500000013656063, -1.485763867205728284 ) ) ;
#51555=CARTESIAN_POINT ( 'NONE',  ( -59.44456063193725015, -138.8125000013656063, -0.3552334253322034230 ) ) ;
#51562=EDGE_LOOP ( 'NONE', ( #15376, #14153, #33001, #85 ) ) ;
#51581=CARTESIAN_POINT ( 'NONE',  ( -55.39835681537999790, -138.8750000000000284, 4.984105922594378235 ) ) ;
#51587=CARTESIAN_POINT ( 'NONE',  ( -55.35523342533222291, -148.5625000013656063, 4.444560631937231499 ) ) ;
#51599=EDGE_CURVE ( 'NONE', #28712, #28080, #50987, .T. ) ;
#51604=CARTESIAN_POINT ( 'NONE',  ( -58.24261429053147765, -125.2500000000000284, -3.805975901505573855 ) ) ;
#51611=CARTESIAN_POINT ( 'NONE',  ( -50.40829686548195099, -150.0000000013655779, -1.485763867205728284 ) ) ;
#51635=CARTESIAN_POINT ( 'NONE',  ( -57.19623071787017210, -152.6250000013656063, 4.297418129356382899 ) ) ;
#51642=CARTESIAN_POINT ( 'NONE',  ( -60.14911071818854538, -138.1875000027312126, 1.666127454062681146 ) ) ;
#51672=CARTESIAN_POINT ( 'NONE',  ( -59.81910112700025905, -138.1875000000000000, -2.462841084822630311 ) ) ;
#51681=CARTESIAN_POINT ( 'NONE',  ( -57.19623071787016499, -140.6250000013656063, 4.297418129356382899 ) ) ;
#51683=CARTESIAN_POINT ( 'NONE',  ( -59.81910112700025905, -130.3125000027312410, -2.462841084822630311 ) ) ;
#51695=CARTESIAN_POINT ( 'NONE',  ( -50.55543936806279248, -126.0625000013655921, 0.3552334253322060320 ) ) ;
#51708=CARTESIAN_POINT ( 'NONE',  ( -53.51423613279429503, -135.2500000013656347, 4.591703134518082763 ) ) ;
#51718=CARTESIAN_POINT ( 'NONE',  ( -58.39396692619412477, -127.6875000013656063, 2.891590998281057701 ) ) ;
#51734=CARTESIAN_POINT ( 'NONE',  ( -58.24261429053147765, -139.3750000027312126, -3.805975901505573855 ) ) ;
#51745=CARTESIAN_POINT ( 'NONE',  ( -53.51423613279429503, -140.2500000013656063, 4.591703134518083651 ) ) ;
#51750=CARTESIAN_POINT ( 'NONE',  ( -56.66612745406270335, -150.3125000000000284, -5.149110718188516067 ) ) ;
#51754=SURFACE_STYLE_USAGE ( .BOTH. , #2875 ) ;
#51759=CARTESIAN_POINT ( 'NONE',  ( -52.80376928212989185, -154.1250000013656063, -4.297418129356378458 ) ) ;
#51760=CARTESIAN_POINT ( 'NONE',  ( -51.75738570946856498, -142.8750000027312126, 3.805975901505576964 ) ) ;
#51767=CARTESIAN_POINT ( 'NONE',  ( -58.39396692619412477, -138.4375000013656063, 2.891590998281057701 ) ) ;
#51782=CARTESIAN_POINT ( 'NONE',  ( -50.55543936806279248, -146.0625000013656063, 0.3552334253322060320 ) ) ;
#51812=ORIENTED_EDGE ( 'NONE', *, *, #9968, .F. ) ;
#51821=CARTESIAN_POINT ( 'NONE',  ( -59.59170313451811296, -132.7500000013656063, 1.485763867205729394 ) ) ;
#51851=CARTESIAN_POINT ( 'NONE',  ( -51.19402409849444524, -138.5000000000000284, -3.242614290531456334 ) ) ;
#51866=CARTESIAN_POINT ( 'NONE',  ( -52.80376928212989185, -140.1250000013655779, -4.297418129356379346 ) ) ;
#51886=CARTESIAN_POINT ( 'NONE',  ( -50.40829686548195099, -136.2500000013656063, -1.485763867205728284 ) ) ;
#51898=CARTESIAN_POINT ( 'NONE',  ( -50.55543936806279248, -144.3125000013656063, 0.3552334253322060320 ) ) ;
#51902=EDGE_CURVE ( 'NONE', #33278, #56532, #4630, .T. ) ;
#51910=CARTESIAN_POINT ( 'NONE',  ( -57.46284108482265651, -126.9375000000000284, 4.819101127000239515 ) ) ;
#51917=CARTESIAN_POINT ( 'NONE',  ( -50.70258187064364108, -147.1250000013656063, 2.196230717870141014 ) ) ;
#51931=CARTESIAN_POINT ( 'NONE',  ( -50.01589407740564042, -140.7500000027312126, 0.3983568153799778022 ) ) ;
#51945=CARTESIAN_POINT ( 'NONE',  ( -58.39396692619412477, -150.6875000013656063, 2.891590998281057701 ) ) ;
#51981=CARTESIAN_POINT ( 'NONE',  ( -52.53715891517739323, -137.4375000000000284, -4.819101127000233298 ) ) ;
#51991=CARTESIAN_POINT ( 'NONE',  ( -57.19623071787016499, -137.6250000013655779, 4.297418129356382899 ) ) ;
#51993=CARTESIAN_POINT ( 'NONE',  ( -52.53715891517739323, -129.5625000027312410, -4.819101127000233298 ) ) ;
#51999=CARTESIAN_POINT ( 'NONE',  ( -57.46284108482265651, -151.0625000027312126, 4.819101127000238627 ) ) ;
#52008=CARTESIAN_POINT ( 'NONE',  ( -57.89159099828107458, -125.6875000013656063, -3.393966926194107447 ) ) ;
#52019=CARTESIAN_POINT ( 'NONE',  ( -57.19623071787017210, -135.3750000013656063, 4.297418129356382899 ) ) ;
#52031=CARTESIAN_POINT ( 'NONE',  ( -50.70258187064364108, -128.3750000013656631, 2.196230717870141014 ) ) ;
#52061=CARTESIAN_POINT ( 'NONE',  ( -54.64476657466781973, -139.8125000013656063, -4.444560631937228834 ) ) ;
#52066=CARTESIAN_POINT ( 'NONE',  ( -59.81910112700025905, -148.1875000000000284, -2.462841084822630311 ) ) ;
#52074=CARTESIAN_POINT ( 'NONE',  ( -59.29741812935640155, -148.8750000013656063, -2.196230717870135685 ) ) ;
#52075=CARTESIAN_POINT ( 'NONE',  ( -57.46284108482265651, -141.0625000027312410, 4.819101127000239515 ) ) ;
#52085=CARTESIAN_POINT ( 'NONE',  ( -53.51423613279429503, -138.2500000013656063, 4.591703134518082763 ) ) ;
#52099=CARTESIAN_POINT ( 'NONE',  ( -52.10840900171896806, -146.1875000013656063, 3.393966926194110556 ) ) ;
#52131=LINE ( 'NONE', #53694, #34332 ) ;
#52142=CARTESIAN_POINT ( 'NONE',  ( -56.48576386720575471, -133.0000000013656063, -4.591703134518078322 ) ) ;
#52148=ORIENTED_EDGE ( 'NONE', *, *, #58343, .T. ) ;
#52149=CARTESIAN_POINT ( 'NONE',  ( -59.98410592259440222, -153.2500000027312410, -0.3983568153799752487 ) ) ;
#52157=CARTESIAN_POINT ( 'NONE',  ( -58.80597590150559739, -147.1250000027312126, 3.242614290531460330 ) ) ;
#52167=CARTESIAN_POINT ( 'NONE',  ( -49.85088928181150436, -138.5625000000000284, -1.666127454062680480 ) ) ;
#52181=CARTESIAN_POINT ( 'NONE',  ( -58.39396692619412477, -136.6875000013656063, 2.891590998281057701 ) ) ;
#52197=( BOUNDED_CURVE ( )  B_SPLINE_CURVE ( 2, ( #59826, #20256, #644, #44042, #53707, #4820, #45014, #30530, #19923 ),
 .UNSPECIFIED., .F., .F. ) 
 B_SPLINE_CURVE_WITH_KNOTS ( ( 3, 2, 2, 2, 3 ),
 ( 0.5750000000000005107, 0.5791666666666672736, 0.5833333333333339255, 0.5875000000000004663, 0.5916666666666671182 ),
 .UNSPECIFIED. ) 
 CURVE ( )  GEOMETRIC_REPRESENTATION_ITEM ( )  RATIONAL_B_SPLINE_CURVE ( ( 0.9999999999999898970, 0.9238795325112968415, 1.000000000000000000, 0.9238795325112867385, 1.000000000000000000, 0.9238795325112867385, 1.000000000000000000, 0.9238795325112786339, 1.000000000000008216 ) ) 
 REPRESENTATION_ITEM ( '' )  );
#52203=CARTESIAN_POINT ( 'NONE',  ( -58.24261429053147765, -138.3750000027312126, -3.805975901505573855 ) ) ;
#52206=CARTESIAN_POINT ( 'NONE',  ( -51.75738570946856498, -138.7500000000000000, 3.805975901505576964 ) ) ;
#52215=CARTESIAN_POINT ( 'NONE',  ( -53.51423613279429503, -143.5000000013656347, 4.591703134518082763 ) ) ;
#52222=LINE ( 'NONE', #47394, #28637 ) ;
#52225=CARTESIAN_POINT ( 'NONE',  ( -49.85088928181150436, -125.5625000000000284, -1.666127454062680702 ) ) ;
#52235=CARTESIAN_POINT ( 'NONE',  ( -59.59170313451811296, -148.5000000013655779, 1.485763867205729394 ) ) ;
#52255=CARTESIAN_POINT ( 'NONE',  ( -55.39835681537999790, -140.0000000027312126, 4.984105922594378235 ) ) ;
#52263=CARTESIAN_POINT ( 'NONE',  ( -52.80376928212989185, -149.1250000013656063, -4.297418129356379346 ) ) ;
#52293=EDGE_CURVE ( 'NONE', #61334, #55226, #15300, .T. ) ;
#52299=LINE ( 'NONE', #23029, #23430 ) ;
#52304=CARTESIAN_POINT ( 'NONE',  ( -58.80597590150559739, -137.0000000000000284, 3.242614290531460330 ) ) ;
#52315=CARTESIAN_POINT ( 'NONE',  ( -54.64476657466781973, -138.0625000013656063, -4.444560631937228834 ) ) ;
#52317=CARTESIAN_POINT ( 'NONE',  ( -51.19402409849444524, -130.6250000027312126, -3.242614290531456334 ) ) ;
#52340=CARTESIAN_POINT ( 'NONE',  ( -56.48576386720575471, -131.7500000013656063, -4.591703134518078322 ) ) ;
#52350=CARTESIAN_POINT ( 'NONE',  ( -50.70258187064364108, -127.3750000013656205, 2.196230717870141014 ) ) ;
#52378=CARTESIAN_POINT ( 'NONE',  ( -50.55543936806279248, -140.0625000013656063, 0.3552334253322060320 ) ) ;
#52383=CARTESIAN_POINT ( 'NONE',  ( -49.85088928181150436, -151.5625000000000284, -1.666127454062680702 ) ) ;
#52396=CARTESIAN_POINT ( 'NONE',  ( -59.59170313451810586, -151.7500000013656063, 1.485763867205729394 ) ) ;
#52397=CARTESIAN_POINT ( 'NONE',  ( -50.18089887299979068, -140.8125000027311842, 2.462841084822635640 ) ) ;
#52408=CARTESIAN_POINT ( 'NONE',  ( -50.70258187064364108, -136.1250000013656063, 2.196230717870141014 ) ) ;
#52414=ORIENTED_EDGE ( 'NONE', *, *, #51136, .T. ) ;
#52422=CARTESIAN_POINT ( 'NONE',  ( -57.89159099828107458, -145.6875000013656063, -3.393966926194107447 ) ) ;
#52440=CYLINDRICAL_SURFACE ( 'NONE', #37748, 5.000000000000000000 ) ;
#52463=CARTESIAN_POINT ( 'NONE',  ( -57.89159099828107458, -131.9375000013656063, -3.393966926194107447 ) ) ;
#52470=CARTESIAN_POINT ( 'NONE',  ( -56.66612745406270335, -153.4375000027311842, -5.149110718188516067 ) ) ;
#52503=CARTESIAN_POINT ( 'NONE',  ( -58.24261429053147765, -155.0000000000000284, -3.805975901505573411 ) ) ;
#52506=CARTESIAN_POINT ( 'NONE',  ( -57.89159099828107458, -134.9375000013656063, -3.393966926194107447 ) ) ;
#52535=CARTESIAN_POINT ( 'NONE',  ( -51.60603307380591787, -142.1875000013656063, -2.891590998281053704 ) ) ;
#52553=CARTESIAN_POINT ( 'NONE',  ( -55.35523342533222291, -144.3125000013656063, 4.444560631937231499 ) ) ;
#52578=CARTESIAN_POINT ( 'NONE',  ( -50.40829686548195099, -146.2500000013656063, -1.485763867205728284 ) ) ;
#52585=CARTESIAN_POINT ( 'NONE',  ( -57.46284108482265651, -138.0625000027312126, 4.819101127000238627 ) ) ;
#52607=ORIENTED_EDGE ( 'NONE', *, *, #16429, .F. ) ;
#52611=CARTESIAN_POINT ( 'NONE',  ( -59.81910112700025905, -136.1875000000000000, -2.462841084822630311 ) ) ;
#52619=CARTESIAN_POINT ( 'NONE',  ( -50.40829686548195099, -138.2500000013656063, -1.485763867205728284 ) ) ;
#52621=CARTESIAN_POINT ( 'NONE',  ( -50.18089887299979068, -124.8125000027312126, 2.462841084822635640 ) ) ;
#52634=CARTESIAN_POINT ( 'NONE',  ( -59.29741812935640155, -126.6250000013656489, -2.196230717870135685 ) ) ;
#52646=CARTESIAN_POINT ( 'NONE',  ( -56.48576386720575471, -128.7500000013656063, -4.591703134518078322 ) ) ;
#52654=ORIENTED_EDGE ( 'NONE', *, *, #31628, .T. ) ;
#52669=ORIENTED_EDGE ( 'NONE', *, *, #46485, .F. ) ;
#52680=CARTESIAN_POINT ( 'NONE',  ( -55.35523342533222291, -154.5625000013656347, 4.444560631937231499 ) ) ;
#52688=CARTESIAN_POINT ( 'NONE',  ( -51.75738570946856498, -147.7500000000000284, 3.805975901505576964 ) ) ;
#52698=CARTESIAN_POINT ( 'NONE',  ( -56.48576386720575471, -152.0000000013656063, -4.591703134518078322 ) ) ;
#52699=CARTESIAN_POINT ( 'NONE',  ( -59.98410592259440222, -142.2500000027312126, -0.3983568153799752487 ) ) ;
#52707=CARTESIAN_POINT ( 'NONE',  ( -50.55543936806279248, -136.0625000013656063, 0.3552334253322060320 ) ) ;
#52721=DIRECTION ( 'NONE',  ( 0.000000000000000000, 1.000000000000000000, 0.000000000000000000 ) ) ;
#52722=CARTESIAN_POINT ( 'NONE',  ( -57.89159099828107458, -142.6875000013656063, -3.393966926194107447 ) ) ;
#52748=VERTEX_POINT ( 'NONE', #54532 ) ;
#52762=CARTESIAN_POINT ( 'NONE',  ( -59.29741812935640155, -153.6250000013655779, -2.196230717870135685 ) ) ;
#52769=CARTESIAN_POINT ( 'NONE',  ( -53.51423613279429503, -132.5000000013656063, 4.591703134518082763 ) ) ;
#52778=CARTESIAN_POINT ( 'NONE',  ( -52.53715891517739323, -153.5625000027312410, -4.819101127000233298 ) ) ;
#52796=CARTESIAN_POINT ( 'NONE',  ( -57.46284108482265651, -144.9375000000000000, 4.819101127000238627 ) ) ;
#52797=CARTESIAN_POINT ( 'NONE',  ( -52.10840900171896806, -154.1875000013656063, 3.393966926194110556 ) ) ;
#52811=CARTESIAN_POINT ( 'NONE',  ( -52.80376928212989185, -134.1250000013656347, -4.297418129356379346 ) ) ;
#52813=CARTESIAN_POINT ( 'NONE',  ( -51.75738570946856498, -145.7500000000000284, 3.805975901505576964 ) ) ;
#52843=CARTESIAN_POINT ( 'NONE',  ( -59.44456063193725015, -143.8125000013656063, -0.3552334253322034230 ) ) ;
#52848=VERTEX_POINT ( 'NONE', #62464 ) ;
#52858=VECTOR ( 'NONE', #63048, 1000.000000000000000 ) ;
#52862=CARTESIAN_POINT ( 'NONE',  ( -50.70258187064364108, -144.1250000013656063, 2.196230717870141014 ) ) ;
#52869=EDGE_CURVE ( 'NONE', #51190, #58682, #16983, .T. ) ;
#52887=CARTESIAN_POINT ( 'NONE',  ( -57.89159099828107458, -149.9375000013656063, -3.393966926194107447 ) ) ;
#52921=CARTESIAN_POINT ( 'NONE',  ( -52.53715891517739323, -133.4375000000000284, -4.819101127000233298 ) ) ;
#52930=CARTESIAN_POINT ( 'NONE',  ( -59.59170313451810586, -138.7500000013655779, 1.485763867205729394 ) ) ;
#52932=CARTESIAN_POINT ( 'NONE',  ( -49.85088928181150436, -124.6875000027312268, -1.666127454062680702 ) ) ;
#52934=CARTESIAN_POINT ( 'NONE',  ( -54.05457638071479920, -135.0000000000000284, 4.837889621885112845 ) ) ;
#52942=DIRECTION ( 'NONE',  ( -0.6485228581062915110, 0.000000000000000000, -0.7611951803011149931 ) ) ;
#52955=CARTESIAN_POINT ( 'NONE',  ( -57.19623071787017210, -130.3750000013656631, 4.297418129356382899 ) ) ;
#52956=CARTESIAN_POINT ( 'NONE',  ( -55.35523342533222291, -148.3125000013656063, 4.444560631937231499 ) ) ;
#52968=CARTESIAN_POINT ( 'NONE',  ( -48.00000000000002132, -155.0000000000000284, -4.041451884327376121 ) ) ;
#52986=CARTESIAN_POINT ( 'NONE',  ( -52.10840900171896806, -149.4375000013656063, 3.393966926194110556 ) ) ;
#52990=CARTESIAN_POINT ( 'NONE',  ( -57.19623071787016499, -136.3750000013656063, 4.297418129356382899 ) ) ;
#52995=ORIENTED_EDGE ( 'NONE', *, *, #37409, .T. ) ;
#52996=CARTESIAN_POINT ( 'NONE',  ( -60.14911071818854538, -145.0625000000000284, 1.666127454062681368 ) ) ;
#53005=CARTESIAN_POINT ( 'NONE',  ( -53.51423613279429503, -148.5000000013655779, 4.591703134518083651 ) ) ;
#53006=CARTESIAN_POINT ( 'NONE',  ( -56.66612745406270335, -137.4375000027312410, -5.149110718188516067 ) ) ;
#53008=LINE ( 'NONE', #8948, #10650 ) ;
#53016=CARTESIAN_POINT ( 'NONE',  ( -57.19623071787017210, -134.3750000013656347, 4.297418129356382899 ) ) ;
#53035=CARTESIAN_POINT ( 'NONE',  ( -57.19623071787017210, -143.3750000013656063, 4.297418129356382899 ) ) ;
#53073=CARTESIAN_POINT ( 'NONE',  ( -51.60603307380591787, -130.1875000013656063, -2.891590998281053704 ) ) ;
#53080=EDGE_CURVE ( 'NONE', #13129, #33278, #48270, .T. ) ;
#53088=CARTESIAN_POINT ( 'NONE',  ( -51.19402409849444524, -151.6250000027312126, -3.242614290531456334 ) ) ;
#53092=ADVANCED_FACE ( 'NONE', ( #44071 ), #1784, .F. ) ;
#53116=AXIS2_PLACEMENT_3D ( 'NONE', #27225, #7934, #47470 ) ;
#53124=CARTESIAN_POINT ( 'NONE',  ( -59.59170313451811296, -135.7500000013656063, 1.485763867205729394 ) ) ;
#53133=CARTESIAN_POINT ( 'NONE',  ( -58.51875683073618717, -135.0000000000000000, -2.985197606355836086 ) ) ;
#53153=CARTESIAN_POINT ( 'NONE',  ( -50.55543936806279248, -141.3125000013656063, 0.3552334253322060320 ) ) ;
#53161=CARTESIAN_POINT ( 'NONE',  ( -50.01589407740564042, -150.6250000000000284, 0.3983568153799778022 ) ) ;
#53174=CARTESIAN_POINT ( 'NONE',  ( -50.70258187064364108, -146.1250000013656063, 2.196230717870141014 ) ) ;
#53199=CARTESIAN_POINT ( 'NONE',  ( -56.48576386720575471, -147.0000000013655779, -4.591703134518078322 ) ) ;
#53236=UNCERTAINTY_MEASURE_WITH_UNIT (LENGTH_MEASURE( 1.000000000000000082E-05 ), #32118, 'distance_accuracy_value', 'NONE');
#53237=CARTESIAN_POINT ( 'NONE',  ( -51.75738570946856498, -153.7500000000000284, 3.805975901505576964 ) ) ;
#53238=CARTESIAN_POINT ( 'NONE',  ( -59.98410592259440222, -133.1250000000000284, -0.3983568153799752487 ) ) ;
#53247=CARTESIAN_POINT ( 'NONE',  ( -59.81910112700025905, -125.3125000027312552, -2.462841084822630311 ) ) ;
#53249=CARTESIAN_POINT ( 'NONE',  ( -53.86834273333172973, -135.0000000000000284, 4.786490365525540192 ) ) ;
#53271=CARTESIAN_POINT ( 'NONE',  ( -57.89159099828107458, -130.6875000013656063, -3.393966926194107447 ) ) ;
#53272=CARTESIAN_POINT ( 'NONE',  ( -53.51423613279429503, -146.2500000013656347, 4.591703134518083651 ) ) ;
#53279=ORIENTED_EDGE ( 'NONE', *, *, #37432, .T. ) ;
#53281=CARTESIAN_POINT ( 'NONE',  ( -57.89159099828107458, -124.9375000013656063, -3.393966926194107447 ) ) ;
#53305=CARTESIAN_POINT ( 'NONE',  ( -59.29741812935640155, -152.8750000013656063, -2.196230717870135685 ) ) ;
#53314=CARTESIAN_POINT ( 'NONE',  ( -52.53715891517739323, -145.4375000000000284, -4.819101127000233298 ) ) ;
#53322=CARTESIAN_POINT ( 'NONE',  ( -59.81910112700024484, -135.3125000027312126, -2.462841084822808835 ) ) ;
#53324=CARTESIAN_POINT ( 'NONE',  ( -50.70258187064364108, -152.3750000013656063, 2.196230717870141014 ) ) ;
#53325=CARTESIAN_POINT ( 'NONE',  ( -53.33387254593733928, -139.9375000027311842, 5.149110718188519620 ) ) ;
#53333=CARTESIAN_POINT ( 'NONE',  ( -59.59170313451811296, -131.5000000013656347, 1.485763867205729394 ) ) ;
#53347=CARTESIAN_POINT ( 'NONE',  ( -59.29741812935640155, -143.6250000013655779, -2.196230717870135685 ) ) ;
#53381=CARTESIAN_POINT ( 'NONE',  ( -51.60603307380591787, -152.9375000013656063, -2.891590998281053704 ) ) ;
#53389=VECTOR ( 'NONE', #10097, 1000.000000000000000 ) ;
#53390=CARTESIAN_POINT ( 'NONE',  ( -58.39396692619412477, -128.6875000013656063, 2.891590998281057701 ) ) ;
#53398=CARTESIAN_POINT ( 'NONE',  ( -60.14911071818854538, -152.0625000000000000, 1.666127454062681146 ) ) ;
#53399=CARTESIAN_POINT ( 'NONE',  ( -53.33387254593733928, -151.9375000027312126, 5.149110718188519620 ) ) ;
#53405=FACE_OUTER_BOUND ( 'NONE', #17497, .T. ) ;
#53413=CARTESIAN_POINT ( 'NONE',  ( -51.75738570946856498, -142.7500000000000284, 3.805975901505576964 ) ) ;
#53414=DIRECTION ( 'NONE',  ( 0.000000000000000000, 1.000000000000000000, 0.000000000000000000 ) ) ;
#53418=CARTESIAN_POINT ( 'NONE',  ( -57.89159099828107458, -152.6875000013656063, -3.393966926194107447 ) ) ;
#53431=VECTOR ( 'NONE', #4090, 1000.000000000000000 ) ;
#53435=CARTESIAN_POINT ( 'NONE',  ( -57.19623071787017210, -136.6250000013655779, 4.297418129356382899 ) ) ;
#53441=CARTESIAN_POINT ( 'NONE',  ( -51.75738570946856498, -139.7500000000000000, 3.805975901505576964 ) ) ;
#53465=CARTESIAN_POINT ( 'NONE',  ( -56.48576386720575471, -139.0000000013655779, -4.591703134518078322 ) ) ;
#53476=CARTESIAN_POINT ( 'NONE',  ( -57.46284108482265651, -143.0625000027312126, 4.819101127000238627 ) ) ;
#53485=CARTESIAN_POINT ( 'NONE',  ( -50.40829686548195099, -146.0000000013656347, -1.485763867205728284 ) ) ;
#53495=CARTESIAN_POINT ( 'NONE',  ( -58.24261429053147765, -142.3750000027312126, -3.805975901505573855 ) ) ;
#53503=LINE ( 'NONE', #18146, #14532 ) ;
#53509=CARTESIAN_POINT ( 'NONE',  ( -59.59170313451811296, -149.7500000013656063, 1.485763867205729394 ) ) ;
#53523=CARTESIAN_POINT ( 'NONE',  ( -53.33387254593710480, -140.8125000000000284, 5.149110718188539160 ) ) ;
#53538=CARTESIAN_POINT ( 'NONE',  ( -49.85088928181150436, -135.5625000000000000, -1.666127454062680480 ) ) ;
#53545=EDGE_LOOP ( 'NONE', ( #3162, #52669, #14740, #36593 ) ) ;
#53552=CARTESIAN_POINT ( 'NONE',  ( -60.14911071818854538, -132.0625000000000284, 1.666127454062681368 ) ) ;
#53560=CARTESIAN_POINT ( 'NONE',  ( -56.66612745406270335, -128.4375000027312410, -5.149110718188516067 ) ) ;
#53562=CARTESIAN_POINT ( 'NONE',  ( -50.45345700379804299, -135.0000000000000000, -0.05411738794798071767 ) ) ;
#53585=CARTESIAN_POINT ( 'NONE',  ( -54.64476657466781973, -128.8125000013656063, -4.444560631937228834 ) ) ;
#53586=CARTESIAN_POINT ( 'NONE',  ( -52.80376928212989185, -144.8750000013656063, -4.297418129356378458 ) ) ;
#53597=CARTESIAN_POINT ( 'NONE',  ( -52.10840900171896806, -125.4375000013656063, 3.393966926194110556 ) ) ;
#53609=EDGE_CURVE ( 'NONE', #19205, #36935, #21217, .T. ) ;
#53621=CARTESIAN_POINT ( 'NONE',  ( -51.60603307380591787, -150.1875000013656063, -2.891590998281053704 ) ) ;
#53631=CARTESIAN_POINT ( 'NONE',  ( -55.39835681537999790, -145.8750000000000284, 4.984105922594378235 ) ) ;
#53637=CARTESIAN_POINT ( 'NONE',  ( -59.44456063193725015, -144.8125000013656063, -0.3552334253322034230 ) ) ;
#53638=CARTESIAN_POINT ( 'NONE',  ( -56.66612745406270335, -140.4375000027312410, -5.149110718188516067 ) ) ;
#53647=CARTESIAN_POINT ( 'NONE',  ( -49.85088928181150436, -139.6875000027311842, -1.666127454062680480 ) ) ;
#53648=CARTESIAN_POINT ( 'NONE',  ( -57.89159099828107458, -132.6875000013656063, -3.393966926194107447 ) ) ;
#53651=CARTESIAN_POINT ( 'NONE',  ( -54.60164318462004474, -146.5000000027312126, -4.984105922594373794 ) ) ;
#53659=CARTESIAN_POINT ( 'NONE',  ( -50.18089887299977647, -143.8125000027311842, 2.462841084822486426 ) ) ;
#53663=CARTESIAN_POINT ( 'NONE',  ( -50.40829686548195099, -142.0000000013656063, -1.485763867205728284 ) ) ;
#53668=CARTESIAN_POINT ( 'NONE',  ( -58.59997141384986463, -154.2812500020484379, 3.067102644406258793 ) ) ;
#53677=CARTESIAN_POINT ( 'NONE',  ( -59.98410592259440222, -153.2500000027312410, -0.3983568153799752487 ) ) ;
#53694=CARTESIAN_POINT ( 'NONE',  ( -51.75738570946856498, -155.0000000000000284, 3.805975901505577408 ) ) ;
#53697=DIRECTION ( 'NONE',  ( 0.000000000000000000, 1.000000000000000000, 0.000000000000000000 ) ) ;
#53704=CARTESIAN_POINT ( 'NONE',  ( -56.48576386720575471, -129.0000000013656063, -4.591703134518078322 ) ) ;
#53707=CARTESIAN_POINT ( 'NONE',  ( -51.19402409849444524, -136.6250000027312410, -3.242614290531456334 ) ) ;
#53714=CARTESIAN_POINT ( 'NONE',  ( -59.98410592259440222, -149.2500000027312126, -0.3983568153799752487 ) ) ;
#53740=( NAMED_UNIT ( * ) SI_UNIT ( $, .STERADIAN. ) SOLID_ANGLE_UNIT ( ) );
#53751=CARTESIAN_POINT ( 'NONE',  ( -58.80597590150559739, -140.0000000000000284, 3.242614290531460330 ) ) ;
#53753=ORIENTED_EDGE ( 'NONE', *, *, #37346, .F. ) ;
#53775=CARTESIAN_POINT ( 'NONE',  ( -59.29741812935640155, -137.8750000013655779, -2.196230717870135685 ) ) ;
#53782=CARTESIAN_POINT ( 'NONE',  ( -54.60164318462004474, -150.3750000000000284, -4.984105922594373794 ) ) ;
#53794=CARTESIAN_POINT ( 'NONE',  ( -50.55543936806279248, -144.0625000013656063, 0.3552334253322060320 ) ) ;
#53821=CARTESIAN_POINT ( 'NONE',  ( -56.48576386720575471, -143.0000000013655779, -4.591703134518078322 ) ) ;
#53826=CARTESIAN_POINT ( 'NONE',  ( -59.81910112700027327, -136.3125000027311273, -2.462841084822392279 ) ) ;
#53827=CARTESIAN_POINT ( 'NONE',  ( -58.24261429053147765, -155.0000000000000284, -3.805975901505573411 ) ) ;
#53840=EDGE_CURVE ( 'NONE', #59502, #38280, #28058, .T. ) ;
#53858=CARTESIAN_POINT ( 'NONE',  ( -51.75738570946856498, -134.7500000000000284, 3.805975901505576964 ) ) ;
#53862=ORIENTED_EDGE ( 'NONE', *, *, #23718, .F. ) ;
#53868=CARTESIAN_POINT ( 'NONE',  ( -50.18089887299978358, -149.6875000000000284, 2.462841084822545934 ) ) ;
#53871=CARTESIAN_POINT ( 'NONE',  ( -59.81910112700025905, -128.3125000027312410, -2.462841084822630311 ) ) ;
#53873=CARTESIAN_POINT ( 'NONE',  ( -55.00774582457342632, -134.9999999999999716, 4.994863783263385315 ) ) ;
#53876=CARTESIAN_POINT ( 'NONE',  ( -55.39835681537999790, -145.8750000000000284, 4.984105922594378235 ) ) ;
#53896=CARTESIAN_POINT ( 'NONE',  ( -59.59170313451811296, -124.5000000013656063, 1.485763867205729394 ) ) ;
#53897=CARTESIAN_POINT ( 'NONE',  ( -59.29741812935640155, -146.6250000013656063, -2.196230717870135685 ) ) ;
#53907=CARTESIAN_POINT ( 'NONE',  ( -52.80376928212989185, -125.1250000013656205, -4.297418129356379346 ) ) ;
#53909=CARTESIAN_POINT ( 'NONE',  ( -58.24261429053147765, -155.0000000000000284, -3.805975901505573411 ) ) ;
#53929=CARTESIAN_POINT ( 'NONE',  ( -52.80376928212989185, -152.1250000013656063, -4.297418129356379346 ) ) ;
#53939=CARTESIAN_POINT ( 'NONE',  ( -56.66612745406270335, -146.3125000000000000, -5.149110718188516067 ) ) ;
#53949=CARTESIAN_POINT ( 'NONE',  ( -54.64476657466781973, -146.0625000013656063, -4.444560631937228834 ) ) ;
#53950=CARTESIAN_POINT ( 'NONE',  ( -54.60164318462004474, -139.5000000027312126, -4.984105922594373794 ) ) ;
#53953=LINE ( 'NONE', #25647, #40403 ) ;
#53962=CARTESIAN_POINT ( 'NONE',  ( -57.19623071787017210, -133.3750000013656063, 4.297418129356382899 ) ) ;
#53966=CARTESIAN_POINT ( 'NONE',  ( -51.75738570946856498, -146.8750000027312126, 3.805975901505576964 ) ) ;
#53980=CARTESIAN_POINT ( 'NONE',  ( -50.55543936806279248, -140.0625000013656063, 0.3552334253322060320 ) ) ;
#53998=CARTESIAN_POINT ( 'NONE',  ( -51.75738570946856498, -145.7500000000000284, 3.805975901505576964 ) ) ;
#54016=CARTESIAN_POINT ( 'NONE',  ( -55.00000000000002132, -155.0000000000000284, 1.734723475976807094E-15 ) ) ;
#54017=CARTESIAN_POINT ( 'NONE',  ( -59.29741812935640155, -125.8750000013656063, -2.196230717870135685 ) ) ;
#54023=DIRECTION ( 'NONE',  ( 0.000000000000000000, 1.000000000000000000, 0.000000000000000000 ) ) ;
#54027=CARTESIAN_POINT ( 'NONE',  ( -51.75738570946856498, -148.8750000027312126, 3.805975901505576964 ) ) ;
#54046=CARTESIAN_POINT ( 'NONE',  ( -52.80376928212989185, -152.8750000013656063, -4.297418129356379346 ) ) ;
#54069=CARTESIAN_POINT ( 'NONE',  ( -59.47615784096000624, -135.0000000000000284, 2.064375355545259527 ) ) ;
#54092=CARTESIAN_POINT ( 'NONE',  ( -57.89159099828107458, -138.9375000013656063, -3.393966926194107447 ) ) ;
#54099=CARTESIAN_POINT ( 'NONE',  ( -52.53715891517739323, -150.4375000000000000, -4.819101127000233298 ) ) ;
#54110=CARTESIAN_POINT ( 'NONE',  ( -58.39396692619412477, -140.4375000013656063, 2.891590998281057701 ) ) ;
#54136=CARTESIAN_POINT ( 'NONE',  ( -59.59170313451811296, -144.7500000013656063, 1.485763867205729394 ) ) ;
#54138=DIRECTION ( 'NONE',  ( 0.000000000000000000, 1.000000000000000000, 0.000000000000000000 ) ) ;
#54161=VECTOR ( 'NONE', #59018, 1000.000000000000000 ) ;
#54179=CARTESIAN_POINT ( 'NONE',  ( -57.46284108482265651, -132.9375000000000284, 4.819101127000239515 ) ) ;
#54186=CARTESIAN_POINT ( 'NONE',  ( -49.85088928181150436, -149.5625000000000284, -1.666127454062680480 ) ) ;
#54189=CARTESIAN_POINT ( 'NONE',  ( -50.55543936806279248, -152.0625000013656063, 0.3552334253322060320 ) ) ;
#54191=CARTESIAN_POINT ( 'NONE',  ( -52.79662235349376687, -135.0000000000000000, 4.334898500269361854 ) ) ;
#54206=VECTOR ( 'NONE', #6290, 1000.000000000000000 ) ;
#54211=VECTOR ( 'NONE', #21825, 1000.000000000000227 ) ;
#54215=CARTESIAN_POINT ( 'NONE',  ( -52.80376928212989185, -125.8750000013656063, -4.297418129356379346 ) ) ;
#54216=CARTESIAN_POINT ( 'NONE',  ( -59.59170313451810586, -146.5000000013656347, 1.485763867205729394 ) ) ;
#54248=CARTESIAN_POINT ( 'NONE',  ( -50.40829686548195099, -146.2500000013656063, -1.485763867205728284 ) ) ;
#54250=EDGE_CURVE ( 'NONE', #32199, #34010, #27407, .T. ) ;
#54254=LINE ( 'NONE', #60048, #1167 ) ;
#54260=CARTESIAN_POINT ( 'NONE',  ( -57.46284108482265651, -143.9375000000000000, 4.819101127000239515 ) ) ;
#54261=AXIS2_PLACEMENT_3D ( 'NONE', #54717, #39265, #30250 ) ;
#54269=CARTESIAN_POINT ( 'NONE',  ( -50.55543936806279248, -146.3125000013656063, 0.3552334253322060320 ) ) ;
#54271=CARTESIAN_POINT ( 'NONE',  ( -54.60164318462004474, -137.5000000027312126, -4.984105922594373794 ) ) ;
#54278=EDGE_LOOP ( 'NONE', ( #20809, #40730, #59487 ) ) ;
#54283=CARTESIAN_POINT ( 'NONE',  ( -59.29741812935640155, -132.6250000013656347, -2.196230717870135685 ) ) ;
#54298=CARTESIAN_POINT ( 'NONE',  ( -57.89159099828107458, -138.6875000013656347, -3.393966926194107447 ) ) ;
#54323=EDGE_CURVE ( 'NONE', #59704, #26446, #40825, .T. ) ;
#54335=LINE ( 'NONE', #9003, #52858 ) ;
#54339=CARTESIAN_POINT ( 'NONE',  ( -52.80376928212989185, -149.8750000013655779, -4.297418129356378458 ) ) ;
#54341=EDGE_CURVE ( 'NONE', #49592, #51345, #5896, .T. ) ;
#54349=CARTESIAN_POINT ( 'NONE',  ( -54.64476657466781973, -129.0625000013656063, -4.444560631937228834 ) ) ;
#54355=CARTESIAN_POINT ( 'NONE',  ( -53.33387254593725402, -149.8125000000000000, 5.149110718188524949 ) ) ;
#54357=DIRECTION ( 'NONE',  ( 0.000000000000000000, 1.000000000000000000, 0.000000000000000000 ) ) ;
#54359=CARTESIAN_POINT ( 'NONE',  ( -58.80597590150559739, -151.1250000027312126, 3.242614290531460330 ) ) ;
#54360=CIRCLE ( 'NONE', #47205, 5.000000000000000000 ) ;
#54373=VERTEX_POINT ( 'NONE', #19330 ) ;
#54380=CARTESIAN_POINT ( 'NONE',  ( -50.70258187064364108, -150.1250000013656063, 2.196230717870141014 ) ) ;
#54401=CARTESIAN_POINT ( 'NONE',  ( -58.89445808962354079, -135.0000000000000000, -2.539947039722357580 ) ) ;
#54425=CARTESIAN_POINT ( 'NONE',  ( -55.35523342533222291, -138.5625000013656063, 4.444560631937231499 ) ) ;
#54436=CARTESIAN_POINT ( 'NONE',  ( -49.85088928181150436, -140.5625000000000284, -1.666127454062680480 ) ) ;
#54445=CARTESIAN_POINT ( 'NONE',  ( -55.35523342533222291, -140.3125000013656063, 4.444560631937231499 ) ) ;
#54460=FACE_OUTER_BOUND ( 'NONE', #15513, .T. ) ;
#54471=CARTESIAN_POINT ( 'NONE',  ( -59.59170313451811296, -143.7500000013656063, 1.485763867205729394 ) ) ;
#54472=DIRECTION ( 'NONE',  ( 0.000000000000000000, 1.000000000000000000, 0.000000000000000000 ) ) ;
#54492=CARTESIAN_POINT ( 'NONE',  ( -50.01589407740564042, -144.7500000027312126, 0.3983568153799778022 ) ) ;
#54497=CARTESIAN_POINT ( 'NONE',  ( -50.18089887299980489, -135.8125000027311557, 2.462841084822814164 ) ) ;
#54503=CARTESIAN_POINT ( 'NONE',  ( -56.66612745406293783, -137.3125000000000000, -5.149110718188535607 ) ) ;
#54511=CARTESIAN_POINT ( 'NONE',  ( -51.75738570946856498, -140.8750000027312126, 3.805975901505576964 ) ) ;
#54512=CARTESIAN_POINT ( 'NONE',  ( -54.60164318462004474, -128.3750000000000284, -4.984105922594373794 ) ) ;
#54519=CARTESIAN_POINT ( 'NONE',  ( -50.70258187064364108, -153.1250000013656063, 2.196230717870141014 ) ) ;
#54532=CARTESIAN_POINT ( 'NONE',  ( -58.80597590150559739, -155.0000000000000284, 3.242614290531457666 ) ) ;
#54543=CARTESIAN_POINT ( 'NONE',  ( -50.70258187064364108, -127.1250000013656205, 2.196230717870141014 ) ) ;
#54544=CARTESIAN_POINT ( 'NONE',  ( -57.19623071787016499, -142.3750000013656063, 4.297418129356382899 ) ) ;
#54585=CARTESIAN_POINT ( 'NONE',  ( -53.33387254593733928, -141.8125000000000284, 5.149110718188519620 ) ) ;
#54594=CARTESIAN_POINT ( 'NONE',  ( -54.64476657466781973, -147.0625000013656063, -4.444560631937228834 ) ) ;
#54596=CARTESIAN_POINT ( 'NONE',  ( -50.18089887299979068, -134.8125000027312126, 2.462841084822635640 ) ) ;
#54608=CARTESIAN_POINT ( 'NONE',  ( -50.55543936806279248, -130.0625000013656063, 0.3552334253322060320 ) ) ;
#54624=CARTESIAN_POINT ( 'NONE',  ( -56.48576386720575471, -136.7500000013655779, -4.591703134518078322 ) ) ;
#54632=CARTESIAN_POINT ( 'NONE',  ( -50.70258187064364108, -131.3750000013656347, 2.196230717870141014 ) ) ;
#54656=ORIENTED_EDGE ( 'NONE', *, *, #25296, .F. ) ;
#54657=CARTESIAN_POINT ( 'NONE',  ( -50.55543936806279248, -151.0625000013656063, 0.3552334253322060320 ) ) ;
#54663=DIRECTION ( 'NONE',  ( 0.000000000000000000, 1.000000000000000000, 0.000000000000000000 ) ) ;
#54664=CARTESIAN_POINT ( 'NONE',  ( -58.39396692619412477, -126.6875000013656063, 2.891590998281057701 ) ) ;
#54674=CARTESIAN_POINT ( 'NONE',  ( -50.18089887299979068, -146.8125000027311842, 2.462841084822635640 ) ) ;
#54695=CARTESIAN_POINT ( 'NONE',  ( -50.18089887299977647, -143.6875000000000284, 2.462841084822486426 ) ) ;
#54698=CARTESIAN_POINT ( 'NONE',  ( -59.29741812935640155, -148.6250000013656063, -2.196230717870135685 ) ) ;
#54711=CARTESIAN_POINT ( 'NONE',  ( -51.75738570946856498, -142.7500000000000284, 3.805975901505576964 ) ) ;
#54717=CARTESIAN_POINT ( 'NONE',  ( -55.00000000000002132, -155.0000000000000284, 1.734723475976807094E-15 ) ) ;
#54718=CARTESIAN_POINT ( 'NONE',  ( -51.75738570946856498, -151.8750000027312126, 3.805975901505576964 ) ) ;
#54730=CARTESIAN_POINT ( 'NONE',  ( -49.85088928181150436, -147.6875000027312126, -1.666127454062680480 ) ) ;
#54746=CARTESIAN_POINT ( 'NONE',  ( -57.19623071787017210, -140.6250000013656063, 4.297418129356382899 ) ) ;
#54748=VERTEX_POINT ( 'NONE', #32802 ) ;
#54754=CARTESIAN_POINT ( 'NONE',  ( -56.66612745406293783, -140.3125000000000000, -5.149110718188535607 ) ) ;
#54763=CARTESIAN_POINT ( 'NONE',  ( -53.51423613279429503, -142.2500000013656063, 4.591703134518082763 ) ) ;
#54789=CARTESIAN_POINT ( 'NONE',  ( -56.48576386720575471, -145.0000000013656063, -4.591703134518078322 ) ) ;
#54790=VECTOR ( 'NONE', #5866, 1000.000000000000000 ) ;
#54823=CARTESIAN_POINT ( 'NONE',  ( -50.01589407740564042, -141.6250000000000284, 0.3983568153799778022 ) ) ;
#54828=CARTESIAN_POINT ( 'NONE',  ( -50.01589407740564042, -130.6250000000000284, 0.3983568153799778022 ) ) ;
#54837=CARTESIAN_POINT ( 'NONE',  ( -59.59170313451811296, -151.5000000013655779, 1.485763867205729394 ) ) ;
#54856=ORIENTED_EDGE ( 'NONE', *, *, #37346, .T. ) ;
#54861=CARTESIAN_POINT ( 'NONE',  ( -57.89159099828107458, -124.6875000013656063, -3.393966926194107447 ) ) ;
#54862=CARTESIAN_POINT ( 'NONE',  ( -59.59170313451810586, -142.5000000013656063, 1.485763867205729394 ) ) ;
#54902=CARTESIAN_POINT ( 'NONE',  ( -51.19402409849444524, -140.5000000000000000, -3.242614290531456334 ) ) ;
#54911=CARTESIAN_POINT ( 'NONE',  ( -52.80376928212989185, -148.1250000013656063, -4.297418129356378458 ) ) ;
#54913=CARTESIAN_POINT ( 'NONE',  ( -58.24261429053147765, -136.3750000027312126, -3.805975901505573855 ) ) ;
#54927=CARTESIAN_POINT ( 'NONE',  ( -59.29741812935640155, -127.6250000013656205, -2.196230717870135685 ) ) ;
#54942=CARTESIAN_POINT ( 'NONE',  ( -57.89159099828107458, -137.6875000013656063, -3.393966926194107447 ) ) ;
#54950=CARTESIAN_POINT ( 'NONE',  ( -56.48576386720575471, -133.0000000013656063, -4.591703134518078322 ) ) ;
#54955=CARTESIAN_POINT ( 'NONE',  ( -51.75738570946856498, -152.8750000027312126, 3.805975901505576964 ) ) ;
#54975=CARTESIAN_POINT ( 'NONE',  ( -53.51423613279429503, -150.2500000013656347, 4.591703134518083651 ) ) ;
#54982=CARTESIAN_POINT ( 'NONE',  ( -55.39835681537999790, -154.8750000000000284, 4.984105922594378235 ) ) ;
#54994=CARTESIAN_POINT ( 'NONE',  ( -54.60164318462004474, -147.5000000027312126, -4.984105922594373794 ) ) ;
#55011=VECTOR ( 'NONE', #38135, 1000.000000000000000 ) ;
#55013=CARTESIAN_POINT ( 'NONE',  ( -57.89159099828107458, -151.6875000013656063, -3.393966926194107447 ) ) ;
#55037=ORIENTED_EDGE ( 'NONE', *, *, #42935, .T. ) ;
#55050=ORIENTED_EDGE ( 'NONE', *, *, #54341, .F. ) ;
#55051=CARTESIAN_POINT ( 'NONE',  ( -51.75738570946856498, -155.0000000000000284, 3.805975901505577408 ) ) ;
#55055=CARTESIAN_POINT ( 'NONE',  ( -58.24261429053147765, -141.3750000027312126, -3.805975901505573855 ) ) ;
#55062=CARTESIAN_POINT ( 'NONE',  ( -54.64476657466781973, -134.0625000013656063, -4.444560631937228834 ) ) ;
#55081=CARTESIAN_POINT ( 'NONE',  ( -50.40829686548195099, -143.0000000013655779, -1.485763867205728284 ) ) ;
#55107=CARTESIAN_POINT ( 'NONE',  ( -55.35523342533222291, -142.5625000013656063, 4.444560631937231499 ) ) ;
#55120=( BOUNDED_CURVE ( )  B_SPLINE_CURVE ( 2, ( #46434, #27129, #26814, #6883, #41909, #36460, #51581, #26496, #52206 ),
 .UNSPECIFIED., .F., .F. ) 
 B_SPLINE_CURVE_WITH_KNOTS ( ( 3, 2, 2, 2, 3 ),
 ( 0.5250000000000004663, 0.5291666666666671182, 0.5333333333333338810, 0.5375000000000005329, 0.5416666666666671848 ),
 .UNSPECIFIED. ) 
 CURVE ( )  GEOMETRIC_REPRESENTATION_ITEM ( )  RATIONAL_B_SPLINE_CURVE ( ( 0.9999999999999918954, 0.9238795325112948431, 1.000000000000000000, 0.9238795325112867385, 1.000000000000000000, 0.9238795325112867385, 1.000000000000000000, 0.9238795325112766355, 1.000000000000010214 ) ) 
 REPRESENTATION_ITEM ( '' )  );
#55137=ADVANCED_FACE ( 'NONE', ( #42643 ), #17585, .F. ) ;
#55141=CARTESIAN_POINT ( 'NONE',  ( -51.19402409849444524, -137.5000000000000284, -3.242614290531456334 ) ) ;
#55151=CARTESIAN_POINT ( 'NONE',  ( -51.75738570946856498, -128.7500000000000284, 3.805975901505576964 ) ) ;
#55163=CARTESIAN_POINT ( 'NONE',  ( -58.39396692619412477, -151.4375000013656063, 2.891590998281057701 ) ) ;
#55169=CARTESIAN_POINT ( 'NONE',  ( -62.00000000000001421, -155.0000000000000284, -4.041451884327373456 ) ) ;
#55174=CARTESIAN_POINT ( 'NONE',  ( -58.24261429053147765, -147.2500000000000284, -3.805975901505573855 ) ) ;
#55186=CARTESIAN_POINT ( 'NONE',  ( -55.35523342533222291, -127.3125000013655921, 4.444560631937231499 ) ) ;
#55187=CARTESIAN_POINT ( 'NONE',  ( -55.35523342533222291, -144.3125000013656063, 4.444560631937231499 ) ) ;
#55223=DIRECTION ( 'NONE',  ( 0.000000000000000000, -1.000000000000000000, 0.000000000000000000 ) ) ;
#55226=VERTEX_POINT ( 'NONE', #14866 ) ;
#55227=CARTESIAN_POINT ( 'NONE',  ( -51.75738570946856498, -141.7500000000000284, 3.805975901505576964 ) ) ;
#55236=ORIENTED_EDGE ( 'NONE', *, *, #45234, .F. ) ;
#55238=CARTESIAN_POINT ( 'NONE',  ( -52.80376928212989185, -142.1250000013656063, -4.297418129356378458 ) ) ;
#55240=CARTESIAN_POINT ( 'NONE',  ( -56.66612745406270335, -135.4375000027312410, -5.149110718188516067 ) ) ;
#55255=CARTESIAN_POINT ( 'NONE',  ( -56.48576386720575471, -129.7500000013656063, -4.591703134518078322 ) ) ;
#55270=CARTESIAN_POINT ( 'NONE',  ( -56.48576386720575471, -137.7500000013656063, -4.591703134518078322 ) ) ;
#55281=CARTESIAN_POINT ( 'NONE',  ( -52.80376928212989185, -132.1250000013656347, -4.297418129356379346 ) ) ;
#55303=ORIENTED_EDGE ( 'NONE', *, *, #56327, .F. ) ;
#55308=CARTESIAN_POINT ( 'NONE',  ( -55.35523342533222291, -149.3125000013656063, 4.444560631937231499 ) ) ;
#55316=CARTESIAN_POINT ( 'NONE',  ( -58.80597590150559739, -152.0000000000000284, 3.242614290531460330 ) ) ;
#55326=CARTESIAN_POINT ( 'NONE',  ( -51.19402409849444524, -146.6250000027312126, -3.242614290531456334 ) ) ;
#55345=CARTESIAN_POINT ( 'NONE',  ( -59.44456063193725015, -150.5625000013656063, -0.3552334253322034230 ) ) ;
#55362=CARTESIAN_POINT ( 'NONE',  ( -53.33387254593731086, -151.9375000027312410, 5.149110718188520508 ) ) ;
#55385=CARTESIAN_POINT ( 'NONE',  ( -54.64476657466781973, -137.0625000013656063, -4.444560631937228834 ) ) ;
#55432=CARTESIAN_POINT ( 'NONE',  ( -50.70258187064364108, -141.3750000013656063, 2.196230717870141014 ) ) ;
#55459=CARTESIAN_POINT ( 'NONE',  ( -52.53715891517739323, -135.5625000027312126, -4.819101127000233298 ) ) ;
#55464=CARTESIAN_POINT ( 'NONE',  ( -53.51423613279429503, -147.5000000013656063, 4.591703134518082763 ) ) ;
#55475=CARTESIAN_POINT ( 'NONE',  ( -58.24261429053147765, -128.2500000000000284, -3.805975901505573855 ) ) ;
#55484=CARTESIAN_POINT ( 'NONE',  ( -56.66612745406270335, -124.4375000027312126, -5.149110718188516067 ) ) ;
#55498=CARTESIAN_POINT ( 'NONE',  ( -59.98410592259440222, -147.1250000000000284, -0.3983568153799752487 ) ) ;
#55512=CARTESIAN_POINT ( 'NONE',  ( -59.44456063193725015, -153.8125000013656347, -0.3552334253322034230 ) ) ;
#55513=CARTESIAN_POINT ( 'NONE',  ( -50.40829686548195099, -143.0000000013655779, -1.485763867205728284 ) ) ;
#55553=CARTESIAN_POINT ( 'NONE',  ( -54.60164318462004474, -140.3750000000000284, -4.984105922594373794 ) ) ;
#55559=CARTESIAN_POINT ( 'NONE',  ( -53.33387254593703375, -136.9375000027311557, 5.149110718188541824 ) ) ;
#55560=ORIENTED_EDGE ( 'NONE', *, *, #36683, .T. ) ;
#55561=CARTESIAN_POINT ( 'NONE',  ( -50.55543936806279248, -142.3125000013656063, 0.3552334253322060320 ) ) ;
#55564=CARTESIAN_POINT ( 'NONE',  ( -52.53715891517739323, -136.5625000027311842, -4.819101127000233298 ) ) ;
#55577=CARTESIAN_POINT ( 'NONE',  ( -54.64476657466781973, -130.8125000013656063, -4.444560631937228834 ) ) ;
#55590=CARTESIAN_POINT ( 'NONE',  ( -57.19623071787017210, -138.3750000013656063, 4.297418129356382899 ) ) ;
#55601=CARTESIAN_POINT ( 'NONE',  ( -52.80376928212989185, -131.1250000013655779, -4.297418129356379346 ) ) ;
#55611=CARTESIAN_POINT ( 'NONE',  ( -50.01589407740564042, -151.6250000000000284, 0.3983568153799778022 ) ) ;
#55623=EDGE_LOOP ( 'NONE', ( #28116, #63253, #2702, #52414 ) ) ;
#55635=CARTESIAN_POINT ( 'NONE',  ( -49.85088928181150436, -154.5625000000000000, -1.666127454062680702 ) ) ;
#55644=CARTESIAN_POINT ( 'NONE',  ( -52.10840900171896806, -152.4375000013656063, 3.393966926194110556 ) ) ;
#55646=CARTESIAN_POINT ( 'NONE',  ( -60.14911071818854538, -146.1875000027311842, 1.666127454062681368 ) ) ;
#55665=CARTESIAN_POINT ( 'NONE',  ( -51.60603307380591787, -149.9375000013656063, -2.891590998281053704 ) ) ;
#55707=CARTESIAN_POINT ( 'NONE',  ( -53.51423613279429503, -136.5000000013656347, 4.591703134518082763 ) ) ;
#55712=CARTESIAN_POINT ( 'NONE',  ( -56.37266686252615955, -135.0000000000000284, -4.242180533871957593 ) ) ;
#55744=CARTESIAN_POINT ( 'NONE',  ( -52.80376928212989185, -139.1250000013656063, -4.297418129356379346 ) ) ;
#55751=FACE_OUTER_BOUND ( 'NONE', #45344, .T. ) ;
#55764=CARTESIAN_POINT ( 'NONE',  ( -59.59170313451810586, -136.7500000013655779, 1.485763867205729394 ) ) ;
#55777=CARTESIAN_POINT ( 'NONE',  ( -56.48576386720575471, -146.0000000013656347, -4.591703134518078322 ) ) ;
#55783=VERTEX_POINT ( 'NONE', #14002 ) ;
#55788=CARTESIAN_POINT ( 'NONE',  ( -50.18089887299979068, -127.6875000000000711, 2.462841084822635640 ) ) ;
#55797=CARTESIAN_POINT ( 'NONE',  ( -56.48576386720575471, -150.7500000013655495, -4.591703134518078322 ) ) ;
#55798=CARTESIAN_POINT ( 'NONE',  ( -53.33387254593727533, -149.9375000027311842, 5.149110718188522284 ) ) ;
#55820=CARTESIAN_POINT ( 'NONE',  ( -58.39396692619412477, -152.6875000013656063, 2.891590998281057701 ) ) ;
#55821=CARTESIAN_POINT ( 'NONE',  ( -50.70258187064364108, -143.1250000013656063, 2.196230717870141014 ) ) ;
#55833=( BOUNDED_CURVE ( )  B_SPLINE_CURVE ( 2, ( #21182, #25368, #55611, #44988, #30504, #16035, #41106, #31143, #50126 ),
 .UNSPECIFIED., .F., .F. ) 
 B_SPLINE_CURVE_WITH_KNOTS ( ( 3, 2, 2, 2, 3 ),
 ( 0.1083333333333334203, 0.1125000000000000999, 0.1166666666666667657, 0.1208333333333334314, 0.1250000000000001110 ),
 .UNSPECIFIED. ) 
 CURVE ( )  GEOMETRIC_REPRESENTATION_ITEM ( )  RATIONAL_B_SPLINE_CURVE ( ( 0.9999999999999984457, 0.9238795325112882928, 1.000000000000000000, 0.9238795325112867385, 1.000000000000000000, 0.9238795325112867385, 1.000000000000000000, 0.9238795325112847401, 1.000000000000001998 ) ) 
 REPRESENTATION_ITEM ( '' )  );
#55863=CARTESIAN_POINT ( 'NONE',  ( -52.53715891517739323, -143.4375000000000284, -4.819101127000233298 ) ) ;
#55874=CARTESIAN_POINT ( 'NONE',  ( -50.40829686548195099, -144.2500000013656063, -1.485763867205728284 ) ) ;
#55876=CARTESIAN_POINT ( 'NONE',  ( -51.75738570946856498, -133.8750000027312126, 3.805975901505576964 ) ) ;
#55889=CARTESIAN_POINT ( 'NONE',  ( -58.39396692619412477, -130.4375000013656063, 2.891590998281057701 ) ) ;
#55895=CARTESIAN_POINT ( 'NONE',  ( -50.18089887299977647, -146.6875000000000000, 2.462841084822515292 ) ) ;
#55903=CARTESIAN_POINT ( 'NONE',  ( -50.70258187064364108, -133.1250000013656063, 2.196230717870141014 ) ) ;
#55912=CARTESIAN_POINT ( 'NONE',  ( -56.48576386720575471, -128.0000000013656063, -4.591703134518078322 ) ) ;
#55924=CARTESIAN_POINT ( 'NONE',  ( -60.14911071818854538, -139.1875000027312126, 1.666127454062681146 ) ) ;
#55938=CARTESIAN_POINT ( 'NONE',  ( -55.35523342533222291, -140.3125000013656063, 4.444560631937231499 ) ) ;
#55945=CARTESIAN_POINT ( 'NONE',  ( -51.75738570946856498, -152.7500000000000284, 3.805975901505576964 ) ) ;
#55954=CARTESIAN_POINT ( 'NONE',  ( -50.55543936806279248, -154.3125000013656347, 0.3552334253322060320 ) ) ;
#55956=CARTESIAN_POINT ( 'NONE',  ( -50.18089887299979068, -144.8125000027312126, 2.462841084822635640 ) ) ;
#55978=CARTESIAN_POINT ( 'NONE',  ( -50.40829686548195099, -147.0000000013655779, -1.485763867205728284 ) ) ;
#56012=ORIENTED_EDGE ( 'NONE', *, *, #25191, .F. ) ;
#56022=CARTESIAN_POINT ( 'NONE',  ( -53.51423613279429503, -134.5000000013656063, 4.591703134518082763 ) ) ;
#56039=CARTESIAN_POINT ( 'NONE',  ( -50.18089887299978358, -150.8125000027312126, 2.462841084822590787 ) ) ;
#56064=CARTESIAN_POINT ( 'NONE',  ( -59.59170313451811296, -138.7500000013656063, 1.485763867205729394 ) ) ;
#56081=CARTESIAN_POINT ( 'NONE',  ( -56.48576386720575471, -137.0000000013655779, -4.591703134518078322 ) ) ;
#56093=CARTESIAN_POINT ( 'NONE',  ( -51.60603307380591787, -147.1875000013656063, -2.891590998281053704 ) ) ;
#56108=ORIENTED_EDGE ( 'NONE', *, *, #7870, .F. ) ;
#56112=CARTESIAN_POINT ( 'NONE',  ( -50.70258187064364108, -149.1250000013656063, 2.196230717870141014 ) ) ;
#56127=CARTESIAN_POINT ( 'NONE',  ( -58.24261429053147765, -138.2500000000000000, -3.805975901505573855 ) ) ;
#56130=CARTESIAN_POINT ( 'NONE',  ( -58.24261429053147765, -140.3750000027312126, -3.805975901505573855 ) ) ;
#56132=APPLICATION_CONTEXT ( 'automotive_design' ) ;
#56136=EDGE_CURVE ( 'NONE', #56532, #11538, #40668, .T. ) ;
#56140=CARTESIAN_POINT ( 'NONE',  ( -56.48576386720575471, -151.0000000013656063, -4.591703134518078322 ) ) ;
#56144=CARTESIAN_POINT ( 'NONE',  ( -51.75738570946856498, -147.7500000000000284, 3.805975901505576964 ) ) ;
#56180=CARTESIAN_POINT ( 'NONE',  ( -60.14911071818854538, -137.0625000000000284, 1.666127454062681368 ) ) ;
#56189=CARTESIAN_POINT ( 'NONE',  ( -51.60603307380591787, -142.1875000013656063, -2.891590998281053704 ) ) ;
#56191=CARTESIAN_POINT ( 'NONE',  ( -59.98410592259440222, -129.2500000027312126, -0.3983568153799752487 ) ) ;
#56204=CARTESIAN_POINT ( 'NONE',  ( -59.98410592259440222, -142.2500000027312126, -0.3983568153799752487 ) ) ;
#56215=EDGE_CURVE ( 'NONE', #49700, #62694, #38378, .T. ) ;
#56220=CARTESIAN_POINT ( 'NONE',  ( -51.60603307380591787, -132.9375000013656063, -2.891590998281053704 ) ) ;
#56231=CARTESIAN_POINT ( 'NONE',  ( -53.51423613279429503, -127.5000000013656347, 4.591703134518082763 ) ) ;
#56254=CARTESIAN_POINT ( 'NONE',  ( -53.51423613279429503, -153.5000000013656063, 4.591703134518082763 ) ) ;
#56258=CARTESIAN_POINT ( 'NONE',  ( -50.70258187064364108, -140.1250000013656347, 2.196230717870141014 ) ) ;
#56260=CARTESIAN_POINT ( 'NONE',  ( -51.75738570946856498, -141.8750000027312126, 3.805975901505576964 ) ) ;
#56264=CARTESIAN_POINT ( 'NONE',  ( -60.14911071818854538, -151.0625000000000000, 1.666127454062681368 ) ) ;
#56274=CARTESIAN_POINT ( 'NONE',  ( -58.24261429053147765, -142.3750000027312126, -3.805975901505573855 ) ) ;
#56281=CARTESIAN_POINT ( 'NONE',  ( -59.59170313451811296, -140.5000000013656347, 1.485763867205729394 ) ) ;
#56293=CARTESIAN_POINT ( 'NONE',  ( -52.80376928212989185, -143.8750000013655779, -4.297418129356379346 ) ) ;
#56295=EDGE_CURVE ( 'NONE', #44367, #49592, #57699, .T. ) ;
#56300=CARTESIAN_POINT ( 'NONE',  ( -50.01589407740564042, -141.7500000027312126, 0.3983568153799778022 ) ) ;
#56327=EDGE_CURVE ( 'NONE', #14198, #52848, #14243, .T. ) ;
#56347=CARTESIAN_POINT ( 'NONE',  ( -56.48576386720575471, -134.0000000013656063, -4.591703134518078322 ) ) ;
#56388=CARTESIAN_POINT ( 'NONE',  ( -59.44456063193725015, -139.8125000013656063, -0.3552334253322034230 ) ) ;
#56395=CARTESIAN_POINT ( 'NONE',  ( -55.00000000000002132, -155.0000000000000284, 1.734723475976807094E-15 ) ) ;
#56402=( BOUNDED_CURVE ( )  B_SPLINE_CURVE ( 2, ( #38123, #48075, #4029, #53538, #8846, #23648, #13671, #19752, #5288 ),
 .UNSPECIFIED., .F., .F. ) 
 B_SPLINE_CURVE_WITH_KNOTS ( ( 3, 2, 2, 2, 3 ),
 ( 0.6416666666666662744, 0.6458333333333329263, 0.6499999999999996891, 0.6541666666666663410, 0.6583333333333329929 ),
 .UNSPECIFIED. ) 
 CURVE ( )  GEOMETRIC_REPRESENTATION_ITEM ( )  RATIONAL_B_SPLINE_CURVE ( ( 1.000000000000008216, 0.9238795325112786339, 1.000000000000000000, 0.9238795325112867385, 1.000000000000000000, 0.9238795325112867385, 1.000000000000000000, 0.9238795325112928447, 0.9999999999999938938 ) ) 
 REPRESENTATION_ITEM ( '' )  );
#56421=CARTESIAN_POINT ( 'NONE',  ( -55.35523342533222291, -146.5625000013656063, 4.444560631937231499 ) ) ;
#56426=ORIENTED_EDGE ( 'NONE', *, *, #26357, .T. ) ;
#56429=DIRECTION ( 'NONE',  ( 0.000000000000000000, 1.000000000000000000, 0.000000000000000000 ) ) ;
#56433=CARTESIAN_POINT ( 'NONE',  ( -52.53715891517739323, -125.4375000000000284, -4.819101127000233298 ) ) ;
#56440=CARTESIAN_POINT ( 'NONE',  ( -57.89159099828107458, -147.6875000013656063, -3.393966926194107447 ) ) ;
#56465=CARTESIAN_POINT ( 'NONE',  ( -54.64476657466781973, -152.0625000013656063, -4.444560631937228834 ) ) ;
#56472=CARTESIAN_POINT ( 'NONE',  ( -51.75738570946856498, -137.8750000027312126, 3.805975901505576964 ) ) ;
#56485=CYLINDRICAL_SURFACE ( 'NONE', #8821, 5.000000000000000000 ) ;
#56502=CARTESIAN_POINT ( 'NONE',  ( -59.81910112700025905, -137.1875000000000000, -2.462841084822630311 ) ) ;
#56512=CARTESIAN_POINT ( 'NONE',  ( -59.29741812935640155, -141.8750000013655779, -2.196230717870135685 ) ) ;
#56514=CARTESIAN_POINT ( 'NONE',  ( -52.53715891517739323, -130.5625000027311842, -4.819101127000233298 ) ) ;
#56527=CARTESIAN_POINT ( 'NONE',  ( -50.40829686548195099, -126.0000000013656063, -1.485763867205728284 ) ) ;
#56532=VERTEX_POINT ( 'NONE', #10374 ) ;
#56540=CARTESIAN_POINT ( 'NONE',  ( -58.39396692619412477, -135.4375000013656063, 2.891590998281057701 ) ) ;
#56550=CARTESIAN_POINT ( 'NONE',  ( -59.29741812935640155, -127.8750000013656063, -2.196230717870135685 ) ) ;
#56563=CARTESIAN_POINT ( 'NONE',  ( -57.46284108482265651, -139.0625000027312126, 4.819101127000238627 ) ) ;
#56575=CARTESIAN_POINT ( 'NONE',  ( -52.80376928212989185, -139.8750000013655779, -4.297418129356378458 ) ) ;
#56582=CARTESIAN_POINT ( 'NONE',  ( -58.24261429053147765, -148.2500000000000284, -3.805975901505573855 ) ) ;
#56583=EDGE_CURVE ( 'NONE', #52748, #59502, #27308, .T. ) ;
#56592=CARTESIAN_POINT ( 'NONE',  ( -53.51423613279429503, -153.5000000013656063, 4.591703134518083651 ) ) ;
#56593=CARTESIAN_POINT ( 'NONE',  ( -53.33387254593733928, -142.9375000027312410, 5.149110718188519620 ) ) ;
#56603=CARTESIAN_POINT ( 'NONE',  ( -51.60603307380591787, -137.9375000013656063, -2.891590998281053704 ) ) ;
#56618=CARTESIAN_POINT ( 'NONE',  ( -55.35523342533222291, -145.3125000013656063, 4.444560631937231499 ) ) ;
#56646=CARTESIAN_POINT ( 'NONE',  ( -58.59997141384986463, -154.8437500006828031, 3.067102644406258793 ) ) ;
#56660=CARTESIAN_POINT ( 'NONE',  ( -59.29741812935640155, -130.8750000013656063, -2.196230717870135685 ) ) ;
#56669=CARTESIAN_POINT ( 'NONE',  ( -57.46284108482265651, -154.0625000027312126, 4.819101127000239515 ) ) ;
#56704=CARTESIAN_POINT ( 'NONE',  ( -54.64476657466781973, -141.0625000013656063, -4.444560631937228834 ) ) ;
#56722=CARTESIAN_POINT ( 'NONE',  ( -59.44456063193725015, -135.8125000013656063, -0.3552334253322034230 ) ) ;
#56734=CARTESIAN_POINT ( 'NONE',  ( -56.48576386720575471, -143.0000000013655779, -4.591703134518078322 ) ) ;
#56745=CARTESIAN_POINT ( 'NONE',  ( -51.75738570946856498, -151.7500000000000284, 3.805975901505576964 ) ) ;
#56746=CARTESIAN_POINT ( 'NONE',  ( -51.75738570946856498, -125.7500000000000284, 3.805975901505576964 ) ) ;
#56754=CARTESIAN_POINT ( 'NONE',  ( -52.80376928212989185, -150.8750000013656063, -4.297418129356379346 ) ) ;
#56766=CARTESIAN_POINT ( 'NONE',  ( -58.24261429053147765, -142.3750000027312126, -3.805975901505573855 ) ) ;
#56782=CARTESIAN_POINT ( 'NONE',  ( -53.51423613279429503, -151.5000000013655779, 4.591703134518082763 ) ) ;
#56819=CARTESIAN_POINT ( 'NONE',  ( -49.85088928181150436, -139.5625000000000284, -1.666127454062680702 ) ) ;
#56829=CARTESIAN_POINT ( 'NONE',  ( -59.29741812935640155, -139.8750000013655779, -2.196230717870135685 ) ) ;
#56831=CARTESIAN_POINT ( 'NONE',  ( -50.01589407740564042, -129.7500000027312126, 0.3983568153799778022 ) ) ;
#56836=CARTESIAN_POINT ( 'NONE',  ( -59.98410592259440222, -151.2500000027312410, -0.3983568153799752487 ) ) ;
#56854=CARTESIAN_POINT ( 'NONE',  ( -52.10840900171896806, -134.1875000013656063, 3.393966926194110556 ) ) ;
#56864=CARTESIAN_POINT ( 'NONE',  ( -59.29741812935640155, -128.8750000013656063, -2.196230717870135685 ) ) ;
#56879=CARTESIAN_POINT ( 'NONE',  ( -58.80597590150559739, -139.1250000027312410, 3.242614290531460330 ) ) ;
#56891=CARTESIAN_POINT ( 'NONE',  ( -50.55543936806279248, -137.0625000013656063, 0.3552334253322060320 ) ) ;
#56896=CARTESIAN_POINT ( 'NONE',  ( -58.24261429053147765, -149.2500000000000284, -3.805975901505573855 ) ) ;
#56906=CARTESIAN_POINT ( 'NONE',  ( -57.89159099828107458, -152.9375000013656063, -3.393966926194107447 ) ) ;
#56907=CARTESIAN_POINT ( 'NONE',  ( -50.18089887299979068, -142.8125000027311842, 2.462841084822635640 ) ) ;
#56915=CARTESIAN_POINT ( 'NONE',  ( -50.40829686548195099, -136.0000000013656063, -1.485763867205728284 ) ) ;
#56917=CARTESIAN_POINT ( 'NONE',  ( -55.00000000000002132, -155.0000000000000284, 1.734723475976807094E-15 ) ) ;
#56930=CARTESIAN_POINT ( 'NONE',  ( -57.19623071787017210, -145.3750000013656347, 4.297418129356382899 ) ) ;
#56971=( BOUNDED_CURVE ( )  B_SPLINE_CURVE ( 2, ( #41016, #1488, #60976, #32005, #31689, #36203, #11740, #50357, #61290 ),
 .UNSPECIFIED., .F., .F. ) 
 B_SPLINE_CURVE_WITH_KNOTS ( ( 3, 2, 2, 2, 3 ),
 ( 0.008333333333333340157, 0.01250000000000001110, 0.01666666666666668031, 0.02083333333333334952, 0.02500000000000002220 ),
 .UNSPECIFIED. ) 
 CURVE ( )  GEOMETRIC_REPRESENTATION_ITEM ( )  RATIONAL_B_SPLINE_CURVE ( ( 0.9999999999999998890, 0.9238795325112868495, 1.000000000000000000, 0.9238795325112867385, 1.000000000000000000, 0.9238795325112867385, 1.000000000000000000, 0.9238795325112864054, 1.000000000000000444 ) ) 
 REPRESENTATION_ITEM ( '' )  );
#56974=CARTESIAN_POINT ( 'NONE',  ( -57.89159099828107458, -129.9375000013656063, -3.393966926194107447 ) ) ;
#57002=FACE_OUTER_BOUND ( 'NONE', #61264, .T. ) ;
#57003=AXIS2_PLACEMENT_3D ( 'NONE', #54016, #30198, #34080 ) ;
#57019=CARTESIAN_POINT ( 'NONE',  ( -58.39396692619412477, -135.6875000013656063, 2.891590998281057701 ) ) ;
#57028=ORIENTED_EDGE ( 'NONE', *, *, #39005, .F. ) ;
#57036=VECTOR ( 'NONE', #16304, 1000.000000000000000 ) ;
#57054=CARTESIAN_POINT ( 'NONE',  ( -54.64476657466781973, -143.0625000013656063, -4.444560631937228834 ) ) ;
#57072=CARTESIAN_POINT ( 'NONE',  ( -57.19623071787017210, -149.3750000013656347, 4.297418129356382899 ) ) ;
#57073=CARTESIAN_POINT ( 'NONE',  ( -51.75738570946856498, -149.8750000027312126, 3.805975901505576964 ) ) ;
#57083=CARTESIAN_POINT ( 'NONE',  ( -51.19402409849444524, -140.6250000027312126, -3.242614290531456334 ) ) ;
#57095=CARTESIAN_POINT ( 'NONE',  ( -50.55543936806279248, -146.3125000013656063, 0.3552334253322060320 ) ) ;
#57138=CARTESIAN_POINT ( 'NONE',  ( -52.53715891517739323, -139.4375000000000000, -4.819101127000233298 ) ) ;
#57149=CARTESIAN_POINT ( 'NONE',  ( -57.19623071787016499, -138.6250000013656063, 4.297418129356382899 ) ) ;
#57151=CARTESIAN_POINT ( 'NONE',  ( -60.14911071818854538, -129.1875000027312126, 1.666127454062681368 ) ) ;
#57163=CARTESIAN_POINT ( 'NONE',  ( -55.39835681537999790, -153.8750000000000284, 4.984105922594378235 ) ) ;
#57174=DIRECTION ( 'NONE',  ( -0.6485228581062915110, 0.000000000000000000, -0.7611951803011149931 ) ) ;
#57175=CARTESIAN_POINT ( 'NONE',  ( -51.60603307380591787, -131.9375000013656063, -2.891590998281053704 ) ) ;
#57185=CARTESIAN_POINT ( 'NONE',  ( -57.19623071787017210, -128.6250000013656347, 4.297418129356382899 ) ) ;
#57212=CARTESIAN_POINT ( 'NONE',  ( -57.89159099828107458, -139.6875000013656063, -3.393966926194107447 ) ) ;
#57217=CARTESIAN_POINT ( 'NONE',  ( -60.14911071818854538, -148.0625000000000000, 1.666127454062681368 ) ) ;
#57226=CARTESIAN_POINT ( 'NONE',  ( -52.80376928212989185, -150.1250000013656063, -4.297418129356378458 ) ) ;
#57227=CARTESIAN_POINT ( 'NONE',  ( -55.39835681537999790, -141.0000000027312126, 4.984105922594378235 ) ) ;
#57237=CARTESIAN_POINT ( 'NONE',  ( -55.35523342533222291, -138.3125000013656063, 4.444560631937231499 ) ) ;
#57243=ORIENTED_EDGE ( 'NONE', *, *, #18804, .F. ) ;
#57252=CARTESIAN_POINT ( 'NONE',  ( -58.39396692619412477, -144.4375000013656063, 2.891590998281057701 ) ) ;
#57296=CARTESIAN_POINT ( 'NONE',  ( -51.60603307380591787, -132.1875000013656063, -2.891590998281053704 ) ) ;
#57303=CARTESIAN_POINT ( 'NONE',  ( -58.80597590150559739, -153.1250000027312126, 3.242614290531460330 ) ) ;
#57338=CARTESIAN_POINT ( 'NONE',  ( -59.29741812935640155, -135.8750000013655779, -2.196230717870135685 ) ) ;
#57366=CARTESIAN_POINT ( 'NONE',  ( -55.35523342533222291, -142.5625000013656063, 4.444560631937231499 ) ) ;
#57373=CYLINDRICAL_SURFACE ( 'NONE', #50229, 5.000000000000000000 ) ;
#57381=VERTEX_POINT ( 'NONE', #36337 ) ;
#57383=CARTESIAN_POINT ( 'NONE',  ( -51.75738570946856498, -154.7500000000000284, 3.805975901505576964 ) ) ;
#57386=CARTESIAN_POINT ( 'NONE',  ( -57.19623071787017210, -145.3750000013656347, 4.297418129356382899 ) ) ;
#57400=CARTESIAN_POINT ( 'NONE',  ( -51.75738570946856498, -140.7500000000000000, 3.805975901505576964 ) ) ;
#57413=CARTESIAN_POINT ( 'NONE',  ( -57.19623071787017210, -147.6250000013655779, 4.297418129356382899 ) ) ;
#57446=DIRECTION ( 'NONE',  ( 0.000000000000000000, 1.000000000000000000, 0.000000000000000000 ) ) ;
#57449=CARTESIAN_POINT ( 'NONE',  ( -50.18089887299979068, -136.6875000000000284, 2.462841084822635640 ) ) ;
#57462=CARTESIAN_POINT ( 'NONE',  ( -50.70258187064364108, -139.3750000013656063, 2.196230717870141014 ) ) ;
#57464=CARTESIAN_POINT ( 'NONE',  ( -59.98410592259440222, -130.2500000027312126, -0.3983568153799752487 ) ) ;
#57472=PLANE ( 'NONE',  #62505 ) ;
#57489=CARTESIAN_POINT ( 'NONE',  ( -55.00000000000002132, -155.0000000000000284, 1.734723475976807094E-15 ) ) ;
#57490=CARTESIAN_POINT ( 'NONE',  ( -50.40829686548195099, -130.0000000013656063, -1.485763867205728284 ) ) ;
#57513=ORIENTED_EDGE ( 'NONE', *, *, #37432, .F. ) ;
#57531=CARTESIAN_POINT ( 'NONE',  ( -55.39835681537999790, -147.8750000000000284, 4.984105922594378235 ) ) ;
#57540=CARTESIAN_POINT ( 'NONE',  ( -59.44456063193725015, -149.8125000013656063, -0.3552334253322034230 ) ) ;
#57541=CARTESIAN_POINT ( 'NONE',  ( -58.24261429053147765, -143.3750000027312126, -3.805975901505573855 ) ) ;
#57548=CARTESIAN_POINT ( 'NONE',  ( -50.55543936806279248, -135.0625000013656063, 0.3552334253322060320 ) ) ;
#57550=EDGE_CURVE ( 'NONE', #40253, #57381, #2708, .T. ) ;
#57566=CARTESIAN_POINT ( 'NONE',  ( -52.10840900171896806, -142.1875000013656063, 3.393966926194110556 ) ) ;
#57601=CARTESIAN_POINT ( 'NONE',  ( -55.35523342533222291, -154.3125000013656347, 4.444560631937231499 ) ) ;
#57608=CARTESIAN_POINT ( 'NONE',  ( -57.19623071787017210, -131.6250000013655779, 4.297418129356382899 ) ) ;
#57650=CARTESIAN_POINT ( 'NONE',  ( -54.64476657466781973, -137.0625000013656063, -4.444560631937228834 ) ) ;
#57681=CARTESIAN_POINT ( 'NONE',  ( -59.29741812935640155, -142.8750000013656063, -2.196230717870135685 ) ) ;
#57686=ORIENTED_EDGE ( 'NONE', *, *, #24410, .F. ) ;
#57698=CARTESIAN_POINT ( 'NONE',  ( -50.55543936806279248, -143.0625000013656063, 0.3552334253322060320 ) ) ;
#57699=LINE ( 'NONE', #13308, #36735 ) ;
#57712=CARTESIAN_POINT ( 'NONE',  ( -58.24261429053147765, -146.2500000000000284, -3.805975901505573855 ) ) ;
#57722=CARTESIAN_POINT ( 'NONE',  ( -50.70258187064364108, -149.3750000013656347, 2.196230717870141014 ) ) ;
#57761=CARTESIAN_POINT ( 'NONE',  ( -53.33387254593733928, -133.8125000000000284, 5.149110718188519620 ) ) ;
#57769=CARTESIAN_POINT ( 'NONE',  ( -59.44456063193725015, -137.8125000013656063, -0.3552334253322034230 ) ) ;
#57771=CARTESIAN_POINT ( 'NONE',  ( -59.98410592259440222, -127.2500000027312126, -0.3983568153799752487 ) ) ;
#57795=CARTESIAN_POINT ( 'NONE',  ( -52.10840900171896806, -131.1875000013656063, 3.393966926194110556 ) ) ;
#57803=ORIENTED_EDGE ( 'NONE', *, *, #61399, .F. ) ;
#57830=CARTESIAN_POINT ( 'NONE',  ( -52.80376928212989185, -150.1250000013656063, -4.297418129356379346 ) ) ;
#57835=CARTESIAN_POINT ( 'NONE',  ( -54.64476657466781973, -135.8125000013656063, -4.444560631937228834 ) ) ;
#57840=CARTESIAN_POINT ( 'NONE',  ( -59.81910112700025905, -146.1875000000000284, -2.462841084822630311 ) ) ;
#57844=( BOUNDED_CURVE ( )  B_SPLINE_CURVE ( 2, ( #63167, #62549, #19078, #24230, #38394, #19404, #13326, #43836, #14263 ),
 .UNSPECIFIED., .F., .F. ) 
 B_SPLINE_CURVE_WITH_KNOTS ( ( 3, 2, 2, 2, 3 ),
 ( 0.3583333333333336146, 0.3625000000000002665, 0.3666666666666669183, 0.3708333333333336257, 0.3750000000000002776 ),
 .UNSPECIFIED. ) 
 CURVE ( )  GEOMETRIC_REPRESENTATION_ITEM ( )  RATIONAL_B_SPLINE_CURVE ( ( 0.9999999999999948930, 0.9238795325112918455, 1.000000000000000000, 0.9238795325112867385, 1.000000000000000000, 0.9238795325112867385, 1.000000000000000000, 0.9238795325112816315, 1.000000000000005107 ) ) 
 REPRESENTATION_ITEM ( '' )  );
#57850=CARTESIAN_POINT ( 'NONE',  ( -50.55543936806279248, -149.3125000013656063, 0.3552334253322060320 ) ) ;
#57851=CARTESIAN_POINT ( 'NONE',  ( -51.19402409849444524, -139.6250000027312126, -3.242614290531456334 ) ) ;
#57852=CARTESIAN_POINT ( 'NONE',  ( -48.00000000000002132, -155.0000000000000284, 4.041451884327384114 ) ) ;
#57858=CARTESIAN_POINT ( 'NONE',  ( -50.55543936806279248, -138.0625000013656063, 0.3552334253322060320 ) ) ;
#57872=CARTESIAN_POINT ( 'NONE',  ( -56.48576386720575471, -139.7500000013656347, -4.591703134518078322 ) ) ;
#57906=CARTESIAN_POINT ( 'NONE',  ( -56.48576386720575471, -151.7500000013656063, -4.591703134518078322 ) ) ;
#57915=CARTESIAN_POINT ( 'NONE',  ( -59.44456063193725015, -131.8125000013656063, -0.3552334253322034230 ) ) ;
#57926=CARTESIAN_POINT ( 'NONE',  ( -59.81910112700025905, -150.3125000027312410, -2.462841084822630311 ) ) ;
#57945=CARTESIAN_POINT ( 'NONE',  ( -51.60603307380591787, -151.9375000013656063, -2.891590998281053704 ) ) ;
#57959=CARTESIAN_POINT ( 'NONE',  ( -59.59170313451811296, -134.7500000013656063, 1.485763867205729394 ) ) ;
#57965=CARTESIAN_POINT ( 'NONE',  ( -59.00781279294024984, -134.9999999999999432, -2.380179661103284161 ) ) ;
#57975=CARTESIAN_POINT ( 'NONE',  ( -58.80597590150559739, -144.1250000027312126, 3.242614290531460330 ) ) ;
#57985=CARTESIAN_POINT ( 'NONE',  ( -51.60603307380591787, -144.1875000013656063, -2.891590998281053704 ) ) ;
#58002=CARTESIAN_POINT ( 'NONE',  ( -57.19623071787017210, -144.3750000013656063, 4.297418129356382899 ) ) ;
#58024=CARTESIAN_POINT ( 'NONE',  ( -52.80376928212989185, -148.1250000013656063, -4.297418129356379346 ) ) ;
#58060=CARTESIAN_POINT ( 'NONE',  ( -58.80597590150559739, -132.0000000000000284, 3.242614290531460330 ) ) ;
#58063=EDGE_LOOP ( 'NONE', ( #13367, #2635, #51301, #22935 ) ) ;
#58069=CARTESIAN_POINT ( 'NONE',  ( -60.14911071818854538, -126.1875000027312410, 1.666127454062681368 ) ) ;
#58071=CARTESIAN_POINT ( 'NONE',  ( -50.55945893837505167, -135.0000000000000568, 1.298165042310468031 ) ) ;
#58077=DIRECTION ( 'NONE',  ( 0.000000000000000000, 1.000000000000000000, 0.000000000000000000 ) ) ;
#58093=CARTESIAN_POINT ( 'NONE',  ( -59.59170313451811296, -131.5000000013656347, 1.485763867205729394 ) ) ;
#58095=CARTESIAN_POINT ( 'NONE',  ( -59.44456063193725015, -145.5625000013656063, -0.3552334253322034230 ) ) ;
#58113=CARTESIAN_POINT ( 'NONE',  ( -58.24261429053147765, -137.3750000027312126, -3.805975901505573855 ) ) ;
#58128=CARTESIAN_POINT ( 'NONE',  ( -52.10840900171896806, -150.4375000013656063, 3.393966926194110556 ) ) ;
#58132=CARTESIAN_POINT ( 'NONE',  ( -59.44456063193725015, -136.5625000013656063, -0.3552334253322034230 ) ) ;
#58137=CARTESIAN_POINT ( 'NONE',  ( -50.01589407740564042, -145.6250000000000284, 0.3983568153799778022 ) ) ;
#58144=CARTESIAN_POINT ( 'NONE',  ( -55.39835672516371545, -134.9999999999999716, 4.984105929804953483 ) ) ;
#58146=CARTESIAN_POINT ( 'NONE',  ( -57.89159099828107458, -149.9375000013656063, -3.393966926194107447 ) ) ;
#58147=CARTESIAN_POINT ( 'NONE',  ( -59.81910112700025905, -140.3125000027312126, -2.462841084822630311 ) ) ;
#58155=CARTESIAN_POINT ( 'NONE',  ( -58.24261429053147765, -153.2500000000000284, -3.805975901505573855 ) ) ;
#58156=CARTESIAN_POINT ( 'NONE',  ( -57.19623071787017210, -131.3750000013656347, 4.297418129356382899 ) ) ;
#58174=CARTESIAN_POINT ( 'NONE',  ( -59.44456063193725015, -140.5625000013656063, -0.3552334253322034230 ) ) ;
#58208=CARTESIAN_POINT ( 'NONE',  ( -53.51423613279429503, -153.2500000013656063, 4.591703134518083651 ) ) ;
#58215=CARTESIAN_POINT ( 'NONE',  ( -50.40829686548195099, -127.2500000013656347, -1.485763867205728284 ) ) ;
#58226=CARTESIAN_POINT ( 'NONE',  ( -60.14911071818854538, -152.1875000027312126, 1.666127454062681368 ) ) ;
#58248=CARTESIAN_POINT ( 'NONE',  ( -54.64476657466781973, -153.8125000013656347, -4.444560631937228834 ) ) ;
#58262=EDGE_CURVE ( 'NONE', #52748, #43968, #25895, .T. ) ;
#58264=CARTESIAN_POINT ( 'NONE',  ( -50.18089887299977647, -142.6875000000000000, 2.462841084822456672 ) ) ;
#58270=CARTESIAN_POINT ( 'NONE',  ( -52.10840900171896806, -136.4375000013656063, 3.393966926194110556 ) ) ;
#58300=CARTESIAN_POINT ( 'NONE',  ( -59.44456063193725015, -138.8125000013656063, -0.3552334253322034230 ) ) ;
#58317=CARTESIAN_POINT ( 'NONE',  ( -52.80376928212989185, -144.8750000013655779, -4.297418129356379346 ) ) ;
#58341=CARTESIAN_POINT ( 'NONE',  ( -55.35523342533222291, -146.5625000013656063, 4.444560631937231499 ) ) ;
#58343=EDGE_CURVE ( 'NONE', #37814, #44139, #1795, .T. ) ;
#58353=CARTESIAN_POINT ( 'NONE',  ( -55.39835681537999790, -140.8750000000000284, 4.984105922594378235 ) ) ;
#58363=CARTESIAN_POINT ( 'NONE',  ( -51.19402409849444524, -145.6250000027312126, -3.242614290531456334 ) ) ;
#58380=CARTESIAN_POINT ( 'NONE',  ( -50.18089887299979068, -134.6875000000000000, 2.462841084822635640 ) ) ;
#58389=ORIENTED_EDGE ( 'NONE', *, *, #25646, .F. ) ;
#58391=CARTESIAN_POINT ( 'NONE',  ( -58.80597590150559739, -127.1250000027312268, 3.242614290531460330 ) ) ;
#58399=LINE ( 'NONE', #8877, #29914 ) ;
#58416=CARTESIAN_POINT ( 'NONE',  ( -50.55543936806279248, -129.0625000013656063, 0.3552334253322060320 ) ) ;
#58417=CARTESIAN_POINT ( 'NONE',  ( -50.40829686548195099, -145.0000000013656063, -1.485763867205728284 ) ) ;
#58425=ORIENTED_EDGE ( 'NONE', *, *, #34127, .T. ) ;
#58428=LINE ( 'NONE', #53909, #9041 ) ;
#58438=EDGE_LOOP ( 'NONE', ( #6351, #26480, #43405, #13999 ) ) ;
#58451=CARTESIAN_POINT ( 'NONE',  ( -59.29741812935640155, -150.8750000013656063, -2.196230717870135685 ) ) ;
#58461=CARTESIAN_POINT ( 'NONE',  ( -59.98410592259440222, -145.1250000000000284, -0.3983568153799752487 ) ) ;
#58468=CARTESIAN_POINT ( 'NONE',  ( -54.64476657466781973, -149.0625000013656063, -4.444560631937228834 ) ) ;
#58469=CARTESIAN_POINT ( 'NONE',  ( -50.01589407740564042, -137.7500000027312126, 0.3983568153799778022 ) ) ;
#58478=CARTESIAN_POINT ( 'NONE',  ( -52.53715891517739323, -139.5625000027312126, -4.819101127000233298 ) ) ;
#58479=CARTESIAN_POINT ( 'NONE',  ( -57.89159099828107458, -134.6875000013656063, -3.393966926194107447 ) ) ;
#58481=DIRECTION ( 'NONE',  ( 0.000000000000000000, 1.000000000000000000, 0.000000000000000000 ) ) ;
#58491=CARTESIAN_POINT ( 'NONE',  ( -58.24261429053147765, -143.2500000000000284, -3.805975901505573855 ) ) ;
#58496=CARTESIAN_POINT ( 'NONE',  ( -59.59170313451811296, -142.5000000013656347, 1.485763867205729394 ) ) ;
#58528=CARTESIAN_POINT ( 'NONE',  ( -59.29741812935640155, -152.6250000013656063, -2.196230717870135685 ) ) ;
#58537=CARTESIAN_POINT ( 'NONE',  ( -57.89159099828107458, -125.9375000013656063, -3.393966926194107447 ) ) ;
#58544=CARTESIAN_POINT ( 'NONE',  ( -55.00000000000002132, -155.0000000000000284, 1.734723475976807094E-15 ) ) ;
#58548=CARTESIAN_POINT ( 'NONE',  ( -50.01589407740564042, -149.7500000027312126, 0.3983568153799778022 ) ) ;
#58567=CARTESIAN_POINT ( 'NONE',  ( -53.51423613279429503, -152.2500000013656347, 4.591703134518082763 ) ) ;
#58599=ADVANCED_FACE ( 'NONE', ( #61594 ), #51310, .F. ) ;
#58613=CARTESIAN_POINT ( 'NONE',  ( -59.44456063193725015, -140.8125000013656063, -0.3552334253322034230 ) ) ;
#58618=CARTESIAN_POINT ( 'NONE',  ( -59.98410592259440222, -148.2500000027312126, -0.3983568153799752487 ) ) ;
#58632=CARTESIAN_POINT ( 'NONE',  ( -50.70258187064364108, -145.1250000013655779, 2.196230717870141014 ) ) ;
#58636=ORIENTED_EDGE ( 'NONE', *, *, #62620, .T. ) ;
#58645=DIRECTION ( 'NONE',  ( 0.000000000000000000, 1.000000000000000000, 0.000000000000000000 ) ) ;
#58654=CARTESIAN_POINT ( 'NONE',  ( -51.60603307380591787, -144.1875000013656063, -2.891590998281053704 ) ) ;
#58682=VERTEX_POINT ( 'NONE', #56127 ) ;
#58692=CARTESIAN_POINT ( 'NONE',  ( -59.98410592259440222, -132.1250000000000284, -0.3983568153799752487 ) ) ;
#58701=CARTESIAN_POINT ( 'NONE',  ( -56.66612745406270335, -125.4375000027312126, -5.149110718188516067 ) ) ;
#58706=DIRECTION ( 'NONE',  ( 0.000000000000000000, 1.000000000000000000, 0.000000000000000000 ) ) ;
#58724=CARTESIAN_POINT ( 'NONE',  ( -62.00000000000001421, -155.0000000000000284, 4.041451884327384114 ) ) ;
#58725=CARTESIAN_POINT ( 'NONE',  ( -52.10840900171896806, -129.1875000013656063, 3.393966926194110556 ) ) ;
#58726=CARTESIAN_POINT ( 'NONE',  ( -59.59170313451810586, -147.5000000013656063, 1.485763867205729394 ) ) ;
#58735=ORIENTED_EDGE ( 'NONE', *, *, #29916, .F. ) ;
#58758=CARTESIAN_POINT ( 'NONE',  ( -58.39396692619412477, -152.6875000013656063, 2.891590998281057701 ) ) ;
#58768=CARTESIAN_POINT ( 'NONE',  ( -50.18089887299979068, -144.6875000000000568, 2.462841084822635640 ) ) ;
#58775=CARTESIAN_POINT ( 'NONE',  ( -59.44456063193725015, -147.8125000013656063, -0.3552334253322034230 ) ) ;
#58776=CARTESIAN_POINT ( 'NONE',  ( -51.75738570946856498, -137.8750000027312126, 3.805975901505576964 ) ) ;
#58788=CARTESIAN_POINT ( 'NONE',  ( -52.80376928212989185, -133.8750000013656063, -4.297418129356379346 ) ) ;
#58791=CARTESIAN_POINT ( 'NONE',  ( -58.24261429053147765, -146.3750000027312126, -3.805975901505573855 ) ) ;
#58802=CARTESIAN_POINT ( 'NONE',  ( -58.39396692619412477, -140.4375000013656063, 2.891590998281057701 ) ) ;
#58836=CARTESIAN_POINT ( 'NONE',  ( -53.51423613279429503, -154.2500000013656063, 4.591703134518083651 ) ) ;
#58843=CARTESIAN_POINT ( 'NONE',  ( -53.51423613279429503, -126.5000000013656063, 4.591703134518082763 ) ) ;
#58853=CARTESIAN_POINT ( 'NONE',  ( -49.85088928181150436, -149.6875000027311842, -1.666127454062680702 ) ) ;
#58858=CARTESIAN_POINT ( 'NONE',  ( -51.75738570946856498, -155.0000000000000284, 3.805975901505577408 ) ) ;
#58873=CARTESIAN_POINT ( 'NONE',  ( -57.19623071787017210, -153.3750000013656347, 4.297418129356382899 ) ) ;
#58920=CARTESIAN_POINT ( 'NONE',  ( -57.19623071787017210, -137.6250000013655779, 4.297418129356382899 ) ) ;
#58923=VERTEX_POINT ( 'NONE', #43517 ) ;
#58935=VERTEX_POINT ( 'NONE', #33256 ) ;
#58940=CARTESIAN_POINT ( 'NONE',  ( -59.29741812935640155, -142.6250000013655779, -2.196230717870135685 ) ) ;
#58968=CARTESIAN_POINT ( 'NONE',  ( -58.39396692619412477, -144.6875000013656063, 2.891590998281057701 ) ) ;
#58991=DIRECTION ( 'NONE',  ( -0.6485228581062915110, 0.000000000000000000, -0.7611951803011149931 ) ) ;
#59008=CARTESIAN_POINT ( 'NONE',  ( -50.01589407740564042, -132.6250000000000284, 0.3983568153799778022 ) ) ;
#59017=CARTESIAN_POINT ( 'NONE',  ( -52.10840900171896806, -154.1875000013656063, 3.393966926194110556 ) ) ;
#59018=DIRECTION ( 'NONE',  ( 0.000000000000000000, -1.000000000000000000, 0.000000000000000000 ) ) ;
#59019=CARTESIAN_POINT ( 'NONE',  ( -50.66154591918759564, -135.0000000000001137, 1.672849277080756147 ) ) ;
#59034=( BOUNDED_CURVE ( )  B_SPLINE_CURVE ( 2, ( #15077, #59468, #53677, #63343, #10254, #39825, #29855, #19257, #54955 ),
 .UNSPECIFIED., .F., .F. ) 
 B_SPLINE_CURVE_WITH_KNOTS ( ( 3, 2, 2, 2, 3 ),
 ( 0.02500000000000002220, 0.02916666666666669488, 0.03333333333333336757, 0.03750000000000003331, 0.04166666666666670599 ),
 .UNSPECIFIED. ) 
 CURVE ( )  GEOMETRIC_REPRESENTATION_ITEM ( )  RATIONAL_B_SPLINE_CURVE ( ( 0.9999999999999996669, 0.9238795325112870716, 1.000000000000000000, 0.9238795325112867385, 1.000000000000000000, 0.9238795325112867385, 1.000000000000000000, 0.9238795325112859613, 1.000000000000000666 ) ) 
 REPRESENTATION_ITEM ( '' )  );
#59047=CARTESIAN_POINT ( 'NONE',  ( -57.19623071787017210, -154.6250000013656063, 4.297418129356382899 ) ) ;
#59048=CARTESIAN_POINT ( 'NONE',  ( -50.55543936806279248, -147.0625000013656063, 0.3552334253322060320 ) ) ;
#59064=DIRECTION ( 'NONE',  ( 0.000000000000000000, 1.000000000000000000, 0.000000000000000000 ) ) ;
#59074=EDGE_LOOP ( 'NONE', ( #5395, #38138, #8647, #26117 ) ) ;
#59077=DIRECTION ( 'NONE',  ( 0.000000000000000000, 1.000000000000000000, 0.000000000000000000 ) ) ;
#59082=ORIENTED_EDGE ( 'NONE', *, *, #62972, .T. ) ;
#59083=CARTESIAN_POINT ( 'NONE',  ( -57.19623071787017210, -149.6250000013655779, 4.297418129356382899 ) ) ;
#59093=CARTESIAN_POINT ( 'NONE',  ( -60.14911071818854538, -146.0624999999999716, 1.666127454062681368 ) ) ;
#59097=VECTOR ( 'NONE', #48878, 1000.000000000000000 ) ;
#59102=CARTESIAN_POINT ( 'NONE',  ( -50.70258187064364108, -146.3750000013655779, 2.196230717870141014 ) ) ;
#59104=CARTESIAN_POINT ( 'NONE',  ( -52.53715891517739323, -139.5625000027311842, -4.819101127000233298 ) ) ;
#59116=CARTESIAN_POINT ( 'NONE',  ( -50.40829686548195099, -134.0000000013656063, -1.485763867205728284 ) ) ;
#59131=CARTESIAN_POINT ( 'NONE',  ( -57.19623071787017210, -139.3750000013656063, 4.297418129356382899 ) ) ;
#59164=CARTESIAN_POINT ( 'NONE',  ( -50.40829686548195099, -150.0000000013656063, -1.485763867205728284 ) ) ;
#59171=CARTESIAN_POINT ( 'NONE',  ( -50.55543936806279248, -127.3125000013655921, 0.3552334253322060320 ) ) ;
#59181=CARTESIAN_POINT ( 'NONE',  ( -54.60164318462004474, -151.5000000027312410, -4.984105922594373794 ) ) ;
#59195=( BOUNDED_CURVE ( )  B_SPLINE_CURVE ( 2, ( #52813, #14192, #12937, #43772, #42838, #47359, #32880, #3307, #62788 ),
 .UNSPECIFIED., .F., .F. ) 
 B_SPLINE_CURVE_WITH_KNOTS ( ( 3, 2, 2, 2, 3 ),
 ( 0.3083333333333336257, 0.3125000000000002776, 0.3166666666666669294, 0.3208333333333336368, 0.3250000000000002887 ),
 .UNSPECIFIED. ) 
 CURVE ( )  GEOMETRIC_REPRESENTATION_ITEM ( )  RATIONAL_B_SPLINE_CURVE ( ( 0.9999999999999948930, 0.9238795325112918455, 1.000000000000000000, 0.9238795325112867385, 1.000000000000000000, 0.9238795325112867385, 1.000000000000000000, 0.9238795325112816315, 1.000000000000005107 ) ) 
 REPRESENTATION_ITEM ( '' )  );
#59199=CARTESIAN_POINT ( 'NONE',  ( -51.75738570946856498, -155.0000000000000284, 3.805975901505577408 ) ) ;
#59204=CARTESIAN_POINT ( 'NONE',  ( -59.44456063193725015, -152.5625000013656063, -0.3552334253322034230 ) ) ;
#59224=CARTESIAN_POINT ( 'NONE',  ( -59.47495026108718008, -134.9999999999999716, -1.537000407889604459 ) ) ;
#59237=CARTESIAN_POINT ( 'NONE',  ( -51.19402409849444524, -136.5000000000000284, -3.242614290531456334 ) ) ;
#59247=CARTESIAN_POINT ( 'NONE',  ( -57.19623071787017210, -138.6250000013655779, 4.297418129356382899 ) ) ;
#59265=CARTESIAN_POINT ( 'NONE',  ( -50.70258187064364108, -141.1250000013655779, 2.196230717870141014 ) ) ;
#59290=CARTESIAN_POINT ( 'NONE',  ( -59.44456063193725015, -144.8125000013656063, -0.3552334253322034230 ) ) ;
#59325=EDGE_LOOP ( 'NONE', ( #59598, #12131, #23378, #5346 ) ) ;
#59332=CARTESIAN_POINT ( 'NONE',  ( -60.14911071818854538, -130.0625000000000284, 1.666127454062681368 ) ) ;
#59342=CARTESIAN_POINT ( 'NONE',  ( -58.39396692619412477, -153.4375000013656063, 2.891590998281057701 ) ) ;
#59366=CARTESIAN_POINT ( 'NONE',  ( -51.60603307380591787, -154.1875000013656063, -2.891590998281053704 ) ) ;
#59367=CARTESIAN_POINT ( 'NONE',  ( -50.55543936806279248, -142.0625000013656063, 0.3552334253322060320 ) ) ;
#59402=CARTESIAN_POINT ( 'NONE',  ( -54.64476657466781973, -146.0625000013656063, -4.444560631937228834 ) ) ;
#59414=CARTESIAN_POINT ( 'NONE',  ( -50.01589407740564042, -141.6250000000000284, 0.3983568153799778022 ) ) ;
#59419=ORIENTED_EDGE ( 'NONE', *, *, #36683, .F. ) ;
#59424=VERTEX_POINT ( 'NONE', #62833 ) ;
#59425=CARTESIAN_POINT ( 'NONE',  ( -53.51423613279429503, -147.5000000013656063, 4.591703134518083651 ) ) ;
#59427=CARTESIAN_POINT ( 'NONE',  ( -57.46284108482265651, -134.0625000027312126, 4.819101127000239515 ) ) ;
#59441=CARTESIAN_POINT ( 'NONE',  ( -56.48576386720575471, -131.7500000013656063, -4.591703134518078322 ) ) ;
#59454=CARTESIAN_POINT ( 'NONE',  ( -50.55543936806279248, -136.0625000013656063, 0.3552334253322060320 ) ) ;
#59462=CARTESIAN_POINT ( 'NONE',  ( -59.29741812935640155, -130.8750000013656063, -2.196230717870135685 ) ) ;
#59468=CARTESIAN_POINT ( 'NONE',  ( -59.81910112700025905, -153.3125000027312410, -2.462841084822619209 ) ) ;
#59487=ORIENTED_EDGE ( 'NONE', *, *, #56583, .T. ) ;
#59488=CARTESIAN_POINT ( 'NONE',  ( -52.80376928212989185, -150.8750000013656063, -4.297418129356378458 ) ) ;
#59495=CARTESIAN_POINT ( 'NONE',  ( -50.70258187064364108, -128.3750000013656631, 2.196230717870141014 ) ) ;
#59502=VERTEX_POINT ( 'NONE', #57383 ) ;
#59506=CARTESIAN_POINT ( 'NONE',  ( -49.85088928181150436, -144.6875000027312126, -1.666127454062680702 ) ) ;
#59528=CARTESIAN_POINT ( 'NONE',  ( -57.19623071787017210, -148.3750000013656063, 4.297418129356382899 ) ) ;
#59546=CARTESIAN_POINT ( 'NONE',  ( -58.24261429053147765, -151.3750000027312126, -3.805975901505573855 ) ) ;
#59555=COLOUR_RGB ( '',0.8941176470588234615, 0.8941176470588234615, 0.8941176470588234615 ) ;
#59576=CARTESIAN_POINT ( 'NONE',  ( -52.10840900171896806, -138.4375000013656063, 3.393966926194110556 ) ) ;
#59594=CARTESIAN_POINT ( 'NONE',  ( -57.19623071787017210, -141.3750000013656063, 4.297418129356382899 ) ) ;
#59598=ORIENTED_EDGE ( 'NONE', *, *, #5172, .F. ) ;
#59621=CARTESIAN_POINT ( 'NONE',  ( -53.51423613279429503, -145.5000000013656063, 4.591703134518082763 ) ) ;
#59631=VERTEX_POINT ( 'NONE', #29660 ) ;
#59653=CARTESIAN_POINT ( 'NONE',  ( -50.01589407740564042, -137.6250000000000284, 0.3983568153799778022 ) ) ;
#59655=EDGE_LOOP ( 'NONE', ( #44299, #16141, #1764, #17642, #655, #26754 ) ) ;
#59656=CARTESIAN_POINT ( 'NONE',  ( -58.24261429053147765, -141.2500000000000284, -3.805975901505573855 ) ) ;
#59661=CARTESIAN_POINT ( 'NONE',  ( -52.53715891517739323, -131.4375000000000284, -4.819101127000233298 ) ) ;
#59668=CARTESIAN_POINT ( 'NONE',  ( -53.51423613279429503, -153.2500000013655779, 4.591703134518082763 ) ) ;
#59673=CARTESIAN_POINT ( 'NONE',  ( -60.14911071818854538, -146.0624999999999716, 1.666127454062681146 ) ) ;
#59687=ORIENTED_EDGE ( 'NONE', *, *, #54250, .F. ) ;
#59694=CARTESIAN_POINT ( 'NONE',  ( -59.59170313451811296, -126.5000000013656063, 1.485763867205729394 ) ) ;
#59695=CARTESIAN_POINT ( 'NONE',  ( -55.35523342533222291, -143.3125000013656063, 4.444560631937231499 ) ) ;
#59704=VERTEX_POINT ( 'NONE', #14239 ) ;
#59736=AXIS2_PLACEMENT_3D ( 'NONE', #43096, #53697, #63363 ) ;
#59737=CARTESIAN_POINT ( 'NONE',  ( -59.98410592259440222, -143.1250000000000284, -0.3983568153799752487 ) ) ;
#59747=CARTESIAN_POINT ( 'NONE',  ( -59.29741812935640155, -147.8750000013655779, -2.196230717870135685 ) ) ;
#59749=CARTESIAN_POINT ( 'NONE',  ( -59.98410592259440222, -133.2500000027312126, -0.3983568153799752487 ) ) ;
#59761=CARTESIAN_POINT ( 'NONE',  ( -51.60603307380591787, -129.9375000013656063, -2.891590998281053704 ) ) ;
#59769=DIRECTION ( 'NONE',  ( 0.000000000000000000, 1.000000000000000000, 0.000000000000000000 ) ) ;
#59777=CARTESIAN_POINT ( 'NONE',  ( -50.70258187064364108, -137.1250000013655779, 2.196230717870141014 ) ) ;
#59789=CARTESIAN_POINT ( 'NONE',  ( -57.89159099828107458, -131.9375000013656063, -3.393966926194107447 ) ) ;
#59815=CARTESIAN_POINT ( 'NONE',  ( -59.44456063193725015, -149.5625000013656063, -0.3552334253322034230 ) ) ;
#59823=CARTESIAN_POINT ( 'NONE',  ( -59.59170313451811296, -124.7500000013655921, 1.485763867205729394 ) ) ;
#59826=CARTESIAN_POINT ( 'NONE',  ( -51.75738570946856498, -136.8750000027312126, 3.805975901505576964 ) ) ;
#59831=CYLINDRICAL_SURFACE ( 'NONE', #30343, 5.000000000000000000 ) ;
#59833=CARTESIAN_POINT ( 'NONE',  ( -60.14911071818854538, -145.1875000027312126, 1.666127454062681368 ) ) ;
#59850=CARTESIAN_POINT ( 'NONE',  ( -56.48576386720575471, -147.7500000013655779, -4.591703134518078322 ) ) ;
#59856=CARTESIAN_POINT ( 'NONE',  ( -55.00000000000001421, -135.0000000000000284, 8.082903768654762899 ) ) ;
#59886=CARTESIAN_POINT ( 'NONE',  ( -52.53715891517739323, -147.5625000027312126, -4.819101127000233298 ) ) ;
#59902=CARTESIAN_POINT ( 'NONE',  ( -57.89159099828107458, -136.9375000013655779, -3.393966926194107447 ) ) ;
#59909=CARTESIAN_POINT ( 'NONE',  ( -52.00883452924551165, -135.0000000000000284, -3.319254266616502136 ) ) ;
#59920=CARTESIAN_POINT ( 'NONE',  ( -50.55543936806279248, -140.0625000013656063, 0.3552334253322060320 ) ) ;
#59944=CARTESIAN_POINT ( 'NONE',  ( -59.44456063193725015, -142.8125000013656063, -0.3552334253322034230 ) ) ;
#59978=EDGE_LOOP ( 'NONE', ( #56012, #46446, #56426, #36947, #3443, #60764, #24571, #46096, #22082, #877, #39700, #22767, #32978, #53279, #19826, #5948, #52995, #25979, #44734, #49779, #14827, #51222, #58636, #8623, #10286, #34808, #45073, #41525, #17620, #19293, #22750, #45320, #24601, #11923, #41320, #46597, #35205, #58425, #30743, #61256, #40489, #25132 ) ) ;
#59979=CARTESIAN_POINT ( 'NONE',  ( -50.18089887299976937, -141.6875000000000000, 2.462841084822427362 ) ) ;
#59984=CARTESIAN_POINT ( 'NONE',  ( -57.46284108482265651, -129.9375000000000000, 4.819101127000239515 ) ) ;
#59991=CARTESIAN_POINT ( 'NONE',  ( -52.80376928212989185, -151.8750000013655779, -4.297418129356379346 ) ) ;
#60016=CARTESIAN_POINT ( 'NONE',  ( -57.19623071787017210, -126.3750000013656489, 4.297418129356382899 ) ) ;
#60017=CARTESIAN_POINT ( 'NONE',  ( -50.70258187064364108, -144.1250000013656063, 2.196230717870141014 ) ) ;
#60038=EDGE_LOOP ( 'NONE', ( #57803, #32032, #18179, #3061 ) ) ;
#60048=CARTESIAN_POINT ( 'NONE',  ( -55.00000000000001421, -135.0000000000000284, -8.082903768654752241 ) ) ;
#60052=CARTESIAN_POINT ( 'NONE',  ( -59.98410592259440222, -140.1250000000000284, -0.3983568153799752487 ) ) ;
#60063=CARTESIAN_POINT ( 'NONE',  ( -55.35523342533222291, -147.5625000013656063, 4.444560631937231499 ) ) ;
#60065=CARTESIAN_POINT ( 'NONE',  ( -55.39835681537999790, -136.0000000027312126, 4.984105922594378235 ) ) ;
#60081=CARTESIAN_POINT ( 'NONE',  ( -59.44456063193725015, -127.5625000013655921, -0.3552334253322034230 ) ) ;
#60083=CARTESIAN_POINT ( 'NONE',  ( -59.81910112700026616, -146.3125000027311842, -2.462841084822510851 ) ) ;
#60086=ORIENTED_EDGE ( 'NONE', *, *, #21609, .T. ) ;
#60096=CARTESIAN_POINT ( 'NONE',  ( -52.80376928212989185, -136.8750000013656063, -4.297418129356379346 ) ) ;
#60106=CARTESIAN_POINT ( 'NONE',  ( -57.19623071787017210, -130.6250000013656347, 4.297418129356382899 ) ) ;
#60131=CARTESIAN_POINT ( 'NONE',  ( -59.29741812935640155, -150.6250000013656063, -2.196230717870135685 ) ) ;
#60138=CARTESIAN_POINT ( 'NONE',  ( -59.44456063193725015, -124.8125000013655921, -0.3552334253322034230 ) ) ;
#60150=CARTESIAN_POINT ( 'NONE',  ( -55.39835681537999790, -147.0000000027312126, 4.984105922594378235 ) ) ;
#60169=CARTESIAN_POINT ( 'NONE',  ( -59.81910112700027327, -138.1875000000000000, -2.462841084822392279 ) ) ;
#60170=CARTESIAN_POINT ( 'NONE',  ( -55.35523342533222291, -148.3125000013656063, 4.444560631937231499 ) ) ;
#60172=CYLINDRICAL_SURFACE ( 'NONE', #1444, 5.000000000000000000 ) ;
#60208=CARTESIAN_POINT ( 'NONE',  ( -59.98410592259440222, -141.2500000027312126, -0.3983568153799752487 ) ) ;
#60215=CARTESIAN_POINT ( 'NONE',  ( -50.40829686548195099, -136.2500000013656063, -1.485763867205728284 ) ) ;
#60223=CARTESIAN_POINT ( 'NONE',  ( -55.22501343921605610, -134.9999999999999432, -4.462558208288625039 ) ) ;
#60225=ORIENTED_EDGE ( 'NONE', *, *, #23961, .F. ) ;
#60246=CARTESIAN_POINT ( 'NONE',  ( -50.18089887299977647, -147.6875000000000284, 2.462841084822530835 ) ) ;
#60264=CARTESIAN_POINT ( 'NONE',  ( -50.70258187064364108, -140.3750000013656063, 2.196230717870141014 ) ) ;
#60296=CARTESIAN_POINT ( 'NONE',  ( -58.80597590150559739, -149.1250000027312126, 3.242614290531460330 ) ) ;
#60301=CARTESIAN_POINT ( 'NONE',  ( -58.24261429053147765, -131.2500000000000284, -3.805975901505573855 ) ) ;
#60309=EDGE_CURVE ( 'NONE', #61181, #61334, #30681, .T. ) ;
#60311=CARTESIAN_POINT ( 'NONE',  ( -58.39396692619412477, -154.4375000013656063, 2.891590998281057701 ) ) ;
#60312=CARTESIAN_POINT ( 'NONE',  ( -48.00000000000002132, -135.0000000000000284, -4.041451884327376121 ) ) ;
#60336=CARTESIAN_POINT ( 'NONE',  ( -54.64476657466781973, -124.8125000013655921, -4.444560631937228834 ) ) ;
#60337=CARTESIAN_POINT ( 'NONE',  ( -50.40829686548195099, -141.0000000013655779, -1.485763867205728284 ) ) ;
#60378=CARTESIAN_POINT ( 'NONE',  ( -54.60164318462004474, -141.3750000000000284, -4.984105922594373794 ) ) ;
#60387=CARTESIAN_POINT ( 'NONE',  ( -59.44456063193725015, -140.8125000013656063, -0.3552334253322034230 ) ) ;
#60389=CARTESIAN_POINT ( 'NONE',  ( -50.01589407740564042, -132.7500000027312126, 0.3983568153799778022 ) ) ;
#60404=CARTESIAN_POINT ( 'NONE',  ( -50.40829686548195099, -128.0000000013656063, -1.485763867205728284 ) ) ;
#60417=CARTESIAN_POINT ( 'NONE',  ( -59.59170313451811296, -137.5000000013656063, 1.485763867205729394 ) ) ;
#60427=CARTESIAN_POINT ( 'NONE',  ( -50.40829686548195099, -131.2500000013656347, -1.485763867205728284 ) ) ;
#60459=CARTESIAN_POINT ( 'NONE',  ( -51.19402409849444524, -153.5000000000000284, -3.242614290531456334 ) ) ;
#60466=CARTESIAN_POINT ( 'NONE',  ( -57.46284108482265651, -149.9375000000000284, 4.819101127000238627 ) ) ;
#60468=CARTESIAN_POINT ( 'NONE',  ( -59.59170313451810586, -152.7500000013655779, 1.485763867205729394 ) ) ;
#60470=CARTESIAN_POINT ( 'NONE',  ( -58.80597590150559739, -145.1250000027312126, 3.242614290531460330 ) ) ;
#60487=CARTESIAN_POINT ( 'NONE',  ( -52.10840900171896806, -149.1875000013656063, 3.393966926194110556 ) ) ;
#60535=CARTESIAN_POINT ( 'NONE',  ( -50.40829686548195099, -133.2500000013656347, -1.485763867205728284 ) ) ;
#60536=ADVANCED_FACE ( 'NONE', ( #18534 ), #57472, .T. ) ;
#60548=CARTESIAN_POINT ( 'NONE',  ( -54.60164318462004474, -149.3750000000000284, -4.984105922594373794 ) ) ;
#60551=ADVANCED_FACE ( 'NONE', ( #14325 ), #9190, .F. ) ;
#60569=( GEOMETRIC_REPRESENTATION_CONTEXT ( 3 ) GLOBAL_UNCERTAINTY_ASSIGNED_CONTEXT ( ( #53236 ) ) GLOBAL_UNIT_ASSIGNED_CONTEXT ( ( #32118, #60780, #62041 ) ) REPRESENTATION_CONTEXT ( 'NONE', 'WORKASPACE' ) );
#60579=CARTESIAN_POINT ( 'NONE',  ( -58.39396692619412477, -141.6875000013656063, 2.891590998281057701 ) ) ;
#60601=CARTESIAN_POINT ( 'NONE',  ( -52.80376928212989185, -135.1250000013656063, -4.297418129356378458 ) ) ;
#60614=CARTESIAN_POINT ( 'NONE',  ( -59.29741812935640155, -147.8750000013656063, -2.196230717870135685 ) ) ;
#60624=CARTESIAN_POINT ( 'NONE',  ( -55.39835681537999790, -127.8750000000000142, 4.984105922594378235 ) ) ;
#60632=CARTESIAN_POINT ( 'NONE',  ( -59.59170313451811296, -150.5000000013655779, 1.485763867205729394 ) ) ;
#60640=CARTESIAN_POINT ( 'NONE',  ( -51.19402409849444524, -152.6250000027312126, -3.242614290531456334 ) ) ;
#60643=CARTESIAN_POINT ( 'NONE',  ( -57.46284108482265651, -146.9375000000000000, 4.819101127000238627 ) ) ;
#60644=DIRECTION ( 'NONE',  ( -0.8660254037844387076, 0.000000000000000000, -0.4999999999999997780 ) ) ;
#60655=CARTESIAN_POINT ( 'NONE',  ( -58.39396692619412477, -151.6875000013656063, 2.891590998281057701 ) ) ;
#60656=CARTESIAN_POINT ( 'NONE',  ( -50.40829686548195099, -144.0000000013656063, -1.485763867205728284 ) ) ;
#60669=CARTESIAN_POINT ( 'NONE',  ( -59.98410592259440222, -136.1250000000000284, -0.3983568153799752487 ) ) ;
#60671=ADVANCED_FACE ( 'NONE', ( #11324 ), #21630, .F. ) ;
#60696=CARTESIAN_POINT ( 'NONE',  ( -58.24261429053147765, -141.2500000000000284, -3.805975901505573855 ) ) ;
#60702=CARTESIAN_POINT ( 'NONE',  ( -58.24261429053147765, -137.3750000027312126, -3.805975901505573855 ) ) ;
#60705=CARTESIAN_POINT ( 'NONE',  ( -50.70258187064364108, -141.3750000013656063, 2.196230717870141014 ) ) ;
#60708=CARTESIAN_POINT ( 'NONE',  ( -56.66612745406270335, -134.4375000027312410, -5.149110718188516067 ) ) ;
#60718=CARTESIAN_POINT ( 'NONE',  ( -57.89159099828107458, -128.6875000013656063, -3.393966926194107447 ) ) ;
#60725=CARTESIAN_POINT ( 'NONE',  ( -58.24261429053147765, -139.2500000000000000, -3.805975901505573855 ) ) ;
#60732=CARTESIAN_POINT ( 'NONE',  ( -59.59170313451811296, -135.5000000013656063, 1.485763867205729394 ) ) ;
#60743=CARTESIAN_POINT ( 'NONE',  ( -57.19623071787017210, -131.6250000013655779, 4.297418129356382899 ) ) ;
#60760=AXIS2_PLACEMENT_3D ( 'NONE', #8150, #28068, #3329 ) ;
#60764=ORIENTED_EDGE ( 'NONE', *, *, #8923, .T. ) ;
#60770=CARTESIAN_POINT ( 'NONE',  ( -56.48576386720575471, -138.7500000013655779, -4.591703134518078322 ) ) ;
#60776=CARTESIAN_POINT ( 'NONE',  ( -56.66612745406270335, -154.3125000000000284, -5.149110718188516067 ) ) ;
#60780=( NAMED_UNIT ( * ) PLANE_ANGLE_UNIT ( ) SI_UNIT ( $, .RADIAN. ) );
#60787=CARTESIAN_POINT ( 'NONE',  ( -58.24261429053147765, -147.3750000027312126, -3.805975901505573855 ) ) ;
#60804=CARTESIAN_POINT ( 'NONE',  ( -57.89159099828107458, -150.6875000013656063, -3.393966926194107447 ) ) ;
#60821=CARTESIAN_POINT ( 'NONE',  ( -55.39835681537999790, -152.0000000027312410, 4.984105922594378235 ) ) ;
#60847=CARTESIAN_POINT ( 'NONE',  ( -58.39396692619412477, -134.6875000013656063, 2.891590998281057701 ) ) ;
#60865=CARTESIAN_POINT ( 'NONE',  ( -54.60164318462004474, -148.5000000027312126, -4.984105922594373794 ) ) ;
#60891=CARTESIAN_POINT ( 'NONE',  ( -57.89159099828107458, -138.9375000013656063, -3.393966926194107447 ) ) ;
#60896=( BOUNDED_CURVE ( )  B_SPLINE_CURVE ( 2, ( #31320, #35521, #16853, #11070, #60296, #25229, #6572, #49986, #50955 ),
 .UNSPECIFIED., .F., .F. ) 
 B_SPLINE_CURVE_WITH_KNOTS ( ( 3, 2, 2, 2, 3 ),
 ( 0.1583333333333334925, 0.1625000000000001721, 0.1666666666666668239, 0.1708333333333335036, 0.1750000000000001554 ),
 .UNSPECIFIED. ) 
 CURVE ( )  GEOMETRIC_REPRESENTATION_ITEM ( )  RATIONAL_B_SPLINE_CURVE ( ( 0.9999999999999970024, 0.9238795325112897361, 1.000000000000000000, 0.9238795325112867385, 1.000000000000000000, 0.9238795325112867385, 1.000000000000000000, 0.9238795325112837409, 1.000000000000003109 ) ) 
 REPRESENTATION_ITEM ( '' )  );
#60912=ADVANCED_BREP_SHAPE_REPRESENTATION ( '', ( #28816, #43054 ), #60569 ) ;
#60920=CARTESIAN_POINT ( 'NONE',  ( -51.75738570946856498, -138.7500000000000000, 3.805975901505576964 ) ) ;
#60926=CARTESIAN_POINT ( 'NONE',  ( -56.48576386720575471, -147.0000000013655779, -4.591703134518078322 ) ) ;
#60939=CARTESIAN_POINT ( 'NONE',  ( -50.18089887299979068, -125.6875000000000711, 2.462841084822635640 ) ) ;
#60947=CARTESIAN_POINT ( 'NONE',  ( -58.39396692619412477, -149.4375000013656063, 2.891590998281057701 ) ) ;
#60972=CARTESIAN_POINT ( 'NONE',  ( -52.10840900171896806, -150.4375000013656063, 3.393966926194110556 ) ) ;
#60976=CARTESIAN_POINT ( 'NONE',  ( -50.01589407740564042, -153.7500000027312410, 0.3983568153799778022 ) ) ;
#61008=CARTESIAN_POINT ( 'NONE',  ( -51.19402409849444524, -139.5000000000000284, -3.242614290531456334 ) ) ;
#61012=EDGE_CURVE ( 'NONE', #11458, #9785, #59034, .T. ) ;
#61019=CARTESIAN_POINT ( 'NONE',  ( -59.59170313451810586, -142.7500000013655779, 1.485763867205729394 ) ) ;
#61021=CARTESIAN_POINT ( 'NONE',  ( -58.24261429053147765, -130.3750000027312126, -3.805975901505573855 ) ) ;
#61031=( BOUNDED_CURVE ( )  B_SPLINE_CURVE ( 2, ( #20407, #21048, #59653, #50632, #55141, #10427, #1446, #54503, #40654 ),
 .UNSPECIFIED., .F., .F. ) 
 B_SPLINE_CURVE_WITH_KNOTS ( ( 3, 2, 2, 2, 3 ),
 ( 0.5750000000000005107, 0.5791666666666672736, 0.5833333333333339255, 0.5875000000000004663, 0.5916666666666671182 ),
 .UNSPECIFIED. ) 
 CURVE ( )  GEOMETRIC_REPRESENTATION_ITEM ( )  RATIONAL_B_SPLINE_CURVE ( ( 0.9999999999999898970, 0.9238795325112968415, 1.000000000000000000, 0.9238795325112867385, 1.000000000000000000, 0.9238795325112867385, 1.000000000000000000, 0.9238795325112786339, 1.000000000000008216 ) ) 
 REPRESENTATION_ITEM ( '' )  );
#61037=CARTESIAN_POINT ( 'NONE',  ( -59.59170313451811296, -124.5000000013656063, 1.485763867205729394 ) ) ;
#61044=CARTESIAN_POINT ( 'NONE',  ( -49.85088928181150436, -146.5625000000000000, -1.666127454062680480 ) ) ;
#61053=CARTESIAN_POINT ( 'NONE',  ( -52.10840900171896806, -132.1875000013656063, 3.393966926194110556 ) ) ;
#61064=CARTESIAN_POINT ( 'NONE',  ( -59.59170313451811296, -129.7500000013656063, 1.485763867205729394 ) ) ;
#61088=CARTESIAN_POINT ( 'NONE',  ( -59.44456063193725015, -140.5625000013656063, -0.3552334253322034230 ) ) ;
#61093=CARTESIAN_POINT ( 'NONE',  ( -55.39835681537999790, -152.8750000000000284, 4.984105922594378235 ) ) ;
#61103=CARTESIAN_POINT ( 'NONE',  ( -54.60164318462004474, -141.5000000027312126, -4.984105922594373794 ) ) ;
#61111=CARTESIAN_POINT ( 'NONE',  ( -59.44456063193725015, -142.5625000013656063, -0.3552334253322034230 ) ) ;
#61125=CARTESIAN_POINT ( 'NONE',  ( -51.60603307380591787, -143.9375000013656063, -2.891590998281053704 ) ) ;
#61147=FACE_OUTER_BOUND ( 'NONE', #3874, .T. ) ;
#61170=CARTESIAN_POINT ( 'NONE',  ( -50.55543936806279248, -134.3125000013656063, 0.3552334253322060320 ) ) ;
#61177=CARTESIAN_POINT ( 'NONE',  ( -58.24261429053147765, -155.0000000000000284, -3.805975901505573411 ) ) ;
#61181=VERTEX_POINT ( 'NONE', #26962 ) ;
#61186=CARTESIAN_POINT ( 'NONE',  ( -58.24261429053147765, -147.3750000027312126, -3.805975901505573855 ) ) ;
#61210=CARTESIAN_POINT ( 'NONE',  ( -59.29741812935640155, -139.8750000013655779, -2.196230717870135685 ) ) ;
#61242=CARTESIAN_POINT ( 'NONE',  ( -59.29741812935640155, -145.8750000013655779, -2.196230717870135685 ) ) ;
#61249=DIRECTION ( 'NONE',  ( -0.6485228581062915110, 0.000000000000000000, -0.7611951803011149931 ) ) ;
#61256=ORIENTED_EDGE ( 'NONE', *, *, #12660, .T. ) ;
#61260=CARTESIAN_POINT ( 'NONE',  ( -59.59170313451811296, -147.5000000013656063, 1.485763867205729394 ) ) ;
#61261=CARTESIAN_POINT ( 'NONE',  ( -59.81910112700025905, -150.3125000027311842, -2.462841084822570359 ) ) ;
#61264=EDGE_LOOP ( 'NONE', ( #60225, #34537, #25062, #59687 ) ) ;
#61282=ORIENTED_EDGE ( 'NONE', *, *, #46485, .T. ) ;
#61286=CARTESIAN_POINT ( 'NONE',  ( -53.51423613279429503, -153.5000000013656063, 4.591703134518082763 ) ) ;
#61290=CARTESIAN_POINT ( 'NONE',  ( -58.24261429053147765, -153.3750000027312126, -3.805975901505573855 ) ) ;
#61327=CARTESIAN_POINT ( 'NONE',  ( -49.85088928181150436, -138.5625000000000284, -1.666127454062680702 ) ) ;
#61334=VERTEX_POINT ( 'NONE', #37552 ) ;
#61336=CARTESIAN_POINT ( 'NONE',  ( -57.89159099828107458, -143.9375000013656063, -3.393966926194107447 ) ) ;
#61338=CARTESIAN_POINT ( 'NONE',  ( -50.01589407740564042, -131.7500000027312126, 0.3983568153799778022 ) ) ;
#61350=CARTESIAN_POINT ( 'NONE',  ( -55.35523342533222291, -126.3125000013655921, 4.444560631937231499 ) ) ;
#61364=CARTESIAN_POINT ( 'NONE',  ( -50.55543936806279248, -135.0625000013656063, 0.3552334253322060320 ) ) ;
#61374=CARTESIAN_POINT ( 'NONE',  ( -52.10840900171896806, -127.4375000013656063, 3.393966926194110556 ) ) ;
#61398=CARTESIAN_POINT ( 'NONE',  ( -54.64476657466781973, -154.0625000013656347, -4.444560631937228834 ) ) ;
#61399=EDGE_CURVE ( 'NONE', #40939, #49453, #17904, .T. ) ;
#61403=CARTESIAN_POINT ( 'NONE',  ( -51.60603307380591787, -138.9375000013656063, -2.891590998281053704 ) ) ;
#61408=ORIENTED_EDGE ( 'NONE', *, *, #27956, .T. ) ;
#61409=CARTESIAN_POINT ( 'NONE',  ( -54.60164318462004474, -151.3750000000000284, -4.984105922594373794 ) ) ;
#61419=CARTESIAN_POINT ( 'NONE',  ( -59.44456063193725015, -153.8125000013656347, -0.3552334253322034230 ) ) ;
#61420=CARTESIAN_POINT ( 'NONE',  ( -50.01589407740564042, -143.7500000027312126, 0.3983568153799778022 ) ) ;
#61428=CARTESIAN_POINT ( 'NONE',  ( -50.40829686548195099, -137.0000000013655779, -1.485763867205728284 ) ) ;
#61442=CARTESIAN_POINT ( 'NONE',  ( -59.44456063193725015, -147.5625000013656063, -0.3552334253322034230 ) ) ;
#61488=CARTESIAN_POINT ( 'NONE',  ( -50.40829686548195099, -132.2500000013656063, -1.485763867205728284 ) ) ;
#61505=CARTESIAN_POINT ( 'NONE',  ( -60.14911071818854538, -147.1875000027312410, 1.666127454062681146 ) ) ;
#61530=CARTESIAN_POINT ( 'NONE',  ( -58.39396692619412477, -138.6875000013656347, 2.891590998281057701 ) ) ;
#61546=VECTOR ( 'NONE', #18819, 1000.000000000000000 ) ;
#61550=CARTESIAN_POINT ( 'NONE',  ( -56.37266686252615955, -135.0000000000000284, -4.242180533871957593 ) ) ;
#61552=CARTESIAN_POINT ( 'NONE',  ( -51.75738570946856498, -145.8750000027312126, 3.805975901505576964 ) ) ;
#61560=CARTESIAN_POINT ( 'NONE',  ( -59.59170313451811296, -148.7500000013655779, 1.485763867205729394 ) ) ;
#61572=CARTESIAN_POINT ( 'NONE',  ( -58.80597590150559739, -125.0000000000000284, 3.242614290531460330 ) ) ;
#61579=CARTESIAN_POINT ( 'NONE',  ( -52.80376928212989185, -149.8750000013655779, -4.297418129356379346 ) ) ;
#61594=FACE_OUTER_BOUND ( 'NONE', #17252, .T. ) ;
#61604=CARTESIAN_POINT ( 'NONE',  ( -57.19623071787017210, -153.6250000013655779, 4.297418129356382899 ) ) ;
#61611=CARTESIAN_POINT ( 'NONE',  ( -58.24261429053147765, -135.3750000027312410, -3.805975901505573855 ) ) ;
#61616=CARTESIAN_POINT ( 'NONE',  ( -55.39835681537999790, -152.8750000000000284, 4.984105922594378235 ) ) ;
#61643=CARTESIAN_POINT ( 'NONE',  ( -50.01589407740564042, -137.6250000000000284, 0.3983568153799778022 ) ) ;
#61652=CARTESIAN_POINT ( 'NONE',  ( -51.60603307380591787, -137.1875000013656063, -2.891590998281053704 ) ) ;
#61654=CARTESIAN_POINT ( 'NONE',  ( -58.24261429053147765, -132.3750000027312126, -3.805975901505573855 ) ) ;
#61660=CARTESIAN_POINT ( 'NONE',  ( -58.24261429053147765, -151.3750000027312126, -3.805975901505573855 ) ) ;
#61668=CARTESIAN_POINT ( 'NONE',  ( -50.70258187064364108, -126.1250000013656205, 2.196230717870141014 ) ) ;
#61679=CARTESIAN_POINT ( 'NONE',  ( -51.60603307380591787, -134.9375000013656063, -2.891590998281053704 ) ) ;
#61691=CARTESIAN_POINT ( 'NONE',  ( -51.60603307380591787, -126.1875000013656063, -2.891590998281053704 ) ) ;
#61714=CARTESIAN_POINT ( 'NONE',  ( -58.24261429053147765, -149.2500000000000284, -3.805975901505573855 ) ) ;
#61718=CARTESIAN_POINT ( 'NONE',  ( -59.44456063193725015, -139.5625000013656063, -0.3552334253322034230 ) ) ;
#61724=VECTOR ( 'NONE', #48540, 1000.000000000000000 ) ;
#61725=CARTESIAN_POINT ( 'NONE',  ( -57.46284108482265651, -150.9375000000000284, 4.819101127000239515 ) ) ;
#61733=CARTESIAN_POINT ( 'NONE',  ( -50.55543936806279248, -153.3125000013656063, 0.3552334253322060320 ) ) ;
#61734=CARTESIAN_POINT ( 'NONE',  ( -59.98410592259440222, -141.2500000027312126, -0.3983568153799752487 ) ) ;
#61744=CARTESIAN_POINT ( 'NONE',  ( -50.40829686548195099, -138.0000000013656063, -1.485763867205728284 ) ) ;
#61746=FACE_OUTER_BOUND ( 'NONE', #54278, .T. ) ;
#61758=CARTESIAN_POINT ( 'NONE',  ( -54.64476657466781973, -145.8125000013656063, -4.444560631937228834 ) ) ;
#61762=DIRECTION ( 'NONE',  ( 0.000000000000000000, 1.000000000000000000, 0.000000000000000000 ) ) ;
#61772=CARTESIAN_POINT ( 'NONE',  ( -60.14911071818854538, -149.0625000000000000, 1.666127454062681146 ) ) ;
#61799=CARTESIAN_POINT ( 'NONE',  ( -52.10840900171896806, -131.4375000013656063, 3.393966926194110556 ) ) ;
#61819=CARTESIAN_POINT ( 'NONE',  ( -50.18089887299978358, -148.8125000027311842, 2.462841084822545934 ) ) ;
#61849=CARTESIAN_POINT ( 'NONE',  ( -57.89159099828107458, -137.9375000013656063, -3.393966926194107447 ) ) ;
#61880=CARTESIAN_POINT ( 'NONE',  ( -52.80376928212989185, -142.1250000013656063, -4.297418129356379346 ) ) ;
#61898=CARTESIAN_POINT ( 'NONE',  ( -53.51423613279429503, -150.2500000013656063, 4.591703134518082763 ) ) ;
#61922=CARTESIAN_POINT ( 'NONE',  ( -57.19623071787017210, -150.6250000013656063, 4.297418129356382899 ) ) ;
#61958=CARTESIAN_POINT ( 'NONE',  ( -50.01589407740564042, -138.6250000000000284, 0.3983568153799778022 ) ) ;
#61968=CARTESIAN_POINT ( 'NONE',  ( -59.44456063193725015, -138.8125000013656063, -0.3552334253322034230 ) ) ;
#61970=CARTESIAN_POINT ( 'NONE',  ( -57.46284108482265651, -132.0625000027312126, 4.819101127000239515 ) ) ;
#61991=VECTOR ( 'NONE', #26704, 1000.000000000000000 ) ;
#61994=CARTESIAN_POINT ( 'NONE',  ( -53.51423613279429503, -132.2500000013656063, 4.591703134518082763 ) ) ;
#62004=CARTESIAN_POINT ( 'NONE',  ( -59.44456063193725015, -129.8125000013656063, -0.3552334253322034230 ) ) ;
#62017=LINE ( 'NONE', #32418, #44234 ) ;
#62025=ORIENTED_EDGE ( 'NONE', *, *, #29916, .T. ) ;
#62026=CARTESIAN_POINT ( 'NONE',  ( -51.60603307380591787, -154.1875000013656063, -2.891590998281053704 ) ) ;
#62030=CARTESIAN_POINT ( 'NONE',  ( -50.55543936806279248, -139.0625000013656063, 0.3552334253322060320 ) ) ;
#62036=CARTESIAN_POINT ( 'NONE',  ( -49.85088928181150436, -150.5625000000000284, -1.666127454062680702 ) ) ;
#62041=( NAMED_UNIT ( * ) SI_UNIT ( $, .STERADIAN. ) SOLID_ANGLE_UNIT ( ) );
#62046=CARTESIAN_POINT ( 'NONE',  ( -59.44456063193725015, -151.8125000013656063, -0.3552334253322034230 ) ) ;
#62047=CARTESIAN_POINT ( 'NONE',  ( -51.75738570946856498, -141.8750000027312126, 3.805975901505576964 ) ) ;
#62048=DIRECTION ( 'NONE',  ( -0.6485228581062915110, 0.000000000000000000, -0.7611951803011149931 ) ) ;
#62056=CARTESIAN_POINT ( 'NONE',  ( -50.40829686548195099, -139.0000000013655779, -1.485763867205728284 ) ) ;
#62071=CARTESIAN_POINT ( 'NONE',  ( -51.60603307380591787, -144.9375000013656063, -2.891590998281053704 ) ) ;
#62113=CARTESIAN_POINT ( 'NONE',  ( -50.70258187064364108, -129.3750000013656347, 2.196230717870141014 ) ) ;
#62120=ORIENTED_EDGE ( 'NONE', *, *, #19972, .F. ) ;
#62140=DIRECTION ( 'NONE',  ( -0.6485228581062915110, 0.000000000000000000, -0.7611951803011149931 ) ) ;
#62156=CARTESIAN_POINT ( 'NONE',  ( -58.39396692619412477, -134.6875000013656063, 2.891590998281057701 ) ) ;
#62174=EDGE_CURVE ( 'NONE', #39445, #59704, #22987, .T. ) ;
#62189=CARTESIAN_POINT ( 'NONE',  ( -50.70258187064364108, -144.3750000013656063, 2.196230717870141014 ) ) ;
#62200=CARTESIAN_POINT ( 'NONE',  ( 0.000000000000000000, 0.000000000000000000, 0.000000000000000000 ) ) ;
#62211=CARTESIAN_POINT ( 'NONE',  ( -55.35523342533222291, -143.3125000013656063, 4.444560631937231499 ) ) ;
#62214=ORIENTED_EDGE ( 'NONE', *, *, #7348, .F. ) ;
#62224=CARTESIAN_POINT ( 'NONE',  ( -55.00000000000002132, -155.0000000000000284, 1.734723475976807094E-15 ) ) ;
#62225=CARTESIAN_POINT ( 'NONE',  ( -51.75738570946856498, -139.7500000000000000, 3.805975901505576964 ) ) ;
#62236=CARTESIAN_POINT ( 'NONE',  ( -54.64476657466781973, -148.0625000013656063, -4.444560631937228834 ) ) ;
#62261=ORIENTED_EDGE ( 'NONE', *, *, #53840, .T. ) ;
#62271=CYLINDRICAL_SURFACE ( 'NONE', #43961, 5.000000000000000000 ) ;
#62277=CARTESIAN_POINT ( 'NONE',  ( -51.19402409849444524, -136.5000000000000284, -3.242614290531456334 ) ) ;
#62285=CARTESIAN_POINT ( 'NONE',  ( -58.39396692619412477, -139.6875000013656347, 2.891590998281057701 ) ) ;
#62287=CARTESIAN_POINT ( 'NONE',  ( -53.33387254593733928, -128.9375000027312126, 5.149110718188519620 ) ) ;
#62298=CARTESIAN_POINT ( 'NONE',  ( -52.10840900171896806, -125.1875000013656063, 3.393966926194110556 ) ) ;
#62308=CARTESIAN_POINT ( 'NONE',  ( -50.55543936806279248, -128.0625000013656063, 0.3552334253322060320 ) ) ;
#62319=CARTESIAN_POINT ( 'NONE',  ( -55.35523342533222291, -129.5625000013656063, 4.444560631937231499 ) ) ;
#62344=FACE_OUTER_BOUND ( 'NONE', #6701, .T. ) ;
#62348=CARTESIAN_POINT ( 'NONE',  ( -50.70258187064364108, -135.1250000013656063, 2.196230717870141014 ) ) ;
#62351=ORIENTED_EDGE ( 'NONE', *, *, #52293, .F. ) ;
#62352=CARTESIAN_POINT ( 'NONE',  ( -59.98410592259440222, -151.1250000000000284, -0.3983568153799752487 ) ) ;
#62362=CARTESIAN_POINT ( 'NONE',  ( -55.35523342533222291, -149.5625000013656063, 4.444560631937231499 ) ) ;
#62363=CARTESIAN_POINT ( 'NONE',  ( -59.81910112700025905, -142.3125000027312410, -2.462841084822630311 ) ) ;
#62372=CARTESIAN_POINT ( 'NONE',  ( -52.10840900171896806, -135.1875000013656063, 3.393966926194110556 ) ) ;
#62383=CARTESIAN_POINT ( 'NONE',  ( -58.59997141384986463, -154.8437500006828031, 3.067102644406258793 ) ) ;
#62388=CARTESIAN_POINT ( 'NONE',  ( -52.80376928212989185, -142.8750000013656063, -4.297418129356379346 ) ) ;
#62434=CARTESIAN_POINT ( 'NONE',  ( -59.59170313451811296, -131.7500000013656063, 1.485763867205729394 ) ) ;
#62439=DIRECTION ( 'NONE',  ( 0.000000000000000000, 1.000000000000000000, 0.000000000000000000 ) ) ;
#62464=CARTESIAN_POINT ( 'NONE',  ( -51.75738570946856498, -141.7500000000000284, 3.805975901505576964 ) ) ;
#62478=CARTESIAN_POINT ( 'NONE',  ( -56.48576386720575471, -138.0000000013656063, -4.591703134518078322 ) ) ;
#62487=EDGE_LOOP ( 'NONE', ( #53862, #40020, #20289, #39437 ) ) ;
#62501=CARTESIAN_POINT ( 'NONE',  ( -51.75738570946856498, -151.8750000027312126, 3.805975901505576964 ) ) ;
#62505=AXIS2_PLACEMENT_3D ( 'NONE', #13390, #38450, #63227 ) ;
#62511=CARTESIAN_POINT ( 'NONE',  ( -59.29741812935640155, -141.8750000013655779, -2.196230717870135685 ) ) ;
#62524=ORIENTED_EDGE ( 'NONE', *, *, #37079, .T. ) ;
#62528=CARTESIAN_POINT ( 'NONE',  ( -50.70258187064364108, -143.1250000013656063, 2.196230717870141014 ) ) ;
#62541=CARTESIAN_POINT ( 'NONE',  ( -51.75738570946856498, -141.7500000000000284, 3.805975901505576964 ) ) ;
#62543=CARTESIAN_POINT ( 'NONE',  ( -51.75738570946856498, -140.8750000027312126, 3.805975901505576964 ) ) ;
#62545=CARTESIAN_POINT ( 'NONE',  ( -51.19402409849444524, -146.5000000000000284, -3.242614290531456334 ) ) ;
#62549=CARTESIAN_POINT ( 'NONE',  ( -59.81910112700026616, -144.1875000000000000, -2.462841084822481541 ) ) ;
#62556=CARTESIAN_POINT ( 'NONE',  ( -51.60603307380591787, -149.1875000013656063, -2.891590998281053704 ) ) ;
#62563=CARTESIAN_POINT ( 'NONE',  ( -53.33387254593723981, -147.8125000000000284, 5.149110718188528502 ) ) ;
#62568=CARTESIAN_POINT ( 'NONE',  ( -58.24261429053147765, -153.2500000000000284, -3.805975901505573855 ) ) ;
#62594=CARTESIAN_POINT ( 'NONE',  ( -55.39835681537999790, -133.8750000000000284, 4.984105922594378235 ) ) ;
#62601=CARTESIAN_POINT ( 'NONE',  ( -59.29741812935640155, -137.8750000013655779, -2.196230717870135685 ) ) ;
#62603=CARTESIAN_POINT ( 'NONE',  ( -58.24261429053147765, -128.3750000027312126, -3.805975901505573855 ) ) ;
#62615=CARTESIAN_POINT ( 'NONE',  ( -53.33387254593731086, -153.8125000000000284, 5.149110718188520508 ) ) ;
#62620=EDGE_CURVE ( 'NONE', #32199, #32996, #25412, .T. ) ;
#62629=CARTESIAN_POINT ( 'NONE',  ( -59.44456063193725015, -128.5625000013656063, -0.3552334253322034230 ) ) ;
#62641=CARTESIAN_POINT ( 'NONE',  ( -57.19623071787017210, -125.6250000013656205, 4.297418129356382899 ) ) ;
#62662=CARTESIAN_POINT ( 'NONE',  ( -50.40829686548195099, -150.2500000013656063, -1.485763867205728284 ) ) ;
#62666=CARTESIAN_POINT ( 'NONE',  ( -52.80376928212989185, -135.8750000013655779, -4.297418129356378458 ) ) ;
#62671=CARTESIAN_POINT ( 'NONE',  ( -50.01589407740564042, -147.6250000000000284, 0.3983568153799778022 ) ) ;
#62680=CARTESIAN_POINT ( 'NONE',  ( -54.64476657466781973, -152.0625000013656063, -4.444560631937228834 ) ) ;
#62681=CARTESIAN_POINT ( 'NONE',  ( -53.33387254593733928, -136.9375000027312126, 5.149110718188519620 ) ) ;
#62688=CARTESIAN_POINT ( 'NONE',  ( -56.66612745406293783, -139.4375000027311842, -5.149110718188535607 ) ) ;
#62689=CARTESIAN_POINT ( 'NONE',  ( -59.59170313451811296, -137.5000000013656063, 1.485763867205729394 ) ) ;
#62694=VERTEX_POINT ( 'NONE', #15497 ) ;
#62703=CARTESIAN_POINT ( 'NONE',  ( -53.51423613279429503, -143.2500000013656063, 4.591703134518082763 ) ) ;
#62737=CARTESIAN_POINT ( 'NONE',  ( -58.39396692619412477, -152.4375000013656063, 2.891590998281057701 ) ) ;
#62745=CARTESIAN_POINT ( 'NONE',  ( -51.60603307380591787, -133.1875000013656063, -2.891590998281053704 ) ) ;
#62767=CARTESIAN_POINT ( 'NONE',  ( -51.75738570946856498, -155.0000000000000284, 3.805975901505577408 ) ) ;
#62771=CARTESIAN_POINT ( 'NONE',  ( -58.39396692619412477, -153.4375000013656063, 2.891590998281057701 ) ) ;
#62773=PLANE ( 'NONE',  #23750 ) ;
#62783=CARTESIAN_POINT ( 'NONE',  ( -60.14911071818854538, -145.1875000027312410, 1.666127454062681146 ) ) ;
#62786=CARTESIAN_POINT ( 'NONE',  ( -53.51423613279429503, -135.5000000013656063, 4.591703134518082763 ) ) ;
#62788=CARTESIAN_POINT ( 'NONE',  ( -58.24261429053147765, -145.2500000000000284, -3.805975901505573855 ) ) ;
#62793=ORIENTED_EDGE ( 'NONE', *, *, #14237, .F. ) ;
#62805=CARTESIAN_POINT ( 'NONE',  ( -53.33387254593719717, -143.9375000027312126, 5.149110718188530278 ) ) ;
#62817=EDGE_CURVE ( 'NONE', #32525, #1423, #16128, .T. ) ;
#62818=CARTESIAN_POINT ( 'NONE',  ( -51.60603307380591787, -143.1875000013656063, -2.891590998281053704 ) ) ;
#62828=CARTESIAN_POINT ( 'NONE',  ( -59.98410592259440222, -143.2500000027312126, -0.3983568153799752487 ) ) ;
#62833=CARTESIAN_POINT ( 'NONE',  ( -58.24261429053147765, -147.2500000000000284, -3.805975901505573855 ) ) ;
#62836=CARTESIAN_POINT ( 'NONE',  ( -53.51423613279429503, -144.2500000013656063, 4.591703134518082763 ) ) ;
#62847=CARTESIAN_POINT ( 'NONE',  ( -59.81910112700026616, -142.1875000000000284, -2.462841084822451343 ) ) ;
#62861=CARTESIAN_POINT ( 'NONE',  ( -50.70258187064364108, -148.3750000013656063, 2.196230717870141014 ) ) ;
#62872=CARTESIAN_POINT ( 'NONE',  ( -58.24261429053147765, -141.2500000000000284, -3.805975901505573855 ) ) ;
#62897=CARTESIAN_POINT ( 'NONE',  ( -57.46284108482265651, -134.9375000000000000, 4.819101127000239515 ) ) ;
#62907=CARTESIAN_POINT ( 'NONE',  ( -50.55543936806279248, -137.3125000013656063, 0.3552334253322060320 ) ) ;
#62910=CARTESIAN_POINT ( 'NONE',  ( -49.85088928181150436, -126.6875000027312410, -1.666127454062680702 ) ) ;
#62933=CARTESIAN_POINT ( 'NONE',  ( -50.70258187064364108, -131.1250000013655779, 2.196230717870141014 ) ) ;
#62934=CARTESIAN_POINT ( 'NONE',  ( -57.19623071787016499, -146.3750000013655779, 4.297418129356382899 ) ) ;
#62958=ORIENTED_EDGE ( 'NONE', *, *, #58343, .F. ) ;
#62961=CARTESIAN_POINT ( 'NONE',  ( 0.000000000000000000, -155.0000000000000284, 0.000000000000000000 ) ) ;
#62969=CARTESIAN_POINT ( 'NONE',  ( -50.70258187064364108, -152.3750000013656063, 2.196230717870141014 ) ) ;
#62972=EDGE_CURVE ( 'NONE', #44963, #28712, #14694, .T. ) ;
#62980=CARTESIAN_POINT ( 'NONE',  ( -51.75738570946856498, -145.7500000000000284, 3.805975901505576964 ) ) ;
#62994=CARTESIAN_POINT ( 'NONE',  ( -52.10840900171896806, -148.4375000013656063, 3.393966926194110556 ) ) ;
#62995=CARTESIAN_POINT ( 'NONE',  ( -50.01589407740564042, -136.7500000027312126, 0.3983568153799778022 ) ) ;
#62999=FACE_OUTER_BOUND ( 'NONE', #33146, .T. ) ;
#63005=CARTESIAN_POINT ( 'NONE',  ( -50.55543936806279248, -132.0625000013656063, 0.3552334253322060320 ) ) ;
#63021=CARTESIAN_POINT ( 'NONE',  ( -51.60603307380591787, -141.9375000013656063, -2.891590998281053704 ) ) ;
#63025=CARTESIAN_POINT ( 'NONE',  ( -50.18089887299977647, -144.6874999999999716, 2.462841084822486426 ) ) ;
#63048=DIRECTION ( 'NONE',  ( 0.000000000000000000, 1.000000000000000000, 0.000000000000000000 ) ) ;
#63051=CARTESIAN_POINT ( 'NONE',  ( -59.44456063193725015, -152.5625000013656063, -0.3552334253322034230 ) ) ;
#63057=CARTESIAN_POINT ( 'NONE',  ( -52.10840900171896806, -128.4375000013656063, 3.393966926194110556 ) ) ;
#63068=CARTESIAN_POINT ( 'NONE',  ( -52.53715891517739323, -149.5625000027312126, -4.819101127000233298 ) ) ;
#63072=EDGE_CURVE ( 'NONE', #38301, #2645, #25802, .T. ) ;
#63083=LINE ( 'NONE', #38608, #2822 ) ;
#63091=DIRECTION ( 'NONE',  ( 0.000000000000000000, -1.000000000000000000, 0.000000000000000000 ) ) ;
#63103=CARTESIAN_POINT ( 'NONE',  ( -51.60603307380591787, -137.1875000013656063, -2.891590998281053704 ) ) ;
#63125=CARTESIAN_POINT ( 'NONE',  ( -58.39396692619412477, -154.4375000013656063, 2.891590998281057701 ) ) ;
#63133=CARTESIAN_POINT ( 'NONE',  ( -57.19623071787017210, -143.6250000013655779, 4.297418129356382899 ) ) ;
#63149=CARTESIAN_POINT ( 'NONE',  ( -58.39396692619412477, -144.4375000013656063, 2.891590998281057701 ) ) ;
#63167=CARTESIAN_POINT ( 'NONE',  ( -58.24261429053147765, -144.2500000000000284, -3.805975901505573855 ) ) ;
#63174=CARTESIAN_POINT ( 'NONE',  ( -56.48576386720575471, -148.0000000013655779, -4.591703134518078322 ) ) ;
#63185=CARTESIAN_POINT ( 'NONE',  ( -60.14911071818854538, -141.0625000000000284, 1.666127454062681146 ) ) ;
#63211=CARTESIAN_POINT ( 'NONE',  ( -54.60164318462004474, -135.3750000000000284, -4.984105922594373794 ) ) ;
#63220=CARTESIAN_POINT ( 'NONE',  ( -60.14911071818854538, -127.1875000027312126, 1.666127454062681368 ) ) ;
#63222=CARTESIAN_POINT ( 'NONE',  ( -55.39835672516371545, -134.9999999999999716, 4.984105929804953483 ) ) ;
#63225=CARTESIAN_POINT ( 'NONE',  ( -53.33387254593719717, -145.8125000000000000, 5.149110718188530278 ) ) ;
#63227=DIRECTION ( 'NONE',  ( -0.8660254037844385966, 0.000000000000000000, -0.5000000000000000000 ) ) ;
#63242=EDGE_CURVE ( 'NONE', #52748, #19205, #54360, .T. ) ;
#63245=CARTESIAN_POINT ( 'NONE',  ( -54.64476657466781973, -130.8125000013656063, -4.444560631937228834 ) ) ;
#63246=CARTESIAN_POINT ( 'NONE',  ( -55.35523342533222291, -145.3125000013656063, 4.444560631937231499 ) ) ;
#63253=ORIENTED_EDGE ( 'NONE', *, *, #48092, .F. ) ;
#63278=ORIENTED_EDGE ( 'NONE', *, *, #15430, .F. ) ;
#63279=CARTESIAN_POINT ( 'NONE',  ( -53.51423613279429503, -152.5000000013655779, 4.591703134518082763 ) ) ;
#63284=CARTESIAN_POINT ( 'NONE',  ( -56.48576386720575471, -135.7500000013656063, -4.591703134518078322 ) ) ;
#63288=CARTESIAN_POINT ( 'NONE',  ( -57.46284108482265651, -145.9375000000000284, 4.819101127000239515 ) ) ;
#63296=CARTESIAN_POINT ( 'NONE',  ( -52.10840900171896806, -149.4375000013656063, 3.393966926194110556 ) ) ;
#63297=CARTESIAN_POINT ( 'NONE',  ( -55.39835681537999790, -138.0000000027312126, 4.984105922594378235 ) ) ;
#63307=CARTESIAN_POINT ( 'NONE',  ( -53.51423613279429503, -132.2500000013656063, 4.591703134518082763 ) ) ;
#63324=VECTOR ( 'NONE', #19951, 1000.000000000000000 ) ;
#63325=CARTESIAN_POINT ( 'NONE',  ( -53.51423613279429503, -140.2500000013656063, 4.591703134518082763 ) ) ;
#63331=( BOUNDED_CURVE ( )  B_SPLINE_CURVE ( 2, ( #18976, #14152, #19613, #19292, #38910, #4505, #39225, #8704, #24131 ),
 .UNSPECIFIED., .F., .F. ) 
 B_SPLINE_CURVE_WITH_KNOTS ( ( 3, 2, 2, 2, 3 ),
 ( 0.3916666666666669960, 0.3958333333333336479, 0.4000000000000003553, 0.4041666666666670071, 0.4083333333333336590 ),
 .UNSPECIFIED. ) 
 CURVE ( )  GEOMETRIC_REPRESENTATION_ITEM ( )  RATIONAL_B_SPLINE_CURVE ( ( 0.9999999999999938938, 0.9238795325112928447, 1.000000000000000000, 0.9238795325112867385, 1.000000000000000000, 0.9238795325112867385, 1.000000000000000000, 0.9238795325112806323, 1.000000000000005995 ) ) 
 REPRESENTATION_ITEM ( '' )  );
#63332=CARTESIAN_POINT ( 'NONE',  ( -51.19402409849444524, -144.5000000000000284, -3.242614290531456334 ) ) ;
#63343=CARTESIAN_POINT ( 'NONE',  ( -60.14911071818854538, -153.1875000027312126, 1.666127454062681146 ) ) ;
#63363=DIRECTION ( 'NONE',  ( -0.6485228581062915110, 0.000000000000000000, -0.7611951803011149931 ) ) ;
#63367=CARTESIAN_POINT ( 'NONE',  ( -54.60164318462004474, -149.5000000027312126, -4.984105922594373794 ) ) ;
#63370=CARTESIAN_POINT ( 'NONE',  ( -50.70258187064364108, -127.3750000013656205, 2.196230717870141014 ) ) ;
#63381=CARTESIAN_POINT ( 'NONE',  ( -57.46284108482265651, -151.0625000027312410, 4.819101127000239515 ) ) ;
#63398=CARTESIAN_POINT ( 'NONE',  ( -58.24261429053147765, -137.2500000000000000, -3.805975901505573855 ) ) ;
#63399=CARTESIAN_POINT ( 'NONE',  ( -51.60603307380591787, -152.9375000013656063, -2.891590998281053704 ) ) ;
#63416=AXIS2_PLACEMENT_3D ( 'NONE', #14508, #34776, #44095 ) ;
#63422=PLANE ( 'NONE',  #63416 ) ;
#63428=LINE ( 'NONE', #29624, #6252 ) ;
#63447=CARTESIAN_POINT ( 'NONE',  ( -54.64476657466781973, -138.0625000013656063, -4.444560631937228834 ) ) ;
#63465=CARTESIAN_POINT ( 'NONE',  ( -54.64476657466781973, -143.8125000013656063, -4.444560631937228834 ) ) ;
#63485=CARTESIAN_POINT ( 'NONE',  ( -51.19402409849444524, -154.5000000000000284, -3.242614290531456334 ) ) ;
#63488=CARTESIAN_POINT ( 'NONE',  ( -52.10840900171896806, -144.4375000013656063, 3.393966926194110556 ) ) ;
#63493=CARTESIAN_POINT ( 'NONE',  ( -59.81910112700026616, -148.1875000000000284, -2.462841084822525506 ) ) ;
#63510=DIRECTION ( 'NONE',  ( 0.000000000000000000, 1.000000000000000000, 0.000000000000000000 ) ) ;
#63527=CARTESIAN_POINT ( 'NONE',  ( -50.01589407740564042, -133.6250000000000284, 0.3983568153799778022 ) ) ;
#63536=CARTESIAN_POINT ( 'NONE',  ( -59.98410592259440222, -126.2500000027311984, -0.3983568153799752487 ) ) ;
#63538=CARTESIAN_POINT ( 'NONE',  ( -50.45012647926553484, -135.0000000000000284, 0.5292737942098199033 ) ) ;
#63544=VECTOR ( 'NONE', #11546, 1000.000000000000000 ) ;
#63545=FACE_OUTER_BOUND ( 'NONE', #4776, .T. ) ;
#63563=CARTESIAN_POINT ( 'NONE',  ( -59.59170313451811296, -129.5000000013656347, 1.485763867205729394 ) ) ;
#63564=CARTESIAN_POINT ( 'NONE',  ( -54.64476657466781973, -147.8125000013656063, -4.444560631937228834 ) ) ;
#63597=CARTESIAN_POINT ( 'NONE',  ( -51.60603307380591787, -151.1875000013656063, -2.891590998281053704 ) ) ;
#63600=ORIENTED_EDGE ( 'NONE', *, *, #11941, .F. ) ;
#63607=CARTESIAN_POINT ( 'NONE',  ( -51.19402409849444524, -146.5000000000000284, -3.242614290531456334 ) ) ;
#63615=CARTESIAN_POINT ( 'NONE',  ( -54.64476657466781973, -148.0625000013656063, -4.444560631937228834 ) ) ;
#63616=CARTESIAN_POINT ( 'NONE',  ( -57.46284108482265651, -140.0625000027312126, 4.819101127000239515 ) ) ;
#63628=CARTESIAN_POINT ( 'NONE',  ( -51.19402409849444524, -153.5000000000000284, -3.242614290531456334 ) ) ;
#63629=CARTESIAN_POINT ( 'NONE',  ( -56.48576386720575471, -134.7500000013656063, -4.591703134518078322 ) ) ;
#63646=CARTESIAN_POINT ( 'NONE',  ( -50.70258187064364108, -142.1250000013656063, 2.196230717870141014 ) ) ;
#63650=CARTESIAN_POINT ( 'NONE',  ( -49.85088928181150436, -144.5625000000000284, -1.666127454062680480 ) ) ;
#63692=COLOUR_RGB('Light Blue',0.38,0.62,0.78);
#63693=FILL_AREA_STYLE_COLOUR('',#63692);
#63694=FILL_AREA_STYLE('',(#63693));
#63695=SURFACE_STYLE_FILL_AREA(#63694);
#63696=SURFACE_SIDE_STYLE('',(#63695));
#63697=SURFACE_STYLE_USAGE(.BOTH.,#63696);
#63698=PRESENTATION_STYLE_ASSIGNMENT((#63697));
ENDSEC;
END-ISO-10303-21;
